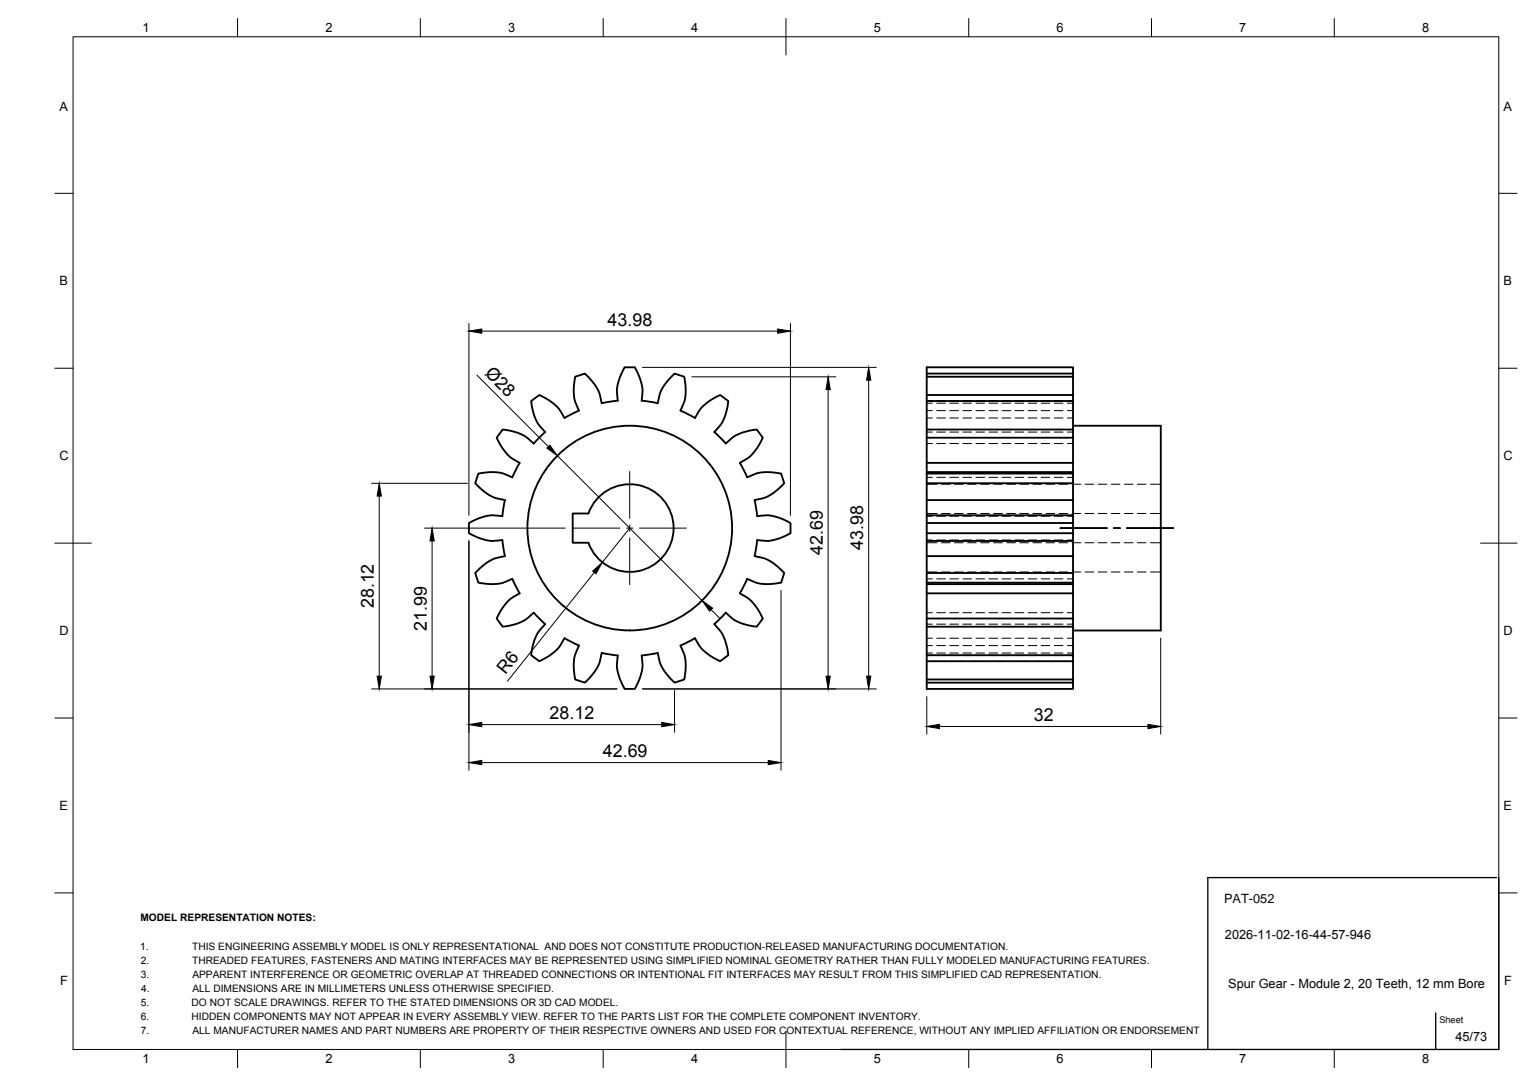
ISO-10303-21;
HEADER;
/* Generated by software containing ST-Developer
 * from STEP Tools, Inc. (www.steptools.com) 
 */

FILE_DESCRIPTION(
/* description */ ('Hand-crank gear train demonstrator'),
/* implementation_level */ '2;1');

FILE_NAME(
/* name */ 'Spur Gear - Module 2, 20 Teeth, 12 mm Bore.step',
/* time_stamp */ '2026-10-28T03:22:13-07:00',
/* author */ (''),
/* organization */ (''),
/* preprocessor_version */ 'ST-DEVELOPER v20.2',
/* originating_system */ 'Autodesk Translation Framework v15.17.0.0',
/* authorisation */ '');

FILE_SCHEMA (('AUTOMOTIVE_DESIGN { 1 0 10303 214 3 1 1 }'));
ENDSEC;

DATA;
#10=MECHANICAL_DESIGN_GEOMETRIC_PRESENTATION_REPRESENTATION('',(#1253),#62758);
#11=(
BOUNDED_SURFACE()
B_SPLINE_SURFACE(5,1,((#29730,#29731),(#29732,#29733),(#29734,#29735),(#29736,
#29737),(#29738,#29739),(#29740,#29741),(#29742,#29743),(#29744,#29745),
(#29746,#29747),(#29748,#29749),(#29750,#29751),(#29752,#29753),(#29754,
#29755),(#29756,#29757),(#29758,#29759),(#29760,#29761),(#29762,#29763),
(#29764,#29765),(#29766,#29767),(#29768,#29769),(#29770,#29771),(#29772,
#29773),(#29774,#29775),(#29776,#29777),(#29778,#29779),(#29780,#29781),
(#29782,#29783),(#29784,#29785),(#29786,#29787),(#29788,#29789),(#29790,
#29791),(#29792,#29793),(#29794,#29795),(#29796,#29797),(#29798,#29799),
(#29800,#29801),(#29802,#29803),(#29804,#29805),(#29806,#29807),(#29808,
#29809),(#29810,#29811),(#29812,#29813),(#29814,#29815),(#29816,#29817),
(#29818,#29819),(#29820,#29821),(#29822,#29823),(#29824,#29825),(#29826,
#29827),(#29828,#29829),(#29830,#29831),(#29832,#29833),(#29834,#29835),
(#29836,#29837),(#29838,#29839),(#29840,#29841),(#29842,#29843),(#29844,
#29845),(#29846,#29847),(#29848,#29849),(#29850,#29851),(#29852,#29853),
(#29854,#29855),(#29856,#29857),(#29858,#29859),(#29860,#29861),(#29862,
#29863),(#29864,#29865),(#29866,#29867),(#29868,#29869)),.UNSPECIFIED.,
 .F.,.F.,.F.)
B_SPLINE_SURFACE_WITH_KNOTS((6,1,1,1,1,1,1,1,1,1,1,1,1,1,1,1,1,1,1,1,1,
1,1,1,1,1,1,1,1,1,1,1,1,1,1,1,1,1,1,1,1,1,1,1,1,1,1,1,1,1,1,1,1,1,1,1,1,
1,1,1,1,1,1,1,1,6),(2,2),(-1.,-0.984615384615383,-0.969230769230768,-0.953846153846152,
-0.938461538461537,-0.923076923076922,-0.907692307692306,-0.892307692307691,
-0.876923076923076,-0.86153846153846,-0.846153846153845,-0.83076923076923,
-0.815384615384614,-0.799999999999999,-0.784615384615384,-0.769230769230768,
-0.753846153846153,-0.738461538461538,-0.723076923076922,-0.707692307692307,
-0.692307692307692,-0.676923076923076,-0.661538461538461,-0.646153846153846,
-0.63076923076923,-0.615384615384615,-0.6,-0.584615384615384,-0.569230769230769,
-0.553846153846154,-0.538461538461538,-0.523076923076923,-0.507692307692308,
-0.492307692307692,-0.476923076923077,-0.461538461538462,-0.446153846153846,
-0.430769230769231,-0.415384615384615,-0.4,-0.384615384615385,-0.369230769230769,
-0.353846153846154,-0.338461538461538,-0.323076923076923,-0.307692307692308,
-0.292307692307692,-0.276923076923077,-0.261538461538462,-0.246153846153846,
-0.230769230769231,-0.215384615384615,-0.2,-0.184615384615385,-0.169230769230769,
-0.153846153846154,-0.138461538461538,-0.123076923076923,-0.107692307692308,
-0.0923076923076923,-0.0769230769230769,-0.0615384615384615,-0.0461538461538462,
-0.0307692307692308,-0.0153846153846154,0.),(-1.,1.),.UNSPECIFIED.)
GEOMETRIC_REPRESENTATION_ITEM()
RATIONAL_B_SPLINE_SURFACE(((1.,1.),(1.,1.),(1.,1.),(1.,1.),(1.,1.),(1.,
1.),(1.,1.),(1.,1.),(1.,1.),(1.,1.),(1.,1.),(1.,1.),(1.,1.),(1.,1.),(1.,
1.),(1.,1.),(1.,1.),(1.,1.),(1.,1.),(1.,1.),(1.,1.),(1.,1.),(1.,1.),(1.,
1.),(1.,1.),(1.,1.),(1.,1.),(1.,1.),(1.,1.),(1.,1.),(1.,1.),(1.,1.),(1.,
1.),(1.,1.),(1.,1.),(1.,1.),(1.,1.),(1.,1.),(1.,1.),(1.,1.),(1.,1.),(1.,
1.),(1.,1.),(1.,1.),(1.,1.),(1.,1.),(1.,1.),(1.,1.),(1.,1.),(1.,1.),(1.,
1.),(1.,1.),(1.,1.),(1.,1.),(1.,1.),(1.,1.),(1.,1.),(1.,1.),(1.,1.),(1.,
1.),(1.,1.),(1.,1.),(1.,1.),(1.,1.),(1.,1.),(1.,1.),(1.,1.),(1.,1.),(1.,
1.),(1.,1.)))
REPRESENTATION_ITEM('')
SURFACE()
);
#12=(
BOUNDED_SURFACE()
B_SPLINE_SURFACE(5,1,((#29948,#29949),(#29950,#29951),(#29952,#29953),(#29954,
#29955),(#29956,#29957),(#29958,#29959),(#29960,#29961),(#29962,#29963),
(#29964,#29965),(#29966,#29967),(#29968,#29969),(#29970,#29971),(#29972,
#29973),(#29974,#29975),(#29976,#29977),(#29978,#29979),(#29980,#29981),
(#29982,#29983),(#29984,#29985),(#29986,#29987),(#29988,#29989),(#29990,
#29991),(#29992,#29993),(#29994,#29995),(#29996,#29997),(#29998,#29999),
(#30000,#30001),(#30002,#30003),(#30004,#30005),(#30006,#30007),(#30008,
#30009),(#30010,#30011),(#30012,#30013),(#30014,#30015),(#30016,#30017),
(#30018,#30019),(#30020,#30021),(#30022,#30023),(#30024,#30025),(#30026,
#30027),(#30028,#30029),(#30030,#30031),(#30032,#30033),(#30034,#30035),
(#30036,#30037),(#30038,#30039),(#30040,#30041),(#30042,#30043),(#30044,
#30045),(#30046,#30047),(#30048,#30049),(#30050,#30051),(#30052,#30053),
(#30054,#30055),(#30056,#30057),(#30058,#30059),(#30060,#30061),(#30062,
#30063),(#30064,#30065),(#30066,#30067),(#30068,#30069),(#30070,#30071),
(#30072,#30073),(#30074,#30075),(#30076,#30077),(#30078,#30079),(#30080,
#30081),(#30082,#30083),(#30084,#30085),(#30086,#30087)),.UNSPECIFIED.,
 .F.,.F.,.F.)
B_SPLINE_SURFACE_WITH_KNOTS((6,1,1,1,1,1,1,1,1,1,1,1,1,1,1,1,1,1,1,1,1,
1,1,1,1,1,1,1,1,1,1,1,1,1,1,1,1,1,1,1,1,1,1,1,1,1,1,1,1,1,1,1,1,1,1,1,1,
1,1,1,1,1,1,1,1,6),(2,2),(-1.,-0.984615384615383,-0.969230769230768,-0.953846153846152,
-0.938461538461537,-0.923076923076922,-0.907692307692306,-0.892307692307691,
-0.876923076923076,-0.86153846153846,-0.846153846153845,-0.83076923076923,
-0.815384615384614,-0.799999999999999,-0.784615384615384,-0.769230769230768,
-0.753846153846153,-0.738461538461538,-0.723076923076922,-0.707692307692307,
-0.692307692307692,-0.676923076923076,-0.661538461538461,-0.646153846153846,
-0.63076923076923,-0.615384615384615,-0.6,-0.584615384615384,-0.569230769230769,
-0.553846153846154,-0.538461538461538,-0.523076923076923,-0.507692307692308,
-0.492307692307692,-0.476923076923077,-0.461538461538462,-0.446153846153846,
-0.430769230769231,-0.415384615384615,-0.4,-0.384615384615385,-0.369230769230769,
-0.353846153846154,-0.338461538461538,-0.323076923076923,-0.307692307692308,
-0.292307692307692,-0.276923076923077,-0.261538461538462,-0.246153846153846,
-0.230769230769231,-0.215384615384615,-0.2,-0.184615384615385,-0.169230769230769,
-0.153846153846154,-0.138461538461538,-0.123076923076923,-0.107692307692308,
-0.0923076923076923,-0.0769230769230769,-0.0615384615384615,-0.0461538461538462,
-0.0307692307692308,-0.0153846153846154,0.),(-1.,1.),.UNSPECIFIED.)
GEOMETRIC_REPRESENTATION_ITEM()
RATIONAL_B_SPLINE_SURFACE(((1.,1.),(1.,1.),(1.,1.),(1.,1.),(1.,1.),(1.,
1.),(1.,1.),(1.,1.),(1.,1.),(1.,1.),(1.,1.),(1.,1.),(1.,1.),(1.,1.),(1.,
1.),(1.,1.),(1.,1.),(1.,1.),(1.,1.),(1.,1.),(1.,1.),(1.,1.),(1.,1.),(1.,
1.),(1.,1.),(1.,1.),(1.,1.),(1.,1.),(1.,1.),(1.,1.),(1.,1.),(1.,1.),(1.,
1.),(1.,1.),(1.,1.),(1.,1.),(1.,1.),(1.,1.),(1.,1.),(1.,1.),(1.,1.),(1.,
1.),(1.,1.),(1.,1.),(1.,1.),(1.,1.),(1.,1.),(1.,1.),(1.,1.),(1.,1.),(1.,
1.),(1.,1.),(1.,1.),(1.,1.),(1.,1.),(1.,1.),(1.,1.),(1.,1.),(1.,1.),(1.,
1.),(1.,1.),(1.,1.),(1.,1.),(1.,1.),(1.,1.),(1.,1.),(1.,1.),(1.,1.),(1.,
1.),(1.,1.)))
REPRESENTATION_ITEM('')
SURFACE()
);
#13=(
BOUNDED_SURFACE()
B_SPLINE_SURFACE(5,1,((#30164,#30165),(#30166,#30167),(#30168,#30169),(#30170,
#30171),(#30172,#30173),(#30174,#30175),(#30176,#30177),(#30178,#30179),
(#30180,#30181),(#30182,#30183),(#30184,#30185),(#30186,#30187),(#30188,
#30189),(#30190,#30191),(#30192,#30193),(#30194,#30195),(#30196,#30197),
(#30198,#30199),(#30200,#30201),(#30202,#30203),(#30204,#30205),(#30206,
#30207),(#30208,#30209),(#30210,#30211),(#30212,#30213),(#30214,#30215),
(#30216,#30217),(#30218,#30219),(#30220,#30221),(#30222,#30223),(#30224,
#30225),(#30226,#30227),(#30228,#30229),(#30230,#30231),(#30232,#30233),
(#30234,#30235),(#30236,#30237),(#30238,#30239),(#30240,#30241),(#30242,
#30243),(#30244,#30245),(#30246,#30247),(#30248,#30249),(#30250,#30251),
(#30252,#30253),(#30254,#30255),(#30256,#30257),(#30258,#30259),(#30260,
#30261),(#30262,#30263),(#30264,#30265),(#30266,#30267),(#30268,#30269),
(#30270,#30271),(#30272,#30273),(#30274,#30275),(#30276,#30277),(#30278,
#30279),(#30280,#30281),(#30282,#30283),(#30284,#30285),(#30286,#30287),
(#30288,#30289),(#30290,#30291),(#30292,#30293),(#30294,#30295),(#30296,
#30297),(#30298,#30299),(#30300,#30301),(#30302,#30303)),.UNSPECIFIED.,
 .F.,.F.,.F.)
B_SPLINE_SURFACE_WITH_KNOTS((6,1,1,1,1,1,1,1,1,1,1,1,1,1,1,1,1,1,1,1,1,
1,1,1,1,1,1,1,1,1,1,1,1,1,1,1,1,1,1,1,1,1,1,1,1,1,1,1,1,1,1,1,1,1,1,1,1,
1,1,1,1,1,1,1,1,6),(2,2),(-1.,-0.984615384615383,-0.969230769230768,-0.953846153846152,
-0.938461538461537,-0.923076923076922,-0.907692307692306,-0.892307692307691,
-0.876923076923076,-0.86153846153846,-0.846153846153845,-0.83076923076923,
-0.815384615384614,-0.799999999999999,-0.784615384615384,-0.769230769230768,
-0.753846153846153,-0.738461538461538,-0.723076923076922,-0.707692307692307,
-0.692307692307692,-0.676923076923076,-0.661538461538461,-0.646153846153846,
-0.63076923076923,-0.615384615384615,-0.6,-0.584615384615384,-0.569230769230769,
-0.553846153846154,-0.538461538461538,-0.523076923076923,-0.507692307692308,
-0.492307692307692,-0.476923076923077,-0.461538461538462,-0.446153846153846,
-0.430769230769231,-0.415384615384615,-0.4,-0.384615384615385,-0.369230769230769,
-0.353846153846154,-0.338461538461538,-0.323076923076923,-0.307692307692308,
-0.292307692307692,-0.276923076923077,-0.261538461538462,-0.246153846153846,
-0.230769230769231,-0.215384615384615,-0.2,-0.184615384615385,-0.169230769230769,
-0.153846153846154,-0.138461538461538,-0.123076923076923,-0.107692307692308,
-0.0923076923076923,-0.0769230769230769,-0.0615384615384615,-0.0461538461538462,
-0.0307692307692308,-0.0153846153846154,0.),(-1.,1.),.UNSPECIFIED.)
GEOMETRIC_REPRESENTATION_ITEM()
RATIONAL_B_SPLINE_SURFACE(((1.,1.),(1.,1.),(1.,1.),(1.,1.),(1.,1.),(1.,
1.),(1.,1.),(1.,1.),(1.,1.),(1.,1.),(1.,1.),(1.,1.),(1.,1.),(1.,1.),(1.,
1.),(1.,1.),(1.,1.),(1.,1.),(1.,1.),(1.,1.),(1.,1.),(1.,1.),(1.,1.),(1.,
1.),(1.,1.),(1.,1.),(1.,1.),(1.,1.),(1.,1.),(1.,1.),(1.,1.),(1.,1.),(1.,
1.),(1.,1.),(1.,1.),(1.,1.),(1.,1.),(1.,1.),(1.,1.),(1.,1.),(1.,1.),(1.,
1.),(1.,1.),(1.,1.),(1.,1.),(1.,1.),(1.,1.),(1.,1.),(1.,1.),(1.,1.),(1.,
1.),(1.,1.),(1.,1.),(1.,1.),(1.,1.),(1.,1.),(1.,1.),(1.,1.),(1.,1.),(1.,
1.),(1.,1.),(1.,1.),(1.,1.),(1.,1.),(1.,1.),(1.,1.),(1.,1.),(1.,1.),(1.,
1.),(1.,1.)))
REPRESENTATION_ITEM('')
SURFACE()
);
#14=(
BOUNDED_SURFACE()
B_SPLINE_SURFACE(5,1,((#30380,#30381),(#30382,#30383),(#30384,#30385),(#30386,
#30387),(#30388,#30389),(#30390,#30391),(#30392,#30393),(#30394,#30395),
(#30396,#30397),(#30398,#30399),(#30400,#30401),(#30402,#30403),(#30404,
#30405),(#30406,#30407),(#30408,#30409),(#30410,#30411),(#30412,#30413),
(#30414,#30415),(#30416,#30417),(#30418,#30419),(#30420,#30421),(#30422,
#30423),(#30424,#30425),(#30426,#30427),(#30428,#30429),(#30430,#30431),
(#30432,#30433),(#30434,#30435),(#30436,#30437),(#30438,#30439),(#30440,
#30441),(#30442,#30443),(#30444,#30445),(#30446,#30447),(#30448,#30449),
(#30450,#30451),(#30452,#30453),(#30454,#30455),(#30456,#30457),(#30458,
#30459),(#30460,#30461),(#30462,#30463),(#30464,#30465),(#30466,#30467),
(#30468,#30469),(#30470,#30471),(#30472,#30473),(#30474,#30475),(#30476,
#30477),(#30478,#30479),(#30480,#30481),(#30482,#30483),(#30484,#30485),
(#30486,#30487),(#30488,#30489),(#30490,#30491),(#30492,#30493),(#30494,
#30495),(#30496,#30497),(#30498,#30499),(#30500,#30501),(#30502,#30503),
(#30504,#30505),(#30506,#30507),(#30508,#30509),(#30510,#30511),(#30512,
#30513),(#30514,#30515),(#30516,#30517),(#30518,#30519)),.UNSPECIFIED.,
 .F.,.F.,.F.)
B_SPLINE_SURFACE_WITH_KNOTS((6,1,1,1,1,1,1,1,1,1,1,1,1,1,1,1,1,1,1,1,1,
1,1,1,1,1,1,1,1,1,1,1,1,1,1,1,1,1,1,1,1,1,1,1,1,1,1,1,1,1,1,1,1,1,1,1,1,
1,1,1,1,1,1,1,1,6),(2,2),(-1.,-0.984615384615383,-0.969230769230768,-0.953846153846152,
-0.938461538461537,-0.923076923076922,-0.907692307692306,-0.892307692307691,
-0.876923076923076,-0.86153846153846,-0.846153846153845,-0.83076923076923,
-0.815384615384614,-0.799999999999999,-0.784615384615384,-0.769230769230768,
-0.753846153846153,-0.738461538461538,-0.723076923076922,-0.707692307692307,
-0.692307692307692,-0.676923076923076,-0.661538461538461,-0.646153846153846,
-0.63076923076923,-0.615384615384615,-0.6,-0.584615384615384,-0.569230769230769,
-0.553846153846154,-0.538461538461538,-0.523076923076923,-0.507692307692308,
-0.492307692307692,-0.476923076923077,-0.461538461538462,-0.446153846153846,
-0.430769230769231,-0.415384615384615,-0.4,-0.384615384615385,-0.369230769230769,
-0.353846153846154,-0.338461538461538,-0.323076923076923,-0.307692307692308,
-0.292307692307692,-0.276923076923077,-0.261538461538462,-0.246153846153846,
-0.230769230769231,-0.215384615384615,-0.2,-0.184615384615385,-0.169230769230769,
-0.153846153846154,-0.138461538461538,-0.123076923076923,-0.107692307692308,
-0.0923076923076923,-0.0769230769230769,-0.0615384615384615,-0.0461538461538462,
-0.0307692307692308,-0.0153846153846154,0.),(-1.,1.),.UNSPECIFIED.)
GEOMETRIC_REPRESENTATION_ITEM()
RATIONAL_B_SPLINE_SURFACE(((1.,1.),(1.,1.),(1.,1.),(1.,1.),(1.,1.),(1.,
1.),(1.,1.),(1.,1.),(1.,1.),(1.,1.),(1.,1.),(1.,1.),(1.,1.),(1.,1.),(1.,
1.),(1.,1.),(1.,1.),(1.,1.),(1.,1.),(1.,1.),(1.,1.),(1.,1.),(1.,1.),(1.,
1.),(1.,1.),(1.,1.),(1.,1.),(1.,1.),(1.,1.),(1.,1.),(1.,1.),(1.,1.),(1.,
1.),(1.,1.),(1.,1.),(1.,1.),(1.,1.),(1.,1.),(1.,1.),(1.,1.),(1.,1.),(1.,
1.),(1.,1.),(1.,1.),(1.,1.),(1.,1.),(1.,1.),(1.,1.),(1.,1.),(1.,1.),(1.,
1.),(1.,1.),(1.,1.),(1.,1.),(1.,1.),(1.,1.),(1.,1.),(1.,1.),(1.,1.),(1.,
1.),(1.,1.),(1.,1.),(1.,1.),(1.,1.),(1.,1.),(1.,1.),(1.,1.),(1.,1.),(1.,
1.),(1.,1.)))
REPRESENTATION_ITEM('')
SURFACE()
);
#15=(
BOUNDED_SURFACE()
B_SPLINE_SURFACE(5,1,((#30596,#30597),(#30598,#30599),(#30600,#30601),(#30602,
#30603),(#30604,#30605),(#30606,#30607),(#30608,#30609),(#30610,#30611),
(#30612,#30613),(#30614,#30615),(#30616,#30617),(#30618,#30619),(#30620,
#30621),(#30622,#30623),(#30624,#30625),(#30626,#30627),(#30628,#30629),
(#30630,#30631),(#30632,#30633),(#30634,#30635),(#30636,#30637),(#30638,
#30639),(#30640,#30641),(#30642,#30643),(#30644,#30645),(#30646,#30647),
(#30648,#30649),(#30650,#30651),(#30652,#30653),(#30654,#30655),(#30656,
#30657),(#30658,#30659),(#30660,#30661),(#30662,#30663),(#30664,#30665),
(#30666,#30667),(#30668,#30669),(#30670,#30671),(#30672,#30673),(#30674,
#30675),(#30676,#30677),(#30678,#30679),(#30680,#30681),(#30682,#30683),
(#30684,#30685),(#30686,#30687),(#30688,#30689),(#30690,#30691),(#30692,
#30693),(#30694,#30695),(#30696,#30697),(#30698,#30699),(#30700,#30701),
(#30702,#30703),(#30704,#30705),(#30706,#30707),(#30708,#30709),(#30710,
#30711),(#30712,#30713),(#30714,#30715),(#30716,#30717),(#30718,#30719),
(#30720,#30721),(#30722,#30723),(#30724,#30725),(#30726,#30727),(#30728,
#30729),(#30730,#30731),(#30732,#30733),(#30734,#30735)),.UNSPECIFIED.,
 .F.,.F.,.F.)
B_SPLINE_SURFACE_WITH_KNOTS((6,1,1,1,1,1,1,1,1,1,1,1,1,1,1,1,1,1,1,1,1,
1,1,1,1,1,1,1,1,1,1,1,1,1,1,1,1,1,1,1,1,1,1,1,1,1,1,1,1,1,1,1,1,1,1,1,1,
1,1,1,1,1,1,1,1,6),(2,2),(-1.,-0.984615384615383,-0.969230769230768,-0.953846153846152,
-0.938461538461537,-0.923076923076922,-0.907692307692306,-0.892307692307691,
-0.876923076923076,-0.86153846153846,-0.846153846153845,-0.83076923076923,
-0.815384615384614,-0.799999999999999,-0.784615384615384,-0.769230769230768,
-0.753846153846153,-0.738461538461538,-0.723076923076922,-0.707692307692307,
-0.692307692307692,-0.676923076923076,-0.661538461538461,-0.646153846153846,
-0.63076923076923,-0.615384615384615,-0.6,-0.584615384615384,-0.569230769230769,
-0.553846153846154,-0.538461538461538,-0.523076923076923,-0.507692307692308,
-0.492307692307692,-0.476923076923077,-0.461538461538462,-0.446153846153846,
-0.430769230769231,-0.415384615384615,-0.4,-0.384615384615385,-0.369230769230769,
-0.353846153846154,-0.338461538461538,-0.323076923076923,-0.307692307692308,
-0.292307692307692,-0.276923076923077,-0.261538461538462,-0.246153846153846,
-0.230769230769231,-0.215384615384615,-0.2,-0.184615384615385,-0.169230769230769,
-0.153846153846154,-0.138461538461538,-0.123076923076923,-0.107692307692308,
-0.0923076923076923,-0.0769230769230769,-0.0615384615384615,-0.0461538461538462,
-0.0307692307692308,-0.0153846153846154,0.),(-1.,1.),.UNSPECIFIED.)
GEOMETRIC_REPRESENTATION_ITEM()
RATIONAL_B_SPLINE_SURFACE(((1.,1.),(1.,1.),(1.,1.),(1.,1.),(1.,1.),(1.,
1.),(1.,1.),(1.,1.),(1.,1.),(1.,1.),(1.,1.),(1.,1.),(1.,1.),(1.,1.),(1.,
1.),(1.,1.),(1.,1.),(1.,1.),(1.,1.),(1.,1.),(1.,1.),(1.,1.),(1.,1.),(1.,
1.),(1.,1.),(1.,1.),(1.,1.),(1.,1.),(1.,1.),(1.,1.),(1.,1.),(1.,1.),(1.,
1.),(1.,1.),(1.,1.),(1.,1.),(1.,1.),(1.,1.),(1.,1.),(1.,1.),(1.,1.),(1.,
1.),(1.,1.),(1.,1.),(1.,1.),(1.,1.),(1.,1.),(1.,1.),(1.,1.),(1.,1.),(1.,
1.),(1.,1.),(1.,1.),(1.,1.),(1.,1.),(1.,1.),(1.,1.),(1.,1.),(1.,1.),(1.,
1.),(1.,1.),(1.,1.),(1.,1.),(1.,1.),(1.,1.),(1.,1.),(1.,1.),(1.,1.),(1.,
1.),(1.,1.)))
REPRESENTATION_ITEM('')
SURFACE()
);
#16=(
BOUNDED_SURFACE()
B_SPLINE_SURFACE(5,1,((#30812,#30813),(#30814,#30815),(#30816,#30817),(#30818,
#30819),(#30820,#30821),(#30822,#30823),(#30824,#30825),(#30826,#30827),
(#30828,#30829),(#30830,#30831),(#30832,#30833),(#30834,#30835),(#30836,
#30837),(#30838,#30839),(#30840,#30841),(#30842,#30843),(#30844,#30845),
(#30846,#30847),(#30848,#30849),(#30850,#30851),(#30852,#30853),(#30854,
#30855),(#30856,#30857),(#30858,#30859),(#30860,#30861),(#30862,#30863),
(#30864,#30865),(#30866,#30867),(#30868,#30869),(#30870,#30871),(#30872,
#30873),(#30874,#30875),(#30876,#30877),(#30878,#30879),(#30880,#30881),
(#30882,#30883),(#30884,#30885),(#30886,#30887),(#30888,#30889),(#30890,
#30891),(#30892,#30893),(#30894,#30895),(#30896,#30897),(#30898,#30899),
(#30900,#30901),(#30902,#30903),(#30904,#30905),(#30906,#30907),(#30908,
#30909),(#30910,#30911),(#30912,#30913),(#30914,#30915),(#30916,#30917),
(#30918,#30919),(#30920,#30921),(#30922,#30923),(#30924,#30925),(#30926,
#30927),(#30928,#30929),(#30930,#30931),(#30932,#30933),(#30934,#30935),
(#30936,#30937),(#30938,#30939),(#30940,#30941),(#30942,#30943),(#30944,
#30945),(#30946,#30947),(#30948,#30949),(#30950,#30951)),.UNSPECIFIED.,
 .F.,.F.,.F.)
B_SPLINE_SURFACE_WITH_KNOTS((6,1,1,1,1,1,1,1,1,1,1,1,1,1,1,1,1,1,1,1,1,
1,1,1,1,1,1,1,1,1,1,1,1,1,1,1,1,1,1,1,1,1,1,1,1,1,1,1,1,1,1,1,1,1,1,1,1,
1,1,1,1,1,1,1,1,6),(2,2),(-1.,-0.984615384615383,-0.969230769230768,-0.953846153846152,
-0.938461538461537,-0.923076923076922,-0.907692307692306,-0.892307692307691,
-0.876923076923076,-0.86153846153846,-0.846153846153845,-0.83076923076923,
-0.815384615384614,-0.799999999999999,-0.784615384615384,-0.769230769230768,
-0.753846153846153,-0.738461538461538,-0.723076923076922,-0.707692307692307,
-0.692307692307692,-0.676923076923076,-0.661538461538461,-0.646153846153846,
-0.63076923076923,-0.615384615384615,-0.6,-0.584615384615384,-0.569230769230769,
-0.553846153846154,-0.538461538461538,-0.523076923076923,-0.507692307692308,
-0.492307692307692,-0.476923076923077,-0.461538461538462,-0.446153846153846,
-0.430769230769231,-0.415384615384615,-0.4,-0.384615384615385,-0.369230769230769,
-0.353846153846154,-0.338461538461538,-0.323076923076923,-0.307692307692308,
-0.292307692307692,-0.276923076923077,-0.261538461538462,-0.246153846153846,
-0.230769230769231,-0.215384615384615,-0.2,-0.184615384615385,-0.169230769230769,
-0.153846153846154,-0.138461538461538,-0.123076923076923,-0.107692307692308,
-0.0923076923076923,-0.0769230769230769,-0.0615384615384615,-0.0461538461538462,
-0.0307692307692308,-0.0153846153846154,0.),(-1.,1.),.UNSPECIFIED.)
GEOMETRIC_REPRESENTATION_ITEM()
RATIONAL_B_SPLINE_SURFACE(((1.,1.),(1.,1.),(1.,1.),(1.,1.),(1.,1.),(1.,
1.),(1.,1.),(1.,1.),(1.,1.),(1.,1.),(1.,1.),(1.,1.),(1.,1.),(1.,1.),(1.,
1.),(1.,1.),(1.,1.),(1.,1.),(1.,1.),(1.,1.),(1.,1.),(1.,1.),(1.,1.),(1.,
1.),(1.,1.),(1.,1.),(1.,1.),(1.,1.),(1.,1.),(1.,1.),(1.,1.),(1.,1.),(1.,
1.),(1.,1.),(1.,1.),(1.,1.),(1.,1.),(1.,1.),(1.,1.),(1.,1.),(1.,1.),(1.,
1.),(1.,1.),(1.,1.),(1.,1.),(1.,1.),(1.,1.),(1.,1.),(1.,1.),(1.,1.),(1.,
1.),(1.,1.),(1.,1.),(1.,1.),(1.,1.),(1.,1.),(1.,1.),(1.,1.),(1.,1.),(1.,
1.),(1.,1.),(1.,1.),(1.,1.),(1.,1.),(1.,1.),(1.,1.),(1.,1.),(1.,1.),(1.,
1.),(1.,1.)))
REPRESENTATION_ITEM('')
SURFACE()
);
#17=(
BOUNDED_SURFACE()
B_SPLINE_SURFACE(5,1,((#31028,#31029),(#31030,#31031),(#31032,#31033),(#31034,
#31035),(#31036,#31037),(#31038,#31039),(#31040,#31041),(#31042,#31043),
(#31044,#31045),(#31046,#31047),(#31048,#31049),(#31050,#31051),(#31052,
#31053),(#31054,#31055),(#31056,#31057),(#31058,#31059),(#31060,#31061),
(#31062,#31063),(#31064,#31065),(#31066,#31067),(#31068,#31069),(#31070,
#31071),(#31072,#31073),(#31074,#31075),(#31076,#31077),(#31078,#31079),
(#31080,#31081),(#31082,#31083),(#31084,#31085),(#31086,#31087),(#31088,
#31089),(#31090,#31091),(#31092,#31093),(#31094,#31095),(#31096,#31097),
(#31098,#31099),(#31100,#31101),(#31102,#31103),(#31104,#31105),(#31106,
#31107),(#31108,#31109),(#31110,#31111),(#31112,#31113),(#31114,#31115),
(#31116,#31117),(#31118,#31119),(#31120,#31121),(#31122,#31123),(#31124,
#31125),(#31126,#31127),(#31128,#31129),(#31130,#31131),(#31132,#31133),
(#31134,#31135),(#31136,#31137),(#31138,#31139),(#31140,#31141),(#31142,
#31143),(#31144,#31145),(#31146,#31147),(#31148,#31149),(#31150,#31151),
(#31152,#31153),(#31154,#31155),(#31156,#31157),(#31158,#31159),(#31160,
#31161),(#31162,#31163),(#31164,#31165),(#31166,#31167)),.UNSPECIFIED.,
 .F.,.F.,.F.)
B_SPLINE_SURFACE_WITH_KNOTS((6,1,1,1,1,1,1,1,1,1,1,1,1,1,1,1,1,1,1,1,1,
1,1,1,1,1,1,1,1,1,1,1,1,1,1,1,1,1,1,1,1,1,1,1,1,1,1,1,1,1,1,1,1,1,1,1,1,
1,1,1,1,1,1,1,1,6),(2,2),(-1.,-0.984615384615383,-0.969230769230768,-0.953846153846152,
-0.938461538461537,-0.923076923076922,-0.907692307692306,-0.892307692307691,
-0.876923076923076,-0.86153846153846,-0.846153846153845,-0.83076923076923,
-0.815384615384614,-0.799999999999999,-0.784615384615384,-0.769230769230768,
-0.753846153846153,-0.738461538461538,-0.723076923076922,-0.707692307692307,
-0.692307692307692,-0.676923076923076,-0.661538461538461,-0.646153846153846,
-0.63076923076923,-0.615384615384615,-0.6,-0.584615384615384,-0.569230769230769,
-0.553846153846154,-0.538461538461538,-0.523076923076923,-0.507692307692308,
-0.492307692307692,-0.476923076923077,-0.461538461538462,-0.446153846153846,
-0.430769230769231,-0.415384615384615,-0.4,-0.384615384615385,-0.369230769230769,
-0.353846153846154,-0.338461538461538,-0.323076923076923,-0.307692307692308,
-0.292307692307692,-0.276923076923077,-0.261538461538462,-0.246153846153846,
-0.230769230769231,-0.215384615384615,-0.2,-0.184615384615385,-0.169230769230769,
-0.153846153846154,-0.138461538461538,-0.123076923076923,-0.107692307692308,
-0.0923076923076923,-0.0769230769230769,-0.0615384615384615,-0.0461538461538462,
-0.0307692307692308,-0.0153846153846154,0.),(-1.,1.),.UNSPECIFIED.)
GEOMETRIC_REPRESENTATION_ITEM()
RATIONAL_B_SPLINE_SURFACE(((1.,1.),(1.,1.),(1.,1.),(1.,1.),(1.,1.),(1.,
1.),(1.,1.),(1.,1.),(1.,1.),(1.,1.),(1.,1.),(1.,1.),(1.,1.),(1.,1.),(1.,
1.),(1.,1.),(1.,1.),(1.,1.),(1.,1.),(1.,1.),(1.,1.),(1.,1.),(1.,1.),(1.,
1.),(1.,1.),(1.,1.),(1.,1.),(1.,1.),(1.,1.),(1.,1.),(1.,1.),(1.,1.),(1.,
1.),(1.,1.),(1.,1.),(1.,1.),(1.,1.),(1.,1.),(1.,1.),(1.,1.),(1.,1.),(1.,
1.),(1.,1.),(1.,1.),(1.,1.),(1.,1.),(1.,1.),(1.,1.),(1.,1.),(1.,1.),(1.,
1.),(1.,1.),(1.,1.),(1.,1.),(1.,1.),(1.,1.),(1.,1.),(1.,1.),(1.,1.),(1.,
1.),(1.,1.),(1.,1.),(1.,1.),(1.,1.),(1.,1.),(1.,1.),(1.,1.),(1.,1.),(1.,
1.),(1.,1.)))
REPRESENTATION_ITEM('')
SURFACE()
);
#18=(
BOUNDED_SURFACE()
B_SPLINE_SURFACE(5,1,((#31244,#31245),(#31246,#31247),(#31248,#31249),(#31250,
#31251),(#31252,#31253),(#31254,#31255),(#31256,#31257),(#31258,#31259),
(#31260,#31261),(#31262,#31263),(#31264,#31265),(#31266,#31267),(#31268,
#31269),(#31270,#31271),(#31272,#31273),(#31274,#31275),(#31276,#31277),
(#31278,#31279),(#31280,#31281),(#31282,#31283),(#31284,#31285),(#31286,
#31287),(#31288,#31289),(#31290,#31291),(#31292,#31293),(#31294,#31295),
(#31296,#31297),(#31298,#31299),(#31300,#31301),(#31302,#31303),(#31304,
#31305),(#31306,#31307),(#31308,#31309),(#31310,#31311),(#31312,#31313),
(#31314,#31315),(#31316,#31317),(#31318,#31319),(#31320,#31321),(#31322,
#31323),(#31324,#31325),(#31326,#31327),(#31328,#31329),(#31330,#31331),
(#31332,#31333),(#31334,#31335),(#31336,#31337),(#31338,#31339),(#31340,
#31341),(#31342,#31343),(#31344,#31345),(#31346,#31347),(#31348,#31349),
(#31350,#31351),(#31352,#31353),(#31354,#31355),(#31356,#31357),(#31358,
#31359),(#31360,#31361),(#31362,#31363),(#31364,#31365),(#31366,#31367),
(#31368,#31369),(#31370,#31371),(#31372,#31373),(#31374,#31375),(#31376,
#31377),(#31378,#31379),(#31380,#31381),(#31382,#31383)),.UNSPECIFIED.,
 .F.,.F.,.F.)
B_SPLINE_SURFACE_WITH_KNOTS((6,1,1,1,1,1,1,1,1,1,1,1,1,1,1,1,1,1,1,1,1,
1,1,1,1,1,1,1,1,1,1,1,1,1,1,1,1,1,1,1,1,1,1,1,1,1,1,1,1,1,1,1,1,1,1,1,1,
1,1,1,1,1,1,1,1,6),(2,2),(-1.,-0.984615384615383,-0.969230769230768,-0.953846153846152,
-0.938461538461537,-0.923076923076922,-0.907692307692306,-0.892307692307691,
-0.876923076923076,-0.86153846153846,-0.846153846153845,-0.83076923076923,
-0.815384615384614,-0.799999999999999,-0.784615384615384,-0.769230769230768,
-0.753846153846153,-0.738461538461538,-0.723076923076922,-0.707692307692307,
-0.692307692307692,-0.676923076923076,-0.661538461538461,-0.646153846153846,
-0.63076923076923,-0.615384615384615,-0.6,-0.584615384615384,-0.569230769230769,
-0.553846153846154,-0.538461538461538,-0.523076923076923,-0.507692307692308,
-0.492307692307692,-0.476923076923077,-0.461538461538462,-0.446153846153846,
-0.430769230769231,-0.415384615384615,-0.4,-0.384615384615385,-0.369230769230769,
-0.353846153846154,-0.338461538461538,-0.323076923076923,-0.307692307692308,
-0.292307692307692,-0.276923076923077,-0.261538461538462,-0.246153846153846,
-0.230769230769231,-0.215384615384615,-0.2,-0.184615384615385,-0.169230769230769,
-0.153846153846154,-0.138461538461538,-0.123076923076923,-0.107692307692308,
-0.0923076923076923,-0.0769230769230769,-0.0615384615384615,-0.0461538461538462,
-0.0307692307692308,-0.0153846153846154,0.),(-1.,1.),.UNSPECIFIED.)
GEOMETRIC_REPRESENTATION_ITEM()
RATIONAL_B_SPLINE_SURFACE(((1.,1.),(1.,1.),(1.,1.),(1.,1.),(1.,1.),(1.,
1.),(1.,1.),(1.,1.),(1.,1.),(1.,1.),(1.,1.),(1.,1.),(1.,1.),(1.,1.),(1.,
1.),(1.,1.),(1.,1.),(1.,1.),(1.,1.),(1.,1.),(1.,1.),(1.,1.),(1.,1.),(1.,
1.),(1.,1.),(1.,1.),(1.,1.),(1.,1.),(1.,1.),(1.,1.),(1.,1.),(1.,1.),(1.,
1.),(1.,1.),(1.,1.),(1.,1.),(1.,1.),(1.,1.),(1.,1.),(1.,1.),(1.,1.),(1.,
1.),(1.,1.),(1.,1.),(1.,1.),(1.,1.),(1.,1.),(1.,1.),(1.,1.),(1.,1.),(1.,
1.),(1.,1.),(1.,1.),(1.,1.),(1.,1.),(1.,1.),(1.,1.),(1.,1.),(1.,1.),(1.,
1.),(1.,1.),(1.,1.),(1.,1.),(1.,1.),(1.,1.),(1.,1.),(1.,1.),(1.,1.),(1.,
1.),(1.,1.)))
REPRESENTATION_ITEM('')
SURFACE()
);
#19=(
BOUNDED_SURFACE()
B_SPLINE_SURFACE(5,1,((#31460,#31461),(#31462,#31463),(#31464,#31465),(#31466,
#31467),(#31468,#31469),(#31470,#31471),(#31472,#31473),(#31474,#31475),
(#31476,#31477),(#31478,#31479),(#31480,#31481),(#31482,#31483),(#31484,
#31485),(#31486,#31487),(#31488,#31489),(#31490,#31491),(#31492,#31493),
(#31494,#31495),(#31496,#31497),(#31498,#31499),(#31500,#31501),(#31502,
#31503),(#31504,#31505),(#31506,#31507),(#31508,#31509),(#31510,#31511),
(#31512,#31513),(#31514,#31515),(#31516,#31517),(#31518,#31519),(#31520,
#31521),(#31522,#31523),(#31524,#31525),(#31526,#31527),(#31528,#31529),
(#31530,#31531),(#31532,#31533),(#31534,#31535),(#31536,#31537),(#31538,
#31539),(#31540,#31541),(#31542,#31543),(#31544,#31545),(#31546,#31547),
(#31548,#31549),(#31550,#31551),(#31552,#31553),(#31554,#31555),(#31556,
#31557),(#31558,#31559),(#31560,#31561),(#31562,#31563),(#31564,#31565),
(#31566,#31567),(#31568,#31569),(#31570,#31571),(#31572,#31573),(#31574,
#31575),(#31576,#31577),(#31578,#31579),(#31580,#31581),(#31582,#31583),
(#31584,#31585),(#31586,#31587),(#31588,#31589),(#31590,#31591),(#31592,
#31593),(#31594,#31595),(#31596,#31597),(#31598,#31599)),.UNSPECIFIED.,
 .F.,.F.,.F.)
B_SPLINE_SURFACE_WITH_KNOTS((6,1,1,1,1,1,1,1,1,1,1,1,1,1,1,1,1,1,1,1,1,
1,1,1,1,1,1,1,1,1,1,1,1,1,1,1,1,1,1,1,1,1,1,1,1,1,1,1,1,1,1,1,1,1,1,1,1,
1,1,1,1,1,1,1,1,6),(2,2),(-1.,-0.984615384615383,-0.969230769230768,-0.953846153846152,
-0.938461538461537,-0.923076923076922,-0.907692307692306,-0.892307692307691,
-0.876923076923076,-0.86153846153846,-0.846153846153845,-0.83076923076923,
-0.815384615384614,-0.799999999999999,-0.784615384615384,-0.769230769230768,
-0.753846153846153,-0.738461538461538,-0.723076923076922,-0.707692307692307,
-0.692307692307692,-0.676923076923076,-0.661538461538461,-0.646153846153846,
-0.63076923076923,-0.615384615384615,-0.6,-0.584615384615384,-0.569230769230769,
-0.553846153846154,-0.538461538461538,-0.523076923076923,-0.507692307692308,
-0.492307692307692,-0.476923076923077,-0.461538461538462,-0.446153846153846,
-0.430769230769231,-0.415384615384615,-0.4,-0.384615384615385,-0.369230769230769,
-0.353846153846154,-0.338461538461538,-0.323076923076923,-0.307692307692308,
-0.292307692307692,-0.276923076923077,-0.261538461538462,-0.246153846153846,
-0.230769230769231,-0.215384615384615,-0.2,-0.184615384615385,-0.169230769230769,
-0.153846153846154,-0.138461538461538,-0.123076923076923,-0.107692307692308,
-0.0923076923076923,-0.0769230769230769,-0.0615384615384615,-0.0461538461538462,
-0.0307692307692308,-0.0153846153846154,0.),(-1.,1.),.UNSPECIFIED.)
GEOMETRIC_REPRESENTATION_ITEM()
RATIONAL_B_SPLINE_SURFACE(((1.,1.),(1.,1.),(1.,1.),(1.,1.),(1.,1.),(1.,
1.),(1.,1.),(1.,1.),(1.,1.),(1.,1.),(1.,1.),(1.,1.),(1.,1.),(1.,1.),(1.,
1.),(1.,1.),(1.,1.),(1.,1.),(1.,1.),(1.,1.),(1.,1.),(1.,1.),(1.,1.),(1.,
1.),(1.,1.),(1.,1.),(1.,1.),(1.,1.),(1.,1.),(1.,1.),(1.,1.),(1.,1.),(1.,
1.),(1.,1.),(1.,1.),(1.,1.),(1.,1.),(1.,1.),(1.,1.),(1.,1.),(1.,1.),(1.,
1.),(1.,1.),(1.,1.),(1.,1.),(1.,1.),(1.,1.),(1.,1.),(1.,1.),(1.,1.),(1.,
1.),(1.,1.),(1.,1.),(1.,1.),(1.,1.),(1.,1.),(1.,1.),(1.,1.),(1.,1.),(1.,
1.),(1.,1.),(1.,1.),(1.,1.),(1.,1.),(1.,1.),(1.,1.),(1.,1.),(1.,1.),(1.,
1.),(1.,1.)))
REPRESENTATION_ITEM('')
SURFACE()
);
#20=(
BOUNDED_SURFACE()
B_SPLINE_SURFACE(5,1,((#31676,#31677),(#31678,#31679),(#31680,#31681),(#31682,
#31683),(#31684,#31685),(#31686,#31687),(#31688,#31689),(#31690,#31691),
(#31692,#31693),(#31694,#31695),(#31696,#31697),(#31698,#31699),(#31700,
#31701),(#31702,#31703),(#31704,#31705),(#31706,#31707),(#31708,#31709),
(#31710,#31711),(#31712,#31713),(#31714,#31715),(#31716,#31717),(#31718,
#31719),(#31720,#31721),(#31722,#31723),(#31724,#31725),(#31726,#31727),
(#31728,#31729),(#31730,#31731),(#31732,#31733),(#31734,#31735),(#31736,
#31737),(#31738,#31739),(#31740,#31741),(#31742,#31743),(#31744,#31745),
(#31746,#31747),(#31748,#31749),(#31750,#31751),(#31752,#31753),(#31754,
#31755),(#31756,#31757),(#31758,#31759),(#31760,#31761),(#31762,#31763),
(#31764,#31765),(#31766,#31767),(#31768,#31769),(#31770,#31771),(#31772,
#31773),(#31774,#31775),(#31776,#31777),(#31778,#31779),(#31780,#31781),
(#31782,#31783),(#31784,#31785),(#31786,#31787),(#31788,#31789),(#31790,
#31791),(#31792,#31793),(#31794,#31795),(#31796,#31797),(#31798,#31799),
(#31800,#31801),(#31802,#31803),(#31804,#31805),(#31806,#31807),(#31808,
#31809),(#31810,#31811),(#31812,#31813),(#31814,#31815)),.UNSPECIFIED.,
 .F.,.F.,.F.)
B_SPLINE_SURFACE_WITH_KNOTS((6,1,1,1,1,1,1,1,1,1,1,1,1,1,1,1,1,1,1,1,1,
1,1,1,1,1,1,1,1,1,1,1,1,1,1,1,1,1,1,1,1,1,1,1,1,1,1,1,1,1,1,1,1,1,1,1,1,
1,1,1,1,1,1,1,1,6),(2,2),(-1.,-0.984615384615383,-0.969230769230768,-0.953846153846152,
-0.938461538461537,-0.923076923076922,-0.907692307692306,-0.892307692307691,
-0.876923076923076,-0.86153846153846,-0.846153846153845,-0.83076923076923,
-0.815384615384614,-0.799999999999999,-0.784615384615384,-0.769230769230768,
-0.753846153846153,-0.738461538461538,-0.723076923076922,-0.707692307692307,
-0.692307692307692,-0.676923076923076,-0.661538461538461,-0.646153846153846,
-0.63076923076923,-0.615384615384615,-0.6,-0.584615384615384,-0.569230769230769,
-0.553846153846154,-0.538461538461538,-0.523076923076923,-0.507692307692308,
-0.492307692307692,-0.476923076923077,-0.461538461538462,-0.446153846153846,
-0.430769230769231,-0.415384615384615,-0.4,-0.384615384615385,-0.369230769230769,
-0.353846153846154,-0.338461538461538,-0.323076923076923,-0.307692307692308,
-0.292307692307692,-0.276923076923077,-0.261538461538462,-0.246153846153846,
-0.230769230769231,-0.215384615384615,-0.2,-0.184615384615385,-0.169230769230769,
-0.153846153846154,-0.138461538461538,-0.123076923076923,-0.107692307692308,
-0.0923076923076923,-0.0769230769230769,-0.0615384615384615,-0.0461538461538462,
-0.0307692307692308,-0.0153846153846154,0.),(-1.,1.),.UNSPECIFIED.)
GEOMETRIC_REPRESENTATION_ITEM()
RATIONAL_B_SPLINE_SURFACE(((1.,1.),(1.,1.),(1.,1.),(1.,1.),(1.,1.),(1.,
1.),(1.,1.),(1.,1.),(1.,1.),(1.,1.),(1.,1.),(1.,1.),(1.,1.),(1.,1.),(1.,
1.),(1.,1.),(1.,1.),(1.,1.),(1.,1.),(1.,1.),(1.,1.),(1.,1.),(1.,1.),(1.,
1.),(1.,1.),(1.,1.),(1.,1.),(1.,1.),(1.,1.),(1.,1.),(1.,1.),(1.,1.),(1.,
1.),(1.,1.),(1.,1.),(1.,1.),(1.,1.),(1.,1.),(1.,1.),(1.,1.),(1.,1.),(1.,
1.),(1.,1.),(1.,1.),(1.,1.),(1.,1.),(1.,1.),(1.,1.),(1.,1.),(1.,1.),(1.,
1.),(1.,1.),(1.,1.),(1.,1.),(1.,1.),(1.,1.),(1.,1.),(1.,1.),(1.,1.),(1.,
1.),(1.,1.),(1.,1.),(1.,1.),(1.,1.),(1.,1.),(1.,1.),(1.,1.),(1.,1.),(1.,
1.),(1.,1.)))
REPRESENTATION_ITEM('')
SURFACE()
);
#21=(
BOUNDED_SURFACE()
B_SPLINE_SURFACE(5,1,((#31892,#31893),(#31894,#31895),(#31896,#31897),(#31898,
#31899),(#31900,#31901),(#31902,#31903),(#31904,#31905),(#31906,#31907),
(#31908,#31909),(#31910,#31911),(#31912,#31913),(#31914,#31915),(#31916,
#31917),(#31918,#31919),(#31920,#31921),(#31922,#31923),(#31924,#31925),
(#31926,#31927),(#31928,#31929),(#31930,#31931),(#31932,#31933),(#31934,
#31935),(#31936,#31937),(#31938,#31939),(#31940,#31941),(#31942,#31943),
(#31944,#31945),(#31946,#31947),(#31948,#31949),(#31950,#31951),(#31952,
#31953),(#31954,#31955),(#31956,#31957),(#31958,#31959),(#31960,#31961),
(#31962,#31963),(#31964,#31965),(#31966,#31967),(#31968,#31969),(#31970,
#31971),(#31972,#31973),(#31974,#31975),(#31976,#31977),(#31978,#31979),
(#31980,#31981),(#31982,#31983),(#31984,#31985),(#31986,#31987),(#31988,
#31989),(#31990,#31991),(#31992,#31993),(#31994,#31995),(#31996,#31997),
(#31998,#31999),(#32000,#32001),(#32002,#32003),(#32004,#32005),(#32006,
#32007),(#32008,#32009),(#32010,#32011),(#32012,#32013),(#32014,#32015),
(#32016,#32017),(#32018,#32019),(#32020,#32021),(#32022,#32023),(#32024,
#32025),(#32026,#32027),(#32028,#32029),(#32030,#32031)),.UNSPECIFIED.,
 .F.,.F.,.F.)
B_SPLINE_SURFACE_WITH_KNOTS((6,1,1,1,1,1,1,1,1,1,1,1,1,1,1,1,1,1,1,1,1,
1,1,1,1,1,1,1,1,1,1,1,1,1,1,1,1,1,1,1,1,1,1,1,1,1,1,1,1,1,1,1,1,1,1,1,1,
1,1,1,1,1,1,1,1,6),(2,2),(-1.,-0.984615384615383,-0.969230769230768,-0.953846153846152,
-0.938461538461537,-0.923076923076922,-0.907692307692306,-0.892307692307691,
-0.876923076923076,-0.86153846153846,-0.846153846153845,-0.83076923076923,
-0.815384615384614,-0.799999999999999,-0.784615384615384,-0.769230769230768,
-0.753846153846153,-0.738461538461538,-0.723076923076922,-0.707692307692307,
-0.692307692307692,-0.676923076923076,-0.661538461538461,-0.646153846153846,
-0.63076923076923,-0.615384615384615,-0.6,-0.584615384615384,-0.569230769230769,
-0.553846153846154,-0.538461538461538,-0.523076923076923,-0.507692307692308,
-0.492307692307692,-0.476923076923077,-0.461538461538462,-0.446153846153846,
-0.430769230769231,-0.415384615384615,-0.4,-0.384615384615385,-0.369230769230769,
-0.353846153846154,-0.338461538461538,-0.323076923076923,-0.307692307692308,
-0.292307692307692,-0.276923076923077,-0.261538461538462,-0.246153846153846,
-0.230769230769231,-0.215384615384615,-0.2,-0.184615384615385,-0.169230769230769,
-0.153846153846154,-0.138461538461538,-0.123076923076923,-0.107692307692308,
-0.0923076923076923,-0.0769230769230769,-0.0615384615384615,-0.0461538461538462,
-0.0307692307692308,-0.0153846153846154,0.),(-1.,1.),.UNSPECIFIED.)
GEOMETRIC_REPRESENTATION_ITEM()
RATIONAL_B_SPLINE_SURFACE(((1.,1.),(1.,1.),(1.,1.),(1.,1.),(1.,1.),(1.,
1.),(1.,1.),(1.,1.),(1.,1.),(1.,1.),(1.,1.),(1.,1.),(1.,1.),(1.,1.),(1.,
1.),(1.,1.),(1.,1.),(1.,1.),(1.,1.),(1.,1.),(1.,1.),(1.,1.),(1.,1.),(1.,
1.),(1.,1.),(1.,1.),(1.,1.),(1.,1.),(1.,1.),(1.,1.),(1.,1.),(1.,1.),(1.,
1.),(1.,1.),(1.,1.),(1.,1.),(1.,1.),(1.,1.),(1.,1.),(1.,1.),(1.,1.),(1.,
1.),(1.,1.),(1.,1.),(1.,1.),(1.,1.),(1.,1.),(1.,1.),(1.,1.),(1.,1.),(1.,
1.),(1.,1.),(1.,1.),(1.,1.),(1.,1.),(1.,1.),(1.,1.),(1.,1.),(1.,1.),(1.,
1.),(1.,1.),(1.,1.),(1.,1.),(1.,1.),(1.,1.),(1.,1.),(1.,1.),(1.,1.),(1.,
1.),(1.,1.)))
REPRESENTATION_ITEM('')
SURFACE()
);
#22=(
BOUNDED_SURFACE()
B_SPLINE_SURFACE(5,1,((#32108,#32109),(#32110,#32111),(#32112,#32113),(#32114,
#32115),(#32116,#32117),(#32118,#32119),(#32120,#32121),(#32122,#32123),
(#32124,#32125),(#32126,#32127),(#32128,#32129),(#32130,#32131),(#32132,
#32133),(#32134,#32135),(#32136,#32137),(#32138,#32139),(#32140,#32141),
(#32142,#32143),(#32144,#32145),(#32146,#32147),(#32148,#32149),(#32150,
#32151),(#32152,#32153),(#32154,#32155),(#32156,#32157),(#32158,#32159),
(#32160,#32161),(#32162,#32163),(#32164,#32165),(#32166,#32167),(#32168,
#32169),(#32170,#32171),(#32172,#32173),(#32174,#32175),(#32176,#32177),
(#32178,#32179),(#32180,#32181),(#32182,#32183),(#32184,#32185),(#32186,
#32187),(#32188,#32189),(#32190,#32191),(#32192,#32193),(#32194,#32195),
(#32196,#32197),(#32198,#32199),(#32200,#32201),(#32202,#32203),(#32204,
#32205),(#32206,#32207),(#32208,#32209),(#32210,#32211),(#32212,#32213),
(#32214,#32215),(#32216,#32217),(#32218,#32219),(#32220,#32221),(#32222,
#32223),(#32224,#32225),(#32226,#32227),(#32228,#32229),(#32230,#32231),
(#32232,#32233),(#32234,#32235),(#32236,#32237),(#32238,#32239),(#32240,
#32241),(#32242,#32243),(#32244,#32245),(#32246,#32247)),.UNSPECIFIED.,
 .F.,.F.,.F.)
B_SPLINE_SURFACE_WITH_KNOTS((6,1,1,1,1,1,1,1,1,1,1,1,1,1,1,1,1,1,1,1,1,
1,1,1,1,1,1,1,1,1,1,1,1,1,1,1,1,1,1,1,1,1,1,1,1,1,1,1,1,1,1,1,1,1,1,1,1,
1,1,1,1,1,1,1,1,6),(2,2),(-1.,-0.984615384615383,-0.969230769230768,-0.953846153846152,
-0.938461538461537,-0.923076923076922,-0.907692307692306,-0.892307692307691,
-0.876923076923076,-0.86153846153846,-0.846153846153845,-0.83076923076923,
-0.815384615384614,-0.799999999999999,-0.784615384615384,-0.769230769230768,
-0.753846153846153,-0.738461538461538,-0.723076923076922,-0.707692307692307,
-0.692307692307692,-0.676923076923076,-0.661538461538461,-0.646153846153846,
-0.63076923076923,-0.615384615384615,-0.6,-0.584615384615384,-0.569230769230769,
-0.553846153846154,-0.538461538461538,-0.523076923076923,-0.507692307692308,
-0.492307692307692,-0.476923076923077,-0.461538461538462,-0.446153846153846,
-0.430769230769231,-0.415384615384615,-0.4,-0.384615384615385,-0.369230769230769,
-0.353846153846154,-0.338461538461538,-0.323076923076923,-0.307692307692308,
-0.292307692307692,-0.276923076923077,-0.261538461538462,-0.246153846153846,
-0.230769230769231,-0.215384615384615,-0.2,-0.184615384615385,-0.169230769230769,
-0.153846153846154,-0.138461538461538,-0.123076923076923,-0.107692307692308,
-0.0923076923076923,-0.0769230769230769,-0.0615384615384615,-0.0461538461538462,
-0.0307692307692308,-0.0153846153846154,0.),(-1.,1.),.UNSPECIFIED.)
GEOMETRIC_REPRESENTATION_ITEM()
RATIONAL_B_SPLINE_SURFACE(((1.,1.),(1.,1.),(1.,1.),(1.,1.),(1.,1.),(1.,
1.),(1.,1.),(1.,1.),(1.,1.),(1.,1.),(1.,1.),(1.,1.),(1.,1.),(1.,1.),(1.,
1.),(1.,1.),(1.,1.),(1.,1.),(1.,1.),(1.,1.),(1.,1.),(1.,1.),(1.,1.),(1.,
1.),(1.,1.),(1.,1.),(1.,1.),(1.,1.),(1.,1.),(1.,1.),(1.,1.),(1.,1.),(1.,
1.),(1.,1.),(1.,1.),(1.,1.),(1.,1.),(1.,1.),(1.,1.),(1.,1.),(1.,1.),(1.,
1.),(1.,1.),(1.,1.),(1.,1.),(1.,1.),(1.,1.),(1.,1.),(1.,1.),(1.,1.),(1.,
1.),(1.,1.),(1.,1.),(1.,1.),(1.,1.),(1.,1.),(1.,1.),(1.,1.),(1.,1.),(1.,
1.),(1.,1.),(1.,1.),(1.,1.),(1.,1.),(1.,1.),(1.,1.),(1.,1.),(1.,1.),(1.,
1.),(1.,1.)))
REPRESENTATION_ITEM('')
SURFACE()
);
#23=(
BOUNDED_SURFACE()
B_SPLINE_SURFACE(5,1,((#32324,#32325),(#32326,#32327),(#32328,#32329),(#32330,
#32331),(#32332,#32333),(#32334,#32335),(#32336,#32337),(#32338,#32339),
(#32340,#32341),(#32342,#32343),(#32344,#32345),(#32346,#32347),(#32348,
#32349),(#32350,#32351),(#32352,#32353),(#32354,#32355),(#32356,#32357),
(#32358,#32359),(#32360,#32361),(#32362,#32363),(#32364,#32365),(#32366,
#32367),(#32368,#32369),(#32370,#32371),(#32372,#32373),(#32374,#32375),
(#32376,#32377),(#32378,#32379),(#32380,#32381),(#32382,#32383),(#32384,
#32385),(#32386,#32387),(#32388,#32389),(#32390,#32391),(#32392,#32393),
(#32394,#32395),(#32396,#32397),(#32398,#32399),(#32400,#32401),(#32402,
#32403),(#32404,#32405),(#32406,#32407),(#32408,#32409),(#32410,#32411),
(#32412,#32413),(#32414,#32415),(#32416,#32417),(#32418,#32419),(#32420,
#32421),(#32422,#32423),(#32424,#32425),(#32426,#32427),(#32428,#32429),
(#32430,#32431),(#32432,#32433),(#32434,#32435),(#32436,#32437),(#32438,
#32439),(#32440,#32441),(#32442,#32443),(#32444,#32445),(#32446,#32447),
(#32448,#32449),(#32450,#32451),(#32452,#32453),(#32454,#32455),(#32456,
#32457),(#32458,#32459),(#32460,#32461),(#32462,#32463)),.UNSPECIFIED.,
 .F.,.F.,.F.)
B_SPLINE_SURFACE_WITH_KNOTS((6,1,1,1,1,1,1,1,1,1,1,1,1,1,1,1,1,1,1,1,1,
1,1,1,1,1,1,1,1,1,1,1,1,1,1,1,1,1,1,1,1,1,1,1,1,1,1,1,1,1,1,1,1,1,1,1,1,
1,1,1,1,1,1,1,1,6),(2,2),(-1.,-0.984615384615383,-0.969230769230768,-0.953846153846152,
-0.938461538461537,-0.923076923076922,-0.907692307692306,-0.892307692307691,
-0.876923076923076,-0.86153846153846,-0.846153846153845,-0.83076923076923,
-0.815384615384614,-0.799999999999999,-0.784615384615384,-0.769230769230768,
-0.753846153846153,-0.738461538461538,-0.723076923076922,-0.707692307692307,
-0.692307692307692,-0.676923076923076,-0.661538461538461,-0.646153846153846,
-0.63076923076923,-0.615384615384615,-0.6,-0.584615384615384,-0.569230769230769,
-0.553846153846154,-0.538461538461538,-0.523076923076923,-0.507692307692308,
-0.492307692307692,-0.476923076923077,-0.461538461538462,-0.446153846153846,
-0.430769230769231,-0.415384615384615,-0.4,-0.384615384615385,-0.369230769230769,
-0.353846153846154,-0.338461538461538,-0.323076923076923,-0.307692307692308,
-0.292307692307692,-0.276923076923077,-0.261538461538462,-0.246153846153846,
-0.230769230769231,-0.215384615384615,-0.2,-0.184615384615385,-0.169230769230769,
-0.153846153846154,-0.138461538461538,-0.123076923076923,-0.107692307692308,
-0.0923076923076923,-0.0769230769230769,-0.0615384615384615,-0.0461538461538462,
-0.0307692307692308,-0.0153846153846154,0.),(-1.,1.),.UNSPECIFIED.)
GEOMETRIC_REPRESENTATION_ITEM()
RATIONAL_B_SPLINE_SURFACE(((1.,1.),(1.,1.),(1.,1.),(1.,1.),(1.,1.),(1.,
1.),(1.,1.),(1.,1.),(1.,1.),(1.,1.),(1.,1.),(1.,1.),(1.,1.),(1.,1.),(1.,
1.),(1.,1.),(1.,1.),(1.,1.),(1.,1.),(1.,1.),(1.,1.),(1.,1.),(1.,1.),(1.,
1.),(1.,1.),(1.,1.),(1.,1.),(1.,1.),(1.,1.),(1.,1.),(1.,1.),(1.,1.),(1.,
1.),(1.,1.),(1.,1.),(1.,1.),(1.,1.),(1.,1.),(1.,1.),(1.,1.),(1.,1.),(1.,
1.),(1.,1.),(1.,1.),(1.,1.),(1.,1.),(1.,1.),(1.,1.),(1.,1.),(1.,1.),(1.,
1.),(1.,1.),(1.,1.),(1.,1.),(1.,1.),(1.,1.),(1.,1.),(1.,1.),(1.,1.),(1.,
1.),(1.,1.),(1.,1.),(1.,1.),(1.,1.),(1.,1.),(1.,1.),(1.,1.),(1.,1.),(1.,
1.),(1.,1.)))
REPRESENTATION_ITEM('')
SURFACE()
);
#24=(
BOUNDED_SURFACE()
B_SPLINE_SURFACE(5,1,((#32540,#32541),(#32542,#32543),(#32544,#32545),(#32546,
#32547),(#32548,#32549),(#32550,#32551),(#32552,#32553),(#32554,#32555),
(#32556,#32557),(#32558,#32559),(#32560,#32561),(#32562,#32563),(#32564,
#32565),(#32566,#32567),(#32568,#32569),(#32570,#32571),(#32572,#32573),
(#32574,#32575),(#32576,#32577),(#32578,#32579),(#32580,#32581),(#32582,
#32583),(#32584,#32585),(#32586,#32587),(#32588,#32589),(#32590,#32591),
(#32592,#32593),(#32594,#32595),(#32596,#32597),(#32598,#32599),(#32600,
#32601),(#32602,#32603),(#32604,#32605),(#32606,#32607),(#32608,#32609),
(#32610,#32611),(#32612,#32613),(#32614,#32615),(#32616,#32617),(#32618,
#32619),(#32620,#32621),(#32622,#32623),(#32624,#32625),(#32626,#32627),
(#32628,#32629),(#32630,#32631),(#32632,#32633),(#32634,#32635),(#32636,
#32637),(#32638,#32639),(#32640,#32641),(#32642,#32643),(#32644,#32645),
(#32646,#32647),(#32648,#32649),(#32650,#32651),(#32652,#32653),(#32654,
#32655),(#32656,#32657),(#32658,#32659),(#32660,#32661),(#32662,#32663),
(#32664,#32665),(#32666,#32667),(#32668,#32669),(#32670,#32671),(#32672,
#32673),(#32674,#32675),(#32676,#32677),(#32678,#32679)),.UNSPECIFIED.,
 .F.,.F.,.F.)
B_SPLINE_SURFACE_WITH_KNOTS((6,1,1,1,1,1,1,1,1,1,1,1,1,1,1,1,1,1,1,1,1,
1,1,1,1,1,1,1,1,1,1,1,1,1,1,1,1,1,1,1,1,1,1,1,1,1,1,1,1,1,1,1,1,1,1,1,1,
1,1,1,1,1,1,1,1,6),(2,2),(-1.,-0.984615384615383,-0.969230769230768,-0.953846153846152,
-0.938461538461537,-0.923076923076922,-0.907692307692306,-0.892307692307691,
-0.876923076923076,-0.86153846153846,-0.846153846153845,-0.83076923076923,
-0.815384615384614,-0.799999999999999,-0.784615384615384,-0.769230769230768,
-0.753846153846153,-0.738461538461538,-0.723076923076922,-0.707692307692307,
-0.692307692307692,-0.676923076923076,-0.661538461538461,-0.646153846153846,
-0.63076923076923,-0.615384615384615,-0.6,-0.584615384615384,-0.569230769230769,
-0.553846153846154,-0.538461538461538,-0.523076923076923,-0.507692307692308,
-0.492307692307692,-0.476923076923077,-0.461538461538462,-0.446153846153846,
-0.430769230769231,-0.415384615384615,-0.4,-0.384615384615385,-0.369230769230769,
-0.353846153846154,-0.338461538461538,-0.323076923076923,-0.307692307692308,
-0.292307692307692,-0.276923076923077,-0.261538461538462,-0.246153846153846,
-0.230769230769231,-0.215384615384615,-0.2,-0.184615384615385,-0.169230769230769,
-0.153846153846154,-0.138461538461538,-0.123076923076923,-0.107692307692308,
-0.0923076923076923,-0.0769230769230769,-0.0615384615384615,-0.0461538461538462,
-0.0307692307692308,-0.0153846153846154,0.),(-1.,1.),.UNSPECIFIED.)
GEOMETRIC_REPRESENTATION_ITEM()
RATIONAL_B_SPLINE_SURFACE(((1.,1.),(1.,1.),(1.,1.),(1.,1.),(1.,1.),(1.,
1.),(1.,1.),(1.,1.),(1.,1.),(1.,1.),(1.,1.),(1.,1.),(1.,1.),(1.,1.),(1.,
1.),(1.,1.),(1.,1.),(1.,1.),(1.,1.),(1.,1.),(1.,1.),(1.,1.),(1.,1.),(1.,
1.),(1.,1.),(1.,1.),(1.,1.),(1.,1.),(1.,1.),(1.,1.),(1.,1.),(1.,1.),(1.,
1.),(1.,1.),(1.,1.),(1.,1.),(1.,1.),(1.,1.),(1.,1.),(1.,1.),(1.,1.),(1.,
1.),(1.,1.),(1.,1.),(1.,1.),(1.,1.),(1.,1.),(1.,1.),(1.,1.),(1.,1.),(1.,
1.),(1.,1.),(1.,1.),(1.,1.),(1.,1.),(1.,1.),(1.,1.),(1.,1.),(1.,1.),(1.,
1.),(1.,1.),(1.,1.),(1.,1.),(1.,1.),(1.,1.),(1.,1.),(1.,1.),(1.,1.),(1.,
1.),(1.,1.)))
REPRESENTATION_ITEM('')
SURFACE()
);
#25=(
BOUNDED_SURFACE()
B_SPLINE_SURFACE(5,1,((#32756,#32757),(#32758,#32759),(#32760,#32761),(#32762,
#32763),(#32764,#32765),(#32766,#32767),(#32768,#32769),(#32770,#32771),
(#32772,#32773),(#32774,#32775),(#32776,#32777),(#32778,#32779),(#32780,
#32781),(#32782,#32783),(#32784,#32785),(#32786,#32787),(#32788,#32789),
(#32790,#32791),(#32792,#32793),(#32794,#32795),(#32796,#32797),(#32798,
#32799),(#32800,#32801),(#32802,#32803),(#32804,#32805),(#32806,#32807),
(#32808,#32809),(#32810,#32811),(#32812,#32813),(#32814,#32815),(#32816,
#32817),(#32818,#32819),(#32820,#32821),(#32822,#32823),(#32824,#32825),
(#32826,#32827),(#32828,#32829),(#32830,#32831),(#32832,#32833),(#32834,
#32835),(#32836,#32837),(#32838,#32839),(#32840,#32841),(#32842,#32843),
(#32844,#32845),(#32846,#32847),(#32848,#32849),(#32850,#32851),(#32852,
#32853),(#32854,#32855),(#32856,#32857),(#32858,#32859),(#32860,#32861),
(#32862,#32863),(#32864,#32865),(#32866,#32867),(#32868,#32869),(#32870,
#32871),(#32872,#32873),(#32874,#32875),(#32876,#32877),(#32878,#32879),
(#32880,#32881),(#32882,#32883),(#32884,#32885),(#32886,#32887),(#32888,
#32889),(#32890,#32891),(#32892,#32893),(#32894,#32895)),.UNSPECIFIED.,
 .F.,.F.,.F.)
B_SPLINE_SURFACE_WITH_KNOTS((6,1,1,1,1,1,1,1,1,1,1,1,1,1,1,1,1,1,1,1,1,
1,1,1,1,1,1,1,1,1,1,1,1,1,1,1,1,1,1,1,1,1,1,1,1,1,1,1,1,1,1,1,1,1,1,1,1,
1,1,1,1,1,1,1,1,6),(2,2),(-1.,-0.984615384615383,-0.969230769230768,-0.953846153846152,
-0.938461538461537,-0.923076923076922,-0.907692307692306,-0.892307692307691,
-0.876923076923076,-0.86153846153846,-0.846153846153845,-0.83076923076923,
-0.815384615384614,-0.799999999999999,-0.784615384615384,-0.769230769230768,
-0.753846153846153,-0.738461538461538,-0.723076923076922,-0.707692307692307,
-0.692307692307692,-0.676923076923076,-0.661538461538461,-0.646153846153846,
-0.63076923076923,-0.615384615384615,-0.6,-0.584615384615384,-0.569230769230769,
-0.553846153846154,-0.538461538461538,-0.523076923076923,-0.507692307692308,
-0.492307692307692,-0.476923076923077,-0.461538461538462,-0.446153846153846,
-0.430769230769231,-0.415384615384615,-0.4,-0.384615384615385,-0.369230769230769,
-0.353846153846154,-0.338461538461538,-0.323076923076923,-0.307692307692308,
-0.292307692307692,-0.276923076923077,-0.261538461538462,-0.246153846153846,
-0.230769230769231,-0.215384615384615,-0.2,-0.184615384615385,-0.169230769230769,
-0.153846153846154,-0.138461538461538,-0.123076923076923,-0.107692307692308,
-0.0923076923076923,-0.0769230769230769,-0.0615384615384615,-0.0461538461538462,
-0.0307692307692308,-0.0153846153846154,0.),(-1.,1.),.UNSPECIFIED.)
GEOMETRIC_REPRESENTATION_ITEM()
RATIONAL_B_SPLINE_SURFACE(((1.,1.),(1.,1.),(1.,1.),(1.,1.),(1.,1.),(1.,
1.),(1.,1.),(1.,1.),(1.,1.),(1.,1.),(1.,1.),(1.,1.),(1.,1.),(1.,1.),(1.,
1.),(1.,1.),(1.,1.),(1.,1.),(1.,1.),(1.,1.),(1.,1.),(1.,1.),(1.,1.),(1.,
1.),(1.,1.),(1.,1.),(1.,1.),(1.,1.),(1.,1.),(1.,1.),(1.,1.),(1.,1.),(1.,
1.),(1.,1.),(1.,1.),(1.,1.),(1.,1.),(1.,1.),(1.,1.),(1.,1.),(1.,1.),(1.,
1.),(1.,1.),(1.,1.),(1.,1.),(1.,1.),(1.,1.),(1.,1.),(1.,1.),(1.,1.),(1.,
1.),(1.,1.),(1.,1.),(1.,1.),(1.,1.),(1.,1.),(1.,1.),(1.,1.),(1.,1.),(1.,
1.),(1.,1.),(1.,1.),(1.,1.),(1.,1.),(1.,1.),(1.,1.),(1.,1.),(1.,1.),(1.,
1.),(1.,1.)))
REPRESENTATION_ITEM('')
SURFACE()
);
#26=(
BOUNDED_SURFACE()
B_SPLINE_SURFACE(5,1,((#32972,#32973),(#32974,#32975),(#32976,#32977),(#32978,
#32979),(#32980,#32981),(#32982,#32983),(#32984,#32985),(#32986,#32987),
(#32988,#32989),(#32990,#32991),(#32992,#32993),(#32994,#32995),(#32996,
#32997),(#32998,#32999),(#33000,#33001),(#33002,#33003),(#33004,#33005),
(#33006,#33007),(#33008,#33009),(#33010,#33011),(#33012,#33013),(#33014,
#33015),(#33016,#33017),(#33018,#33019),(#33020,#33021),(#33022,#33023),
(#33024,#33025),(#33026,#33027),(#33028,#33029),(#33030,#33031),(#33032,
#33033),(#33034,#33035),(#33036,#33037),(#33038,#33039),(#33040,#33041),
(#33042,#33043),(#33044,#33045),(#33046,#33047),(#33048,#33049),(#33050,
#33051),(#33052,#33053),(#33054,#33055),(#33056,#33057),(#33058,#33059),
(#33060,#33061),(#33062,#33063),(#33064,#33065),(#33066,#33067),(#33068,
#33069),(#33070,#33071),(#33072,#33073),(#33074,#33075),(#33076,#33077),
(#33078,#33079),(#33080,#33081),(#33082,#33083),(#33084,#33085),(#33086,
#33087),(#33088,#33089),(#33090,#33091),(#33092,#33093),(#33094,#33095),
(#33096,#33097),(#33098,#33099),(#33100,#33101),(#33102,#33103),(#33104,
#33105),(#33106,#33107),(#33108,#33109),(#33110,#33111)),.UNSPECIFIED.,
 .F.,.F.,.F.)
B_SPLINE_SURFACE_WITH_KNOTS((6,1,1,1,1,1,1,1,1,1,1,1,1,1,1,1,1,1,1,1,1,
1,1,1,1,1,1,1,1,1,1,1,1,1,1,1,1,1,1,1,1,1,1,1,1,1,1,1,1,1,1,1,1,1,1,1,1,
1,1,1,1,1,1,1,1,6),(2,2),(-1.,-0.984615384615383,-0.969230769230768,-0.953846153846152,
-0.938461538461537,-0.923076923076922,-0.907692307692306,-0.892307692307691,
-0.876923076923076,-0.86153846153846,-0.846153846153845,-0.83076923076923,
-0.815384615384614,-0.799999999999999,-0.784615384615384,-0.769230769230768,
-0.753846153846153,-0.738461538461538,-0.723076923076922,-0.707692307692307,
-0.692307692307692,-0.676923076923076,-0.661538461538461,-0.646153846153846,
-0.63076923076923,-0.615384615384615,-0.6,-0.584615384615384,-0.569230769230769,
-0.553846153846154,-0.538461538461538,-0.523076923076923,-0.507692307692308,
-0.492307692307692,-0.476923076923077,-0.461538461538462,-0.446153846153846,
-0.430769230769231,-0.415384615384615,-0.4,-0.384615384615385,-0.369230769230769,
-0.353846153846154,-0.338461538461538,-0.323076923076923,-0.307692307692308,
-0.292307692307692,-0.276923076923077,-0.261538461538462,-0.246153846153846,
-0.230769230769231,-0.215384615384615,-0.2,-0.184615384615385,-0.169230769230769,
-0.153846153846154,-0.138461538461538,-0.123076923076923,-0.107692307692308,
-0.0923076923076923,-0.0769230769230769,-0.0615384615384615,-0.0461538461538462,
-0.0307692307692308,-0.0153846153846154,0.),(-1.,1.),.UNSPECIFIED.)
GEOMETRIC_REPRESENTATION_ITEM()
RATIONAL_B_SPLINE_SURFACE(((1.,1.),(1.,1.),(1.,1.),(1.,1.),(1.,1.),(1.,
1.),(1.,1.),(1.,1.),(1.,1.),(1.,1.),(1.,1.),(1.,1.),(1.,1.),(1.,1.),(1.,
1.),(1.,1.),(1.,1.),(1.,1.),(1.,1.),(1.,1.),(1.,1.),(1.,1.),(1.,1.),(1.,
1.),(1.,1.),(1.,1.),(1.,1.),(1.,1.),(1.,1.),(1.,1.),(1.,1.),(1.,1.),(1.,
1.),(1.,1.),(1.,1.),(1.,1.),(1.,1.),(1.,1.),(1.,1.),(1.,1.),(1.,1.),(1.,
1.),(1.,1.),(1.,1.),(1.,1.),(1.,1.),(1.,1.),(1.,1.),(1.,1.),(1.,1.),(1.,
1.),(1.,1.),(1.,1.),(1.,1.),(1.,1.),(1.,1.),(1.,1.),(1.,1.),(1.,1.),(1.,
1.),(1.,1.),(1.,1.),(1.,1.),(1.,1.),(1.,1.),(1.,1.),(1.,1.),(1.,1.),(1.,
1.),(1.,1.)))
REPRESENTATION_ITEM('')
SURFACE()
);
#27=(
BOUNDED_SURFACE()
B_SPLINE_SURFACE(5,1,((#33188,#33189),(#33190,#33191),(#33192,#33193),(#33194,
#33195),(#33196,#33197),(#33198,#33199),(#33200,#33201),(#33202,#33203),
(#33204,#33205),(#33206,#33207),(#33208,#33209),(#33210,#33211),(#33212,
#33213),(#33214,#33215),(#33216,#33217),(#33218,#33219),(#33220,#33221),
(#33222,#33223),(#33224,#33225),(#33226,#33227),(#33228,#33229),(#33230,
#33231),(#33232,#33233),(#33234,#33235),(#33236,#33237),(#33238,#33239),
(#33240,#33241),(#33242,#33243),(#33244,#33245),(#33246,#33247),(#33248,
#33249),(#33250,#33251),(#33252,#33253),(#33254,#33255),(#33256,#33257),
(#33258,#33259),(#33260,#33261),(#33262,#33263),(#33264,#33265),(#33266,
#33267),(#33268,#33269),(#33270,#33271),(#33272,#33273),(#33274,#33275),
(#33276,#33277),(#33278,#33279),(#33280,#33281),(#33282,#33283),(#33284,
#33285),(#33286,#33287),(#33288,#33289),(#33290,#33291),(#33292,#33293),
(#33294,#33295),(#33296,#33297),(#33298,#33299),(#33300,#33301),(#33302,
#33303),(#33304,#33305),(#33306,#33307),(#33308,#33309),(#33310,#33311),
(#33312,#33313),(#33314,#33315),(#33316,#33317),(#33318,#33319),(#33320,
#33321),(#33322,#33323),(#33324,#33325),(#33326,#33327)),.UNSPECIFIED.,
 .F.,.F.,.F.)
B_SPLINE_SURFACE_WITH_KNOTS((6,1,1,1,1,1,1,1,1,1,1,1,1,1,1,1,1,1,1,1,1,
1,1,1,1,1,1,1,1,1,1,1,1,1,1,1,1,1,1,1,1,1,1,1,1,1,1,1,1,1,1,1,1,1,1,1,1,
1,1,1,1,1,1,1,1,6),(2,2),(-1.,-0.984615384615383,-0.969230769230768,-0.953846153846152,
-0.938461538461537,-0.923076923076922,-0.907692307692306,-0.892307692307691,
-0.876923076923076,-0.86153846153846,-0.846153846153845,-0.83076923076923,
-0.815384615384614,-0.799999999999999,-0.784615384615384,-0.769230769230768,
-0.753846153846153,-0.738461538461538,-0.723076923076922,-0.707692307692307,
-0.692307692307692,-0.676923076923076,-0.661538461538461,-0.646153846153846,
-0.63076923076923,-0.615384615384615,-0.6,-0.584615384615384,-0.569230769230769,
-0.553846153846154,-0.538461538461538,-0.523076923076923,-0.507692307692308,
-0.492307692307692,-0.476923076923077,-0.461538461538462,-0.446153846153846,
-0.430769230769231,-0.415384615384615,-0.4,-0.384615384615385,-0.369230769230769,
-0.353846153846154,-0.338461538461538,-0.323076923076923,-0.307692307692308,
-0.292307692307692,-0.276923076923077,-0.261538461538462,-0.246153846153846,
-0.230769230769231,-0.215384615384615,-0.2,-0.184615384615385,-0.169230769230769,
-0.153846153846154,-0.138461538461538,-0.123076923076923,-0.107692307692308,
-0.0923076923076923,-0.0769230769230769,-0.0615384615384615,-0.0461538461538462,
-0.0307692307692308,-0.0153846153846154,0.),(-1.,1.),.UNSPECIFIED.)
GEOMETRIC_REPRESENTATION_ITEM()
RATIONAL_B_SPLINE_SURFACE(((1.,1.),(1.,1.),(1.,1.),(1.,1.),(1.,1.),(1.,
1.),(1.,1.),(1.,1.),(1.,1.),(1.,1.),(1.,1.),(1.,1.),(1.,1.),(1.,1.),(1.,
1.),(1.,1.),(1.,1.),(1.,1.),(1.,1.),(1.,1.),(1.,1.),(1.,1.),(1.,1.),(1.,
1.),(1.,1.),(1.,1.),(1.,1.),(1.,1.),(1.,1.),(1.,1.),(1.,1.),(1.,1.),(1.,
1.),(1.,1.),(1.,1.),(1.,1.),(1.,1.),(1.,1.),(1.,1.),(1.,1.),(1.,1.),(1.,
1.),(1.,1.),(1.,1.),(1.,1.),(1.,1.),(1.,1.),(1.,1.),(1.,1.),(1.,1.),(1.,
1.),(1.,1.),(1.,1.),(1.,1.),(1.,1.),(1.,1.),(1.,1.),(1.,1.),(1.,1.),(1.,
1.),(1.,1.),(1.,1.),(1.,1.),(1.,1.),(1.,1.),(1.,1.),(1.,1.),(1.,1.),(1.,
1.),(1.,1.)))
REPRESENTATION_ITEM('')
SURFACE()
);
#28=(
BOUNDED_SURFACE()
B_SPLINE_SURFACE(5,1,((#33404,#33405),(#33406,#33407),(#33408,#33409),(#33410,
#33411),(#33412,#33413),(#33414,#33415),(#33416,#33417),(#33418,#33419),
(#33420,#33421),(#33422,#33423),(#33424,#33425),(#33426,#33427),(#33428,
#33429),(#33430,#33431),(#33432,#33433),(#33434,#33435),(#33436,#33437),
(#33438,#33439),(#33440,#33441),(#33442,#33443),(#33444,#33445),(#33446,
#33447),(#33448,#33449),(#33450,#33451),(#33452,#33453),(#33454,#33455),
(#33456,#33457),(#33458,#33459),(#33460,#33461),(#33462,#33463),(#33464,
#33465),(#33466,#33467),(#33468,#33469),(#33470,#33471),(#33472,#33473),
(#33474,#33475),(#33476,#33477),(#33478,#33479),(#33480,#33481),(#33482,
#33483),(#33484,#33485),(#33486,#33487),(#33488,#33489),(#33490,#33491),
(#33492,#33493),(#33494,#33495),(#33496,#33497),(#33498,#33499),(#33500,
#33501),(#33502,#33503),(#33504,#33505),(#33506,#33507),(#33508,#33509),
(#33510,#33511),(#33512,#33513),(#33514,#33515),(#33516,#33517),(#33518,
#33519),(#33520,#33521),(#33522,#33523),(#33524,#33525),(#33526,#33527),
(#33528,#33529),(#33530,#33531),(#33532,#33533),(#33534,#33535),(#33536,
#33537),(#33538,#33539),(#33540,#33541),(#33542,#33543)),.UNSPECIFIED.,
 .F.,.F.,.F.)
B_SPLINE_SURFACE_WITH_KNOTS((6,1,1,1,1,1,1,1,1,1,1,1,1,1,1,1,1,1,1,1,1,
1,1,1,1,1,1,1,1,1,1,1,1,1,1,1,1,1,1,1,1,1,1,1,1,1,1,1,1,1,1,1,1,1,1,1,1,
1,1,1,1,1,1,1,1,6),(2,2),(-1.,-0.984615384615383,-0.969230769230768,-0.953846153846152,
-0.938461538461537,-0.923076923076922,-0.907692307692306,-0.892307692307691,
-0.876923076923076,-0.86153846153846,-0.846153846153845,-0.83076923076923,
-0.815384615384614,-0.799999999999999,-0.784615384615384,-0.769230769230768,
-0.753846153846153,-0.738461538461538,-0.723076923076922,-0.707692307692307,
-0.692307692307692,-0.676923076923076,-0.661538461538461,-0.646153846153846,
-0.63076923076923,-0.615384615384615,-0.6,-0.584615384615384,-0.569230769230769,
-0.553846153846154,-0.538461538461538,-0.523076923076923,-0.507692307692308,
-0.492307692307692,-0.476923076923077,-0.461538461538462,-0.446153846153846,
-0.430769230769231,-0.415384615384615,-0.4,-0.384615384615385,-0.369230769230769,
-0.353846153846154,-0.338461538461538,-0.323076923076923,-0.307692307692308,
-0.292307692307692,-0.276923076923077,-0.261538461538462,-0.246153846153846,
-0.230769230769231,-0.215384615384615,-0.2,-0.184615384615385,-0.169230769230769,
-0.153846153846154,-0.138461538461538,-0.123076923076923,-0.107692307692308,
-0.0923076923076923,-0.0769230769230769,-0.0615384615384615,-0.0461538461538462,
-0.0307692307692308,-0.0153846153846154,0.),(-1.,1.),.UNSPECIFIED.)
GEOMETRIC_REPRESENTATION_ITEM()
RATIONAL_B_SPLINE_SURFACE(((1.,1.),(1.,1.),(1.,1.),(1.,1.),(1.,1.),(1.,
1.),(1.,1.),(1.,1.),(1.,1.),(1.,1.),(1.,1.),(1.,1.),(1.,1.),(1.,1.),(1.,
1.),(1.,1.),(1.,1.),(1.,1.),(1.,1.),(1.,1.),(1.,1.),(1.,1.),(1.,1.),(1.,
1.),(1.,1.),(1.,1.),(1.,1.),(1.,1.),(1.,1.),(1.,1.),(1.,1.),(1.,1.),(1.,
1.),(1.,1.),(1.,1.),(1.,1.),(1.,1.),(1.,1.),(1.,1.),(1.,1.),(1.,1.),(1.,
1.),(1.,1.),(1.,1.),(1.,1.),(1.,1.),(1.,1.),(1.,1.),(1.,1.),(1.,1.),(1.,
1.),(1.,1.),(1.,1.),(1.,1.),(1.,1.),(1.,1.),(1.,1.),(1.,1.),(1.,1.),(1.,
1.),(1.,1.),(1.,1.),(1.,1.),(1.,1.),(1.,1.),(1.,1.),(1.,1.),(1.,1.),(1.,
1.),(1.,1.)))
REPRESENTATION_ITEM('')
SURFACE()
);
#29=(
BOUNDED_SURFACE()
B_SPLINE_SURFACE(5,1,((#33620,#33621),(#33622,#33623),(#33624,#33625),(#33626,
#33627),(#33628,#33629),(#33630,#33631),(#33632,#33633),(#33634,#33635),
(#33636,#33637),(#33638,#33639),(#33640,#33641),(#33642,#33643),(#33644,
#33645),(#33646,#33647),(#33648,#33649),(#33650,#33651),(#33652,#33653),
(#33654,#33655),(#33656,#33657),(#33658,#33659),(#33660,#33661),(#33662,
#33663),(#33664,#33665),(#33666,#33667),(#33668,#33669),(#33670,#33671),
(#33672,#33673),(#33674,#33675),(#33676,#33677),(#33678,#33679),(#33680,
#33681),(#33682,#33683),(#33684,#33685),(#33686,#33687),(#33688,#33689),
(#33690,#33691),(#33692,#33693),(#33694,#33695),(#33696,#33697),(#33698,
#33699),(#33700,#33701),(#33702,#33703),(#33704,#33705),(#33706,#33707),
(#33708,#33709),(#33710,#33711),(#33712,#33713),(#33714,#33715),(#33716,
#33717),(#33718,#33719),(#33720,#33721),(#33722,#33723),(#33724,#33725),
(#33726,#33727),(#33728,#33729),(#33730,#33731),(#33732,#33733),(#33734,
#33735),(#33736,#33737),(#33738,#33739),(#33740,#33741),(#33742,#33743),
(#33744,#33745),(#33746,#33747),(#33748,#33749),(#33750,#33751),(#33752,
#33753),(#33754,#33755),(#33756,#33757),(#33758,#33759)),.UNSPECIFIED.,
 .F.,.F.,.F.)
B_SPLINE_SURFACE_WITH_KNOTS((6,1,1,1,1,1,1,1,1,1,1,1,1,1,1,1,1,1,1,1,1,
1,1,1,1,1,1,1,1,1,1,1,1,1,1,1,1,1,1,1,1,1,1,1,1,1,1,1,1,1,1,1,1,1,1,1,1,
1,1,1,1,1,1,1,1,6),(2,2),(-1.,-0.984615384615383,-0.969230769230768,-0.953846153846152,
-0.938461538461537,-0.923076923076922,-0.907692307692306,-0.892307692307691,
-0.876923076923076,-0.86153846153846,-0.846153846153845,-0.83076923076923,
-0.815384615384614,-0.799999999999999,-0.784615384615384,-0.769230769230768,
-0.753846153846153,-0.738461538461538,-0.723076923076922,-0.707692307692307,
-0.692307692307692,-0.676923076923076,-0.661538461538461,-0.646153846153846,
-0.63076923076923,-0.615384615384615,-0.6,-0.584615384615384,-0.569230769230769,
-0.553846153846154,-0.538461538461538,-0.523076923076923,-0.507692307692308,
-0.492307692307692,-0.476923076923077,-0.461538461538462,-0.446153846153846,
-0.430769230769231,-0.415384615384615,-0.4,-0.384615384615385,-0.369230769230769,
-0.353846153846154,-0.338461538461538,-0.323076923076923,-0.307692307692308,
-0.292307692307692,-0.276923076923077,-0.261538461538462,-0.246153846153846,
-0.230769230769231,-0.215384615384615,-0.2,-0.184615384615385,-0.169230769230769,
-0.153846153846154,-0.138461538461538,-0.123076923076923,-0.107692307692308,
-0.0923076923076923,-0.0769230769230769,-0.0615384615384615,-0.0461538461538462,
-0.0307692307692308,-0.0153846153846154,0.),(-1.,1.),.UNSPECIFIED.)
GEOMETRIC_REPRESENTATION_ITEM()
RATIONAL_B_SPLINE_SURFACE(((1.,1.),(1.,1.),(1.,1.),(1.,1.),(1.,1.),(1.,
1.),(1.,1.),(1.,1.),(1.,1.),(1.,1.),(1.,1.),(1.,1.),(1.,1.),(1.,1.),(1.,
1.),(1.,1.),(1.,1.),(1.,1.),(1.,1.),(1.,1.),(1.,1.),(1.,1.),(1.,1.),(1.,
1.),(1.,1.),(1.,1.),(1.,1.),(1.,1.),(1.,1.),(1.,1.),(1.,1.),(1.,1.),(1.,
1.),(1.,1.),(1.,1.),(1.,1.),(1.,1.),(1.,1.),(1.,1.),(1.,1.),(1.,1.),(1.,
1.),(1.,1.),(1.,1.),(1.,1.),(1.,1.),(1.,1.),(1.,1.),(1.,1.),(1.,1.),(1.,
1.),(1.,1.),(1.,1.),(1.,1.),(1.,1.),(1.,1.),(1.,1.),(1.,1.),(1.,1.),(1.,
1.),(1.,1.),(1.,1.),(1.,1.),(1.,1.),(1.,1.),(1.,1.),(1.,1.),(1.,1.),(1.,
1.),(1.,1.)))
REPRESENTATION_ITEM('')
SURFACE()
);
#30=(
BOUNDED_SURFACE()
B_SPLINE_SURFACE(5,1,((#33836,#33837),(#33838,#33839),(#33840,#33841),(#33842,
#33843),(#33844,#33845),(#33846,#33847),(#33848,#33849),(#33850,#33851),
(#33852,#33853),(#33854,#33855),(#33856,#33857),(#33858,#33859),(#33860,
#33861),(#33862,#33863),(#33864,#33865),(#33866,#33867),(#33868,#33869),
(#33870,#33871),(#33872,#33873),(#33874,#33875),(#33876,#33877),(#33878,
#33879),(#33880,#33881),(#33882,#33883),(#33884,#33885),(#33886,#33887),
(#33888,#33889),(#33890,#33891),(#33892,#33893),(#33894,#33895),(#33896,
#33897),(#33898,#33899),(#33900,#33901),(#33902,#33903),(#33904,#33905),
(#33906,#33907),(#33908,#33909),(#33910,#33911),(#33912,#33913),(#33914,
#33915),(#33916,#33917),(#33918,#33919),(#33920,#33921),(#33922,#33923),
(#33924,#33925),(#33926,#33927),(#33928,#33929),(#33930,#33931),(#33932,
#33933),(#33934,#33935),(#33936,#33937),(#33938,#33939),(#33940,#33941),
(#33942,#33943),(#33944,#33945),(#33946,#33947),(#33948,#33949),(#33950,
#33951),(#33952,#33953),(#33954,#33955),(#33956,#33957),(#33958,#33959),
(#33960,#33961),(#33962,#33963),(#33964,#33965),(#33966,#33967),(#33968,
#33969),(#33970,#33971),(#33972,#33973),(#33974,#33975)),.UNSPECIFIED.,
 .F.,.F.,.F.)
B_SPLINE_SURFACE_WITH_KNOTS((6,1,1,1,1,1,1,1,1,1,1,1,1,1,1,1,1,1,1,1,1,
1,1,1,1,1,1,1,1,1,1,1,1,1,1,1,1,1,1,1,1,1,1,1,1,1,1,1,1,1,1,1,1,1,1,1,1,
1,1,1,1,1,1,1,1,6),(2,2),(-1.,-0.984615384615383,-0.969230769230768,-0.953846153846152,
-0.938461538461537,-0.923076923076922,-0.907692307692306,-0.892307692307691,
-0.876923076923076,-0.86153846153846,-0.846153846153845,-0.83076923076923,
-0.815384615384614,-0.799999999999999,-0.784615384615384,-0.769230769230768,
-0.753846153846153,-0.738461538461538,-0.723076923076922,-0.707692307692307,
-0.692307692307692,-0.676923076923076,-0.661538461538461,-0.646153846153846,
-0.63076923076923,-0.615384615384615,-0.6,-0.584615384615384,-0.569230769230769,
-0.553846153846154,-0.538461538461538,-0.523076923076923,-0.507692307692308,
-0.492307692307692,-0.476923076923077,-0.461538461538462,-0.446153846153846,
-0.430769230769231,-0.415384615384615,-0.4,-0.384615384615385,-0.369230769230769,
-0.353846153846154,-0.338461538461538,-0.323076923076923,-0.307692307692308,
-0.292307692307692,-0.276923076923077,-0.261538461538462,-0.246153846153846,
-0.230769230769231,-0.215384615384615,-0.2,-0.184615384615385,-0.169230769230769,
-0.153846153846154,-0.138461538461538,-0.123076923076923,-0.107692307692308,
-0.0923076923076923,-0.0769230769230769,-0.0615384615384615,-0.0461538461538462,
-0.0307692307692308,-0.0153846153846154,0.),(-1.,1.),.UNSPECIFIED.)
GEOMETRIC_REPRESENTATION_ITEM()
RATIONAL_B_SPLINE_SURFACE(((1.,1.),(1.,1.),(1.,1.),(1.,1.),(1.,1.),(1.,
1.),(1.,1.),(1.,1.),(1.,1.),(1.,1.),(1.,1.),(1.,1.),(1.,1.),(1.,1.),(1.,
1.),(1.,1.),(1.,1.),(1.,1.),(1.,1.),(1.,1.),(1.,1.),(1.,1.),(1.,1.),(1.,
1.),(1.,1.),(1.,1.),(1.,1.),(1.,1.),(1.,1.),(1.,1.),(1.,1.),(1.,1.),(1.,
1.),(1.,1.),(1.,1.),(1.,1.),(1.,1.),(1.,1.),(1.,1.),(1.,1.),(1.,1.),(1.,
1.),(1.,1.),(1.,1.),(1.,1.),(1.,1.),(1.,1.),(1.,1.),(1.,1.),(1.,1.),(1.,
1.),(1.,1.),(1.,1.),(1.,1.),(1.,1.),(1.,1.),(1.,1.),(1.,1.),(1.,1.),(1.,
1.),(1.,1.),(1.,1.),(1.,1.),(1.,1.),(1.,1.),(1.,1.),(1.,1.),(1.,1.),(1.,
1.),(1.,1.)))
REPRESENTATION_ITEM('')
SURFACE()
);
#31=(
BOUNDED_SURFACE()
B_SPLINE_SURFACE(5,1,((#34052,#34053),(#34054,#34055),(#34056,#34057),(#34058,
#34059),(#34060,#34061),(#34062,#34063),(#34064,#34065),(#34066,#34067),
(#34068,#34069),(#34070,#34071),(#34072,#34073),(#34074,#34075),(#34076,
#34077),(#34078,#34079),(#34080,#34081),(#34082,#34083),(#34084,#34085),
(#34086,#34087),(#34088,#34089),(#34090,#34091),(#34092,#34093),(#34094,
#34095),(#34096,#34097),(#34098,#34099),(#34100,#34101),(#34102,#34103),
(#34104,#34105),(#34106,#34107),(#34108,#34109),(#34110,#34111),(#34112,
#34113),(#34114,#34115),(#34116,#34117),(#34118,#34119),(#34120,#34121),
(#34122,#34123),(#34124,#34125),(#34126,#34127),(#34128,#34129),(#34130,
#34131),(#34132,#34133),(#34134,#34135),(#34136,#34137),(#34138,#34139),
(#34140,#34141),(#34142,#34143),(#34144,#34145),(#34146,#34147),(#34148,
#34149),(#34150,#34151),(#34152,#34153),(#34154,#34155),(#34156,#34157),
(#34158,#34159),(#34160,#34161),(#34162,#34163),(#34164,#34165),(#34166,
#34167),(#34168,#34169),(#34170,#34171),(#34172,#34173),(#34174,#34175),
(#34176,#34177),(#34178,#34179),(#34180,#34181),(#34182,#34183),(#34184,
#34185),(#34186,#34187),(#34188,#34189),(#34190,#34191)),.UNSPECIFIED.,
 .F.,.F.,.F.)
B_SPLINE_SURFACE_WITH_KNOTS((6,1,1,1,1,1,1,1,1,1,1,1,1,1,1,1,1,1,1,1,1,
1,1,1,1,1,1,1,1,1,1,1,1,1,1,1,1,1,1,1,1,1,1,1,1,1,1,1,1,1,1,1,1,1,1,1,1,
1,1,1,1,1,1,1,1,6),(2,2),(-1.,-0.984615384615383,-0.969230769230768,-0.953846153846152,
-0.938461538461537,-0.923076923076922,-0.907692307692306,-0.892307692307691,
-0.876923076923076,-0.86153846153846,-0.846153846153845,-0.83076923076923,
-0.815384615384614,-0.799999999999999,-0.784615384615384,-0.769230769230768,
-0.753846153846153,-0.738461538461538,-0.723076923076922,-0.707692307692307,
-0.692307692307692,-0.676923076923076,-0.661538461538461,-0.646153846153846,
-0.63076923076923,-0.615384615384615,-0.6,-0.584615384615384,-0.569230769230769,
-0.553846153846154,-0.538461538461538,-0.523076923076923,-0.507692307692308,
-0.492307692307692,-0.476923076923077,-0.461538461538462,-0.446153846153846,
-0.430769230769231,-0.415384615384615,-0.4,-0.384615384615385,-0.369230769230769,
-0.353846153846154,-0.338461538461538,-0.323076923076923,-0.307692307692308,
-0.292307692307692,-0.276923076923077,-0.261538461538462,-0.246153846153846,
-0.230769230769231,-0.215384615384615,-0.2,-0.184615384615385,-0.169230769230769,
-0.153846153846154,-0.138461538461538,-0.123076923076923,-0.107692307692308,
-0.0923076923076923,-0.0769230769230769,-0.0615384615384615,-0.0461538461538462,
-0.0307692307692308,-0.0153846153846154,0.),(-1.,1.),.UNSPECIFIED.)
GEOMETRIC_REPRESENTATION_ITEM()
RATIONAL_B_SPLINE_SURFACE(((1.,1.),(1.,1.),(1.,1.),(1.,1.),(1.,1.),(1.,
1.),(1.,1.),(1.,1.),(1.,1.),(1.,1.),(1.,1.),(1.,1.),(1.,1.),(1.,1.),(1.,
1.),(1.,1.),(1.,1.),(1.,1.),(1.,1.),(1.,1.),(1.,1.),(1.,1.),(1.,1.),(1.,
1.),(1.,1.),(1.,1.),(1.,1.),(1.,1.),(1.,1.),(1.,1.),(1.,1.),(1.,1.),(1.,
1.),(1.,1.),(1.,1.),(1.,1.),(1.,1.),(1.,1.),(1.,1.),(1.,1.),(1.,1.),(1.,
1.),(1.,1.),(1.,1.),(1.,1.),(1.,1.),(1.,1.),(1.,1.),(1.,1.),(1.,1.),(1.,
1.),(1.,1.),(1.,1.),(1.,1.),(1.,1.),(1.,1.),(1.,1.),(1.,1.),(1.,1.),(1.,
1.),(1.,1.),(1.,1.),(1.,1.),(1.,1.),(1.,1.),(1.,1.),(1.,1.),(1.,1.),(1.,
1.),(1.,1.)))
REPRESENTATION_ITEM('')
SURFACE()
);
#32=(
BOUNDED_SURFACE()
B_SPLINE_SURFACE(5,1,((#34268,#34269),(#34270,#34271),(#34272,#34273),(#34274,
#34275),(#34276,#34277),(#34278,#34279),(#34280,#34281),(#34282,#34283),
(#34284,#34285),(#34286,#34287),(#34288,#34289),(#34290,#34291),(#34292,
#34293),(#34294,#34295),(#34296,#34297),(#34298,#34299),(#34300,#34301),
(#34302,#34303),(#34304,#34305),(#34306,#34307),(#34308,#34309),(#34310,
#34311),(#34312,#34313),(#34314,#34315),(#34316,#34317),(#34318,#34319),
(#34320,#34321),(#34322,#34323),(#34324,#34325),(#34326,#34327),(#34328,
#34329),(#34330,#34331),(#34332,#34333),(#34334,#34335),(#34336,#34337),
(#34338,#34339),(#34340,#34341),(#34342,#34343),(#34344,#34345),(#34346,
#34347),(#34348,#34349),(#34350,#34351),(#34352,#34353),(#34354,#34355),
(#34356,#34357),(#34358,#34359),(#34360,#34361),(#34362,#34363),(#34364,
#34365),(#34366,#34367),(#34368,#34369),(#34370,#34371),(#34372,#34373),
(#34374,#34375),(#34376,#34377),(#34378,#34379),(#34380,#34381),(#34382,
#34383),(#34384,#34385),(#34386,#34387),(#34388,#34389),(#34390,#34391),
(#34392,#34393),(#34394,#34395),(#34396,#34397),(#34398,#34399),(#34400,
#34401),(#34402,#34403),(#34404,#34405),(#34406,#34407)),.UNSPECIFIED.,
 .F.,.F.,.F.)
B_SPLINE_SURFACE_WITH_KNOTS((6,1,1,1,1,1,1,1,1,1,1,1,1,1,1,1,1,1,1,1,1,
1,1,1,1,1,1,1,1,1,1,1,1,1,1,1,1,1,1,1,1,1,1,1,1,1,1,1,1,1,1,1,1,1,1,1,1,
1,1,1,1,1,1,1,1,6),(2,2),(-1.,-0.984615384615383,-0.969230769230768,-0.953846153846152,
-0.938461538461537,-0.923076923076922,-0.907692307692306,-0.892307692307691,
-0.876923076923076,-0.86153846153846,-0.846153846153845,-0.83076923076923,
-0.815384615384614,-0.799999999999999,-0.784615384615384,-0.769230769230768,
-0.753846153846153,-0.738461538461538,-0.723076923076922,-0.707692307692307,
-0.692307692307692,-0.676923076923076,-0.661538461538461,-0.646153846153846,
-0.63076923076923,-0.615384615384615,-0.6,-0.584615384615384,-0.569230769230769,
-0.553846153846154,-0.538461538461538,-0.523076923076923,-0.507692307692308,
-0.492307692307692,-0.476923076923077,-0.461538461538462,-0.446153846153846,
-0.430769230769231,-0.415384615384615,-0.4,-0.384615384615385,-0.369230769230769,
-0.353846153846154,-0.338461538461538,-0.323076923076923,-0.307692307692308,
-0.292307692307692,-0.276923076923077,-0.261538461538462,-0.246153846153846,
-0.230769230769231,-0.215384615384615,-0.2,-0.184615384615385,-0.169230769230769,
-0.153846153846154,-0.138461538461538,-0.123076923076923,-0.107692307692308,
-0.0923076923076923,-0.0769230769230769,-0.0615384615384615,-0.0461538461538462,
-0.0307692307692308,-0.0153846153846154,0.),(-1.,1.),.UNSPECIFIED.)
GEOMETRIC_REPRESENTATION_ITEM()
RATIONAL_B_SPLINE_SURFACE(((1.,1.),(1.,1.),(1.,1.),(1.,1.),(1.,1.),(1.,
1.),(1.,1.),(1.,1.),(1.,1.),(1.,1.),(1.,1.),(1.,1.),(1.,1.),(1.,1.),(1.,
1.),(1.,1.),(1.,1.),(1.,1.),(1.,1.),(1.,1.),(1.,1.),(1.,1.),(1.,1.),(1.,
1.),(1.,1.),(1.,1.),(1.,1.),(1.,1.),(1.,1.),(1.,1.),(1.,1.),(1.,1.),(1.,
1.),(1.,1.),(1.,1.),(1.,1.),(1.,1.),(1.,1.),(1.,1.),(1.,1.),(1.,1.),(1.,
1.),(1.,1.),(1.,1.),(1.,1.),(1.,1.),(1.,1.),(1.,1.),(1.,1.),(1.,1.),(1.,
1.),(1.,1.),(1.,1.),(1.,1.),(1.,1.),(1.,1.),(1.,1.),(1.,1.),(1.,1.),(1.,
1.),(1.,1.),(1.,1.),(1.,1.),(1.,1.),(1.,1.),(1.,1.),(1.,1.),(1.,1.),(1.,
1.),(1.,1.)))
REPRESENTATION_ITEM('')
SURFACE()
);
#33=(
BOUNDED_SURFACE()
B_SPLINE_SURFACE(5,1,((#34484,#34485),(#34486,#34487),(#34488,#34489),(#34490,
#34491),(#34492,#34493),(#34494,#34495),(#34496,#34497),(#34498,#34499),
(#34500,#34501),(#34502,#34503),(#34504,#34505),(#34506,#34507),(#34508,
#34509),(#34510,#34511),(#34512,#34513),(#34514,#34515),(#34516,#34517),
(#34518,#34519),(#34520,#34521),(#34522,#34523),(#34524,#34525),(#34526,
#34527),(#34528,#34529),(#34530,#34531),(#34532,#34533),(#34534,#34535),
(#34536,#34537),(#34538,#34539),(#34540,#34541),(#34542,#34543),(#34544,
#34545),(#34546,#34547),(#34548,#34549),(#34550,#34551),(#34552,#34553),
(#34554,#34555),(#34556,#34557),(#34558,#34559),(#34560,#34561),(#34562,
#34563),(#34564,#34565),(#34566,#34567),(#34568,#34569),(#34570,#34571),
(#34572,#34573),(#34574,#34575),(#34576,#34577),(#34578,#34579),(#34580,
#34581),(#34582,#34583),(#34584,#34585),(#34586,#34587),(#34588,#34589),
(#34590,#34591),(#34592,#34593),(#34594,#34595),(#34596,#34597),(#34598,
#34599),(#34600,#34601),(#34602,#34603),(#34604,#34605),(#34606,#34607),
(#34608,#34609),(#34610,#34611),(#34612,#34613),(#34614,#34615),(#34616,
#34617),(#34618,#34619),(#34620,#34621),(#34622,#34623)),.UNSPECIFIED.,
 .F.,.F.,.F.)
B_SPLINE_SURFACE_WITH_KNOTS((6,1,1,1,1,1,1,1,1,1,1,1,1,1,1,1,1,1,1,1,1,
1,1,1,1,1,1,1,1,1,1,1,1,1,1,1,1,1,1,1,1,1,1,1,1,1,1,1,1,1,1,1,1,1,1,1,1,
1,1,1,1,1,1,1,1,6),(2,2),(-1.,-0.984615384615383,-0.969230769230768,-0.953846153846152,
-0.938461538461537,-0.923076923076922,-0.907692307692306,-0.892307692307691,
-0.876923076923076,-0.86153846153846,-0.846153846153845,-0.83076923076923,
-0.815384615384614,-0.799999999999999,-0.784615384615384,-0.769230769230768,
-0.753846153846153,-0.738461538461538,-0.723076923076922,-0.707692307692307,
-0.692307692307692,-0.676923076923076,-0.661538461538461,-0.646153846153846,
-0.63076923076923,-0.615384615384615,-0.6,-0.584615384615384,-0.569230769230769,
-0.553846153846154,-0.538461538461538,-0.523076923076923,-0.507692307692308,
-0.492307692307692,-0.476923076923077,-0.461538461538462,-0.446153846153846,
-0.430769230769231,-0.415384615384615,-0.4,-0.384615384615385,-0.369230769230769,
-0.353846153846154,-0.338461538461538,-0.323076923076923,-0.307692307692308,
-0.292307692307692,-0.276923076923077,-0.261538461538462,-0.246153846153846,
-0.230769230769231,-0.215384615384615,-0.2,-0.184615384615385,-0.169230769230769,
-0.153846153846154,-0.138461538461538,-0.123076923076923,-0.107692307692308,
-0.0923076923076923,-0.0769230769230769,-0.0615384615384615,-0.0461538461538462,
-0.0307692307692308,-0.0153846153846154,0.),(-1.,1.),.UNSPECIFIED.)
GEOMETRIC_REPRESENTATION_ITEM()
RATIONAL_B_SPLINE_SURFACE(((1.,1.),(1.,1.),(1.,1.),(1.,1.),(1.,1.),(1.,
1.),(1.,1.),(1.,1.),(1.,1.),(1.,1.),(1.,1.),(1.,1.),(1.,1.),(1.,1.),(1.,
1.),(1.,1.),(1.,1.),(1.,1.),(1.,1.),(1.,1.),(1.,1.),(1.,1.),(1.,1.),(1.,
1.),(1.,1.),(1.,1.),(1.,1.),(1.,1.),(1.,1.),(1.,1.),(1.,1.),(1.,1.),(1.,
1.),(1.,1.),(1.,1.),(1.,1.),(1.,1.),(1.,1.),(1.,1.),(1.,1.),(1.,1.),(1.,
1.),(1.,1.),(1.,1.),(1.,1.),(1.,1.),(1.,1.),(1.,1.),(1.,1.),(1.,1.),(1.,
1.),(1.,1.),(1.,1.),(1.,1.),(1.,1.),(1.,1.),(1.,1.),(1.,1.),(1.,1.),(1.,
1.),(1.,1.),(1.,1.),(1.,1.),(1.,1.),(1.,1.),(1.,1.),(1.,1.),(1.,1.),(1.,
1.),(1.,1.)))
REPRESENTATION_ITEM('')
SURFACE()
);
#34=(
BOUNDED_SURFACE()
B_SPLINE_SURFACE(5,1,((#34700,#34701),(#34702,#34703),(#34704,#34705),(#34706,
#34707),(#34708,#34709),(#34710,#34711),(#34712,#34713),(#34714,#34715),
(#34716,#34717),(#34718,#34719),(#34720,#34721),(#34722,#34723),(#34724,
#34725),(#34726,#34727),(#34728,#34729),(#34730,#34731),(#34732,#34733),
(#34734,#34735),(#34736,#34737),(#34738,#34739),(#34740,#34741),(#34742,
#34743),(#34744,#34745),(#34746,#34747),(#34748,#34749),(#34750,#34751),
(#34752,#34753),(#34754,#34755),(#34756,#34757),(#34758,#34759),(#34760,
#34761),(#34762,#34763),(#34764,#34765),(#34766,#34767),(#34768,#34769),
(#34770,#34771),(#34772,#34773),(#34774,#34775),(#34776,#34777),(#34778,
#34779),(#34780,#34781),(#34782,#34783),(#34784,#34785),(#34786,#34787),
(#34788,#34789),(#34790,#34791),(#34792,#34793),(#34794,#34795),(#34796,
#34797),(#34798,#34799),(#34800,#34801),(#34802,#34803),(#34804,#34805),
(#34806,#34807),(#34808,#34809),(#34810,#34811),(#34812,#34813),(#34814,
#34815),(#34816,#34817),(#34818,#34819),(#34820,#34821),(#34822,#34823),
(#34824,#34825),(#34826,#34827),(#34828,#34829),(#34830,#34831),(#34832,
#34833),(#34834,#34835),(#34836,#34837),(#34838,#34839)),.UNSPECIFIED.,
 .F.,.F.,.F.)
B_SPLINE_SURFACE_WITH_KNOTS((6,1,1,1,1,1,1,1,1,1,1,1,1,1,1,1,1,1,1,1,1,
1,1,1,1,1,1,1,1,1,1,1,1,1,1,1,1,1,1,1,1,1,1,1,1,1,1,1,1,1,1,1,1,1,1,1,1,
1,1,1,1,1,1,1,1,6),(2,2),(-1.,-0.984615384615383,-0.969230769230768,-0.953846153846152,
-0.938461538461537,-0.923076923076922,-0.907692307692306,-0.892307692307691,
-0.876923076923076,-0.86153846153846,-0.846153846153845,-0.83076923076923,
-0.815384615384614,-0.799999999999999,-0.784615384615384,-0.769230769230768,
-0.753846153846153,-0.738461538461538,-0.723076923076922,-0.707692307692307,
-0.692307692307692,-0.676923076923076,-0.661538461538461,-0.646153846153846,
-0.63076923076923,-0.615384615384615,-0.6,-0.584615384615384,-0.569230769230769,
-0.553846153846154,-0.538461538461538,-0.523076923076923,-0.507692307692308,
-0.492307692307692,-0.476923076923077,-0.461538461538462,-0.446153846153846,
-0.430769230769231,-0.415384615384615,-0.4,-0.384615384615385,-0.369230769230769,
-0.353846153846154,-0.338461538461538,-0.323076923076923,-0.307692307692308,
-0.292307692307692,-0.276923076923077,-0.261538461538462,-0.246153846153846,
-0.230769230769231,-0.215384615384615,-0.2,-0.184615384615385,-0.169230769230769,
-0.153846153846154,-0.138461538461538,-0.123076923076923,-0.107692307692308,
-0.0923076923076923,-0.0769230769230769,-0.0615384615384615,-0.0461538461538462,
-0.0307692307692308,-0.0153846153846154,0.),(-1.,1.),.UNSPECIFIED.)
GEOMETRIC_REPRESENTATION_ITEM()
RATIONAL_B_SPLINE_SURFACE(((1.,1.),(1.,1.),(1.,1.),(1.,1.),(1.,1.),(1.,
1.),(1.,1.),(1.,1.),(1.,1.),(1.,1.),(1.,1.),(1.,1.),(1.,1.),(1.,1.),(1.,
1.),(1.,1.),(1.,1.),(1.,1.),(1.,1.),(1.,1.),(1.,1.),(1.,1.),(1.,1.),(1.,
1.),(1.,1.),(1.,1.),(1.,1.),(1.,1.),(1.,1.),(1.,1.),(1.,1.),(1.,1.),(1.,
1.),(1.,1.),(1.,1.),(1.,1.),(1.,1.),(1.,1.),(1.,1.),(1.,1.),(1.,1.),(1.,
1.),(1.,1.),(1.,1.),(1.,1.),(1.,1.),(1.,1.),(1.,1.),(1.,1.),(1.,1.),(1.,
1.),(1.,1.),(1.,1.),(1.,1.),(1.,1.),(1.,1.),(1.,1.),(1.,1.),(1.,1.),(1.,
1.),(1.,1.),(1.,1.),(1.,1.),(1.,1.),(1.,1.),(1.,1.),(1.,1.),(1.,1.),(1.,
1.),(1.,1.)))
REPRESENTATION_ITEM('')
SURFACE()
);
#35=(
BOUNDED_SURFACE()
B_SPLINE_SURFACE(5,1,((#34916,#34917),(#34918,#34919),(#34920,#34921),(#34922,
#34923),(#34924,#34925),(#34926,#34927),(#34928,#34929),(#34930,#34931),
(#34932,#34933),(#34934,#34935),(#34936,#34937),(#34938,#34939),(#34940,
#34941),(#34942,#34943),(#34944,#34945),(#34946,#34947),(#34948,#34949),
(#34950,#34951),(#34952,#34953),(#34954,#34955),(#34956,#34957),(#34958,
#34959),(#34960,#34961),(#34962,#34963),(#34964,#34965),(#34966,#34967),
(#34968,#34969),(#34970,#34971),(#34972,#34973),(#34974,#34975),(#34976,
#34977),(#34978,#34979),(#34980,#34981),(#34982,#34983),(#34984,#34985),
(#34986,#34987),(#34988,#34989),(#34990,#34991),(#34992,#34993),(#34994,
#34995),(#34996,#34997),(#34998,#34999),(#35000,#35001),(#35002,#35003),
(#35004,#35005),(#35006,#35007),(#35008,#35009),(#35010,#35011),(#35012,
#35013),(#35014,#35015),(#35016,#35017),(#35018,#35019),(#35020,#35021),
(#35022,#35023),(#35024,#35025),(#35026,#35027),(#35028,#35029),(#35030,
#35031),(#35032,#35033),(#35034,#35035),(#35036,#35037),(#35038,#35039),
(#35040,#35041),(#35042,#35043),(#35044,#35045),(#35046,#35047),(#35048,
#35049),(#35050,#35051),(#35052,#35053),(#35054,#35055)),.UNSPECIFIED.,
 .F.,.F.,.F.)
B_SPLINE_SURFACE_WITH_KNOTS((6,1,1,1,1,1,1,1,1,1,1,1,1,1,1,1,1,1,1,1,1,
1,1,1,1,1,1,1,1,1,1,1,1,1,1,1,1,1,1,1,1,1,1,1,1,1,1,1,1,1,1,1,1,1,1,1,1,
1,1,1,1,1,1,1,1,6),(2,2),(-1.,-0.984615384615383,-0.969230769230768,-0.953846153846152,
-0.938461538461537,-0.923076923076922,-0.907692307692306,-0.892307692307691,
-0.876923076923076,-0.86153846153846,-0.846153846153845,-0.83076923076923,
-0.815384615384614,-0.799999999999999,-0.784615384615384,-0.769230769230768,
-0.753846153846153,-0.738461538461538,-0.723076923076922,-0.707692307692307,
-0.692307692307692,-0.676923076923076,-0.661538461538461,-0.646153846153846,
-0.63076923076923,-0.615384615384615,-0.6,-0.584615384615384,-0.569230769230769,
-0.553846153846154,-0.538461538461538,-0.523076923076923,-0.507692307692308,
-0.492307692307692,-0.476923076923077,-0.461538461538462,-0.446153846153846,
-0.430769230769231,-0.415384615384615,-0.4,-0.384615384615385,-0.369230769230769,
-0.353846153846154,-0.338461538461538,-0.323076923076923,-0.307692307692308,
-0.292307692307692,-0.276923076923077,-0.261538461538462,-0.246153846153846,
-0.230769230769231,-0.215384615384615,-0.2,-0.184615384615385,-0.169230769230769,
-0.153846153846154,-0.138461538461538,-0.123076923076923,-0.107692307692308,
-0.0923076923076923,-0.0769230769230769,-0.0615384615384615,-0.0461538461538462,
-0.0307692307692308,-0.0153846153846154,0.),(-1.,1.),.UNSPECIFIED.)
GEOMETRIC_REPRESENTATION_ITEM()
RATIONAL_B_SPLINE_SURFACE(((1.,1.),(1.,1.),(1.,1.),(1.,1.),(1.,1.),(1.,
1.),(1.,1.),(1.,1.),(1.,1.),(1.,1.),(1.,1.),(1.,1.),(1.,1.),(1.,1.),(1.,
1.),(1.,1.),(1.,1.),(1.,1.),(1.,1.),(1.,1.),(1.,1.),(1.,1.),(1.,1.),(1.,
1.),(1.,1.),(1.,1.),(1.,1.),(1.,1.),(1.,1.),(1.,1.),(1.,1.),(1.,1.),(1.,
1.),(1.,1.),(1.,1.),(1.,1.),(1.,1.),(1.,1.),(1.,1.),(1.,1.),(1.,1.),(1.,
1.),(1.,1.),(1.,1.),(1.,1.),(1.,1.),(1.,1.),(1.,1.),(1.,1.),(1.,1.),(1.,
1.),(1.,1.),(1.,1.),(1.,1.),(1.,1.),(1.,1.),(1.,1.),(1.,1.),(1.,1.),(1.,
1.),(1.,1.),(1.,1.),(1.,1.),(1.,1.),(1.,1.),(1.,1.),(1.,1.),(1.,1.),(1.,
1.),(1.,1.)))
REPRESENTATION_ITEM('')
SURFACE()
);
#36=(
BOUNDED_SURFACE()
B_SPLINE_SURFACE(5,1,((#35132,#35133),(#35134,#35135),(#35136,#35137),(#35138,
#35139),(#35140,#35141),(#35142,#35143),(#35144,#35145),(#35146,#35147),
(#35148,#35149),(#35150,#35151),(#35152,#35153),(#35154,#35155),(#35156,
#35157),(#35158,#35159),(#35160,#35161),(#35162,#35163),(#35164,#35165),
(#35166,#35167),(#35168,#35169),(#35170,#35171),(#35172,#35173),(#35174,
#35175),(#35176,#35177),(#35178,#35179),(#35180,#35181),(#35182,#35183),
(#35184,#35185),(#35186,#35187),(#35188,#35189),(#35190,#35191),(#35192,
#35193),(#35194,#35195),(#35196,#35197),(#35198,#35199),(#35200,#35201),
(#35202,#35203),(#35204,#35205),(#35206,#35207),(#35208,#35209),(#35210,
#35211),(#35212,#35213),(#35214,#35215),(#35216,#35217),(#35218,#35219),
(#35220,#35221),(#35222,#35223),(#35224,#35225),(#35226,#35227),(#35228,
#35229),(#35230,#35231),(#35232,#35233),(#35234,#35235),(#35236,#35237),
(#35238,#35239),(#35240,#35241),(#35242,#35243),(#35244,#35245),(#35246,
#35247),(#35248,#35249),(#35250,#35251),(#35252,#35253),(#35254,#35255),
(#35256,#35257),(#35258,#35259),(#35260,#35261),(#35262,#35263),(#35264,
#35265),(#35266,#35267),(#35268,#35269),(#35270,#35271)),.UNSPECIFIED.,
 .F.,.F.,.F.)
B_SPLINE_SURFACE_WITH_KNOTS((6,1,1,1,1,1,1,1,1,1,1,1,1,1,1,1,1,1,1,1,1,
1,1,1,1,1,1,1,1,1,1,1,1,1,1,1,1,1,1,1,1,1,1,1,1,1,1,1,1,1,1,1,1,1,1,1,1,
1,1,1,1,1,1,1,1,6),(2,2),(-1.,-0.984615384615383,-0.969230769230768,-0.953846153846152,
-0.938461538461537,-0.923076923076922,-0.907692307692306,-0.892307692307691,
-0.876923076923076,-0.86153846153846,-0.846153846153845,-0.83076923076923,
-0.815384615384614,-0.799999999999999,-0.784615384615384,-0.769230769230768,
-0.753846153846153,-0.738461538461538,-0.723076923076922,-0.707692307692307,
-0.692307692307692,-0.676923076923076,-0.661538461538461,-0.646153846153846,
-0.63076923076923,-0.615384615384615,-0.6,-0.584615384615384,-0.569230769230769,
-0.553846153846154,-0.538461538461538,-0.523076923076923,-0.507692307692308,
-0.492307692307692,-0.476923076923077,-0.461538461538462,-0.446153846153846,
-0.430769230769231,-0.415384615384615,-0.4,-0.384615384615385,-0.369230769230769,
-0.353846153846154,-0.338461538461538,-0.323076923076923,-0.307692307692308,
-0.292307692307692,-0.276923076923077,-0.261538461538462,-0.246153846153846,
-0.230769230769231,-0.215384615384615,-0.2,-0.184615384615385,-0.169230769230769,
-0.153846153846154,-0.138461538461538,-0.123076923076923,-0.107692307692308,
-0.0923076923076923,-0.0769230769230769,-0.0615384615384615,-0.0461538461538462,
-0.0307692307692308,-0.0153846153846154,0.),(-1.,1.),.UNSPECIFIED.)
GEOMETRIC_REPRESENTATION_ITEM()
RATIONAL_B_SPLINE_SURFACE(((1.,1.),(1.,1.),(1.,1.),(1.,1.),(1.,1.),(1.,
1.),(1.,1.),(1.,1.),(1.,1.),(1.,1.),(1.,1.),(1.,1.),(1.,1.),(1.,1.),(1.,
1.),(1.,1.),(1.,1.),(1.,1.),(1.,1.),(1.,1.),(1.,1.),(1.,1.),(1.,1.),(1.,
1.),(1.,1.),(1.,1.),(1.,1.),(1.,1.),(1.,1.),(1.,1.),(1.,1.),(1.,1.),(1.,
1.),(1.,1.),(1.,1.),(1.,1.),(1.,1.),(1.,1.),(1.,1.),(1.,1.),(1.,1.),(1.,
1.),(1.,1.),(1.,1.),(1.,1.),(1.,1.),(1.,1.),(1.,1.),(1.,1.),(1.,1.),(1.,
1.),(1.,1.),(1.,1.),(1.,1.),(1.,1.),(1.,1.),(1.,1.),(1.,1.),(1.,1.),(1.,
1.),(1.,1.),(1.,1.),(1.,1.),(1.,1.),(1.,1.),(1.,1.),(1.,1.),(1.,1.),(1.,
1.),(1.,1.)))
REPRESENTATION_ITEM('')
SURFACE()
);
#37=(
BOUNDED_SURFACE()
B_SPLINE_SURFACE(5,1,((#35348,#35349),(#35350,#35351),(#35352,#35353),(#35354,
#35355),(#35356,#35357),(#35358,#35359),(#35360,#35361),(#35362,#35363),
(#35364,#35365),(#35366,#35367),(#35368,#35369),(#35370,#35371),(#35372,
#35373),(#35374,#35375),(#35376,#35377),(#35378,#35379),(#35380,#35381),
(#35382,#35383),(#35384,#35385),(#35386,#35387),(#35388,#35389),(#35390,
#35391),(#35392,#35393),(#35394,#35395),(#35396,#35397),(#35398,#35399),
(#35400,#35401),(#35402,#35403),(#35404,#35405),(#35406,#35407),(#35408,
#35409),(#35410,#35411),(#35412,#35413),(#35414,#35415),(#35416,#35417),
(#35418,#35419),(#35420,#35421),(#35422,#35423),(#35424,#35425),(#35426,
#35427),(#35428,#35429),(#35430,#35431),(#35432,#35433),(#35434,#35435),
(#35436,#35437),(#35438,#35439),(#35440,#35441),(#35442,#35443),(#35444,
#35445),(#35446,#35447),(#35448,#35449),(#35450,#35451),(#35452,#35453),
(#35454,#35455),(#35456,#35457),(#35458,#35459),(#35460,#35461),(#35462,
#35463),(#35464,#35465),(#35466,#35467),(#35468,#35469),(#35470,#35471),
(#35472,#35473),(#35474,#35475),(#35476,#35477),(#35478,#35479),(#35480,
#35481),(#35482,#35483),(#35484,#35485),(#35486,#35487)),.UNSPECIFIED.,
 .F.,.F.,.F.)
B_SPLINE_SURFACE_WITH_KNOTS((6,1,1,1,1,1,1,1,1,1,1,1,1,1,1,1,1,1,1,1,1,
1,1,1,1,1,1,1,1,1,1,1,1,1,1,1,1,1,1,1,1,1,1,1,1,1,1,1,1,1,1,1,1,1,1,1,1,
1,1,1,1,1,1,1,1,6),(2,2),(-1.,-0.984615384615383,-0.969230769230768,-0.953846153846152,
-0.938461538461537,-0.923076923076922,-0.907692307692306,-0.892307692307691,
-0.876923076923076,-0.86153846153846,-0.846153846153845,-0.83076923076923,
-0.815384615384614,-0.799999999999999,-0.784615384615384,-0.769230769230768,
-0.753846153846153,-0.738461538461538,-0.723076923076922,-0.707692307692307,
-0.692307692307692,-0.676923076923076,-0.661538461538461,-0.646153846153846,
-0.63076923076923,-0.615384615384615,-0.6,-0.584615384615384,-0.569230769230769,
-0.553846153846154,-0.538461538461538,-0.523076923076923,-0.507692307692308,
-0.492307692307692,-0.476923076923077,-0.461538461538462,-0.446153846153846,
-0.430769230769231,-0.415384615384615,-0.4,-0.384615384615385,-0.369230769230769,
-0.353846153846154,-0.338461538461538,-0.323076923076923,-0.307692307692308,
-0.292307692307692,-0.276923076923077,-0.261538461538462,-0.246153846153846,
-0.230769230769231,-0.215384615384615,-0.2,-0.184615384615385,-0.169230769230769,
-0.153846153846154,-0.138461538461538,-0.123076923076923,-0.107692307692308,
-0.0923076923076923,-0.0769230769230769,-0.0615384615384615,-0.0461538461538462,
-0.0307692307692308,-0.0153846153846154,0.),(-1.,1.),.UNSPECIFIED.)
GEOMETRIC_REPRESENTATION_ITEM()
RATIONAL_B_SPLINE_SURFACE(((1.,1.),(1.,1.),(1.,1.),(1.,1.),(1.,1.),(1.,
1.),(1.,1.),(1.,1.),(1.,1.),(1.,1.),(1.,1.),(1.,1.),(1.,1.),(1.,1.),(1.,
1.),(1.,1.),(1.,1.),(1.,1.),(1.,1.),(1.,1.),(1.,1.),(1.,1.),(1.,1.),(1.,
1.),(1.,1.),(1.,1.),(1.,1.),(1.,1.),(1.,1.),(1.,1.),(1.,1.),(1.,1.),(1.,
1.),(1.,1.),(1.,1.),(1.,1.),(1.,1.),(1.,1.),(1.,1.),(1.,1.),(1.,1.),(1.,
1.),(1.,1.),(1.,1.),(1.,1.),(1.,1.),(1.,1.),(1.,1.),(1.,1.),(1.,1.),(1.,
1.),(1.,1.),(1.,1.),(1.,1.),(1.,1.),(1.,1.),(1.,1.),(1.,1.),(1.,1.),(1.,
1.),(1.,1.),(1.,1.),(1.,1.),(1.,1.),(1.,1.),(1.,1.),(1.,1.),(1.,1.),(1.,
1.),(1.,1.)))
REPRESENTATION_ITEM('')
SURFACE()
);
#38=(
BOUNDED_SURFACE()
B_SPLINE_SURFACE(5,1,((#35564,#35565),(#35566,#35567),(#35568,#35569),(#35570,
#35571),(#35572,#35573),(#35574,#35575),(#35576,#35577),(#35578,#35579),
(#35580,#35581),(#35582,#35583),(#35584,#35585),(#35586,#35587),(#35588,
#35589),(#35590,#35591),(#35592,#35593),(#35594,#35595),(#35596,#35597),
(#35598,#35599),(#35600,#35601),(#35602,#35603),(#35604,#35605),(#35606,
#35607),(#35608,#35609),(#35610,#35611),(#35612,#35613),(#35614,#35615),
(#35616,#35617),(#35618,#35619),(#35620,#35621),(#35622,#35623),(#35624,
#35625),(#35626,#35627),(#35628,#35629),(#35630,#35631),(#35632,#35633),
(#35634,#35635),(#35636,#35637),(#35638,#35639),(#35640,#35641),(#35642,
#35643),(#35644,#35645),(#35646,#35647),(#35648,#35649),(#35650,#35651),
(#35652,#35653),(#35654,#35655),(#35656,#35657),(#35658,#35659),(#35660,
#35661),(#35662,#35663),(#35664,#35665),(#35666,#35667),(#35668,#35669),
(#35670,#35671),(#35672,#35673),(#35674,#35675),(#35676,#35677),(#35678,
#35679),(#35680,#35681),(#35682,#35683),(#35684,#35685),(#35686,#35687),
(#35688,#35689),(#35690,#35691),(#35692,#35693),(#35694,#35695),(#35696,
#35697),(#35698,#35699),(#35700,#35701),(#35702,#35703)),.UNSPECIFIED.,
 .F.,.F.,.F.)
B_SPLINE_SURFACE_WITH_KNOTS((6,1,1,1,1,1,1,1,1,1,1,1,1,1,1,1,1,1,1,1,1,
1,1,1,1,1,1,1,1,1,1,1,1,1,1,1,1,1,1,1,1,1,1,1,1,1,1,1,1,1,1,1,1,1,1,1,1,
1,1,1,1,1,1,1,1,6),(2,2),(-1.,-0.984615384615383,-0.969230769230768,-0.953846153846152,
-0.938461538461537,-0.923076923076922,-0.907692307692306,-0.892307692307691,
-0.876923076923076,-0.86153846153846,-0.846153846153845,-0.83076923076923,
-0.815384615384614,-0.799999999999999,-0.784615384615384,-0.769230769230768,
-0.753846153846153,-0.738461538461538,-0.723076923076922,-0.707692307692307,
-0.692307692307692,-0.676923076923076,-0.661538461538461,-0.646153846153846,
-0.63076923076923,-0.615384615384615,-0.6,-0.584615384615384,-0.569230769230769,
-0.553846153846154,-0.538461538461538,-0.523076923076923,-0.507692307692308,
-0.492307692307692,-0.476923076923077,-0.461538461538462,-0.446153846153846,
-0.430769230769231,-0.415384615384615,-0.4,-0.384615384615385,-0.369230769230769,
-0.353846153846154,-0.338461538461538,-0.323076923076923,-0.307692307692308,
-0.292307692307692,-0.276923076923077,-0.261538461538462,-0.246153846153846,
-0.230769230769231,-0.215384615384615,-0.2,-0.184615384615385,-0.169230769230769,
-0.153846153846154,-0.138461538461538,-0.123076923076923,-0.107692307692308,
-0.0923076923076923,-0.0769230769230769,-0.0615384615384615,-0.0461538461538462,
-0.0307692307692308,-0.0153846153846154,0.),(-1.,1.),.UNSPECIFIED.)
GEOMETRIC_REPRESENTATION_ITEM()
RATIONAL_B_SPLINE_SURFACE(((1.,1.),(1.,1.),(1.,1.),(1.,1.),(1.,1.),(1.,
1.),(1.,1.),(1.,1.),(1.,1.),(1.,1.),(1.,1.),(1.,1.),(1.,1.),(1.,1.),(1.,
1.),(1.,1.),(1.,1.),(1.,1.),(1.,1.),(1.,1.),(1.,1.),(1.,1.),(1.,1.),(1.,
1.),(1.,1.),(1.,1.),(1.,1.),(1.,1.),(1.,1.),(1.,1.),(1.,1.),(1.,1.),(1.,
1.),(1.,1.),(1.,1.),(1.,1.),(1.,1.),(1.,1.),(1.,1.),(1.,1.),(1.,1.),(1.,
1.),(1.,1.),(1.,1.),(1.,1.),(1.,1.),(1.,1.),(1.,1.),(1.,1.),(1.,1.),(1.,
1.),(1.,1.),(1.,1.),(1.,1.),(1.,1.),(1.,1.),(1.,1.),(1.,1.),(1.,1.),(1.,
1.),(1.,1.),(1.,1.),(1.,1.),(1.,1.),(1.,1.),(1.,1.),(1.,1.),(1.,1.),(1.,
1.),(1.,1.)))
REPRESENTATION_ITEM('')
SURFACE()
);
#39=(
BOUNDED_SURFACE()
B_SPLINE_SURFACE(5,1,((#35780,#35781),(#35782,#35783),(#35784,#35785),(#35786,
#35787),(#35788,#35789),(#35790,#35791),(#35792,#35793),(#35794,#35795),
(#35796,#35797),(#35798,#35799),(#35800,#35801),(#35802,#35803),(#35804,
#35805),(#35806,#35807),(#35808,#35809),(#35810,#35811),(#35812,#35813),
(#35814,#35815),(#35816,#35817),(#35818,#35819),(#35820,#35821),(#35822,
#35823),(#35824,#35825),(#35826,#35827),(#35828,#35829),(#35830,#35831),
(#35832,#35833),(#35834,#35835),(#35836,#35837),(#35838,#35839),(#35840,
#35841),(#35842,#35843),(#35844,#35845),(#35846,#35847),(#35848,#35849),
(#35850,#35851),(#35852,#35853),(#35854,#35855),(#35856,#35857),(#35858,
#35859),(#35860,#35861),(#35862,#35863),(#35864,#35865),(#35866,#35867),
(#35868,#35869),(#35870,#35871),(#35872,#35873),(#35874,#35875),(#35876,
#35877),(#35878,#35879),(#35880,#35881),(#35882,#35883),(#35884,#35885),
(#35886,#35887),(#35888,#35889),(#35890,#35891),(#35892,#35893),(#35894,
#35895),(#35896,#35897),(#35898,#35899),(#35900,#35901),(#35902,#35903),
(#35904,#35905),(#35906,#35907),(#35908,#35909),(#35910,#35911),(#35912,
#35913),(#35914,#35915),(#35916,#35917),(#35918,#35919)),.UNSPECIFIED.,
 .F.,.F.,.F.)
B_SPLINE_SURFACE_WITH_KNOTS((6,1,1,1,1,1,1,1,1,1,1,1,1,1,1,1,1,1,1,1,1,
1,1,1,1,1,1,1,1,1,1,1,1,1,1,1,1,1,1,1,1,1,1,1,1,1,1,1,1,1,1,1,1,1,1,1,1,
1,1,1,1,1,1,1,1,6),(2,2),(-1.,-0.984615384615383,-0.969230769230768,-0.953846153846152,
-0.938461538461537,-0.923076923076922,-0.907692307692306,-0.892307692307691,
-0.876923076923076,-0.86153846153846,-0.846153846153845,-0.83076923076923,
-0.815384615384614,-0.799999999999999,-0.784615384615384,-0.769230769230768,
-0.753846153846153,-0.738461538461538,-0.723076923076922,-0.707692307692307,
-0.692307692307692,-0.676923076923076,-0.661538461538461,-0.646153846153846,
-0.63076923076923,-0.615384615384615,-0.6,-0.584615384615384,-0.569230769230769,
-0.553846153846154,-0.538461538461538,-0.523076923076923,-0.507692307692308,
-0.492307692307692,-0.476923076923077,-0.461538461538462,-0.446153846153846,
-0.430769230769231,-0.415384615384615,-0.4,-0.384615384615385,-0.369230769230769,
-0.353846153846154,-0.338461538461538,-0.323076923076923,-0.307692307692308,
-0.292307692307692,-0.276923076923077,-0.261538461538462,-0.246153846153846,
-0.230769230769231,-0.215384615384615,-0.2,-0.184615384615385,-0.169230769230769,
-0.153846153846154,-0.138461538461538,-0.123076923076923,-0.107692307692308,
-0.0923076923076923,-0.0769230769230769,-0.0615384615384615,-0.0461538461538462,
-0.0307692307692308,-0.0153846153846154,0.),(-1.,1.),.UNSPECIFIED.)
GEOMETRIC_REPRESENTATION_ITEM()
RATIONAL_B_SPLINE_SURFACE(((1.,1.),(1.,1.),(1.,1.),(1.,1.),(1.,1.),(1.,
1.),(1.,1.),(1.,1.),(1.,1.),(1.,1.),(1.,1.),(1.,1.),(1.,1.),(1.,1.),(1.,
1.),(1.,1.),(1.,1.),(1.,1.),(1.,1.),(1.,1.),(1.,1.),(1.,1.),(1.,1.),(1.,
1.),(1.,1.),(1.,1.),(1.,1.),(1.,1.),(1.,1.),(1.,1.),(1.,1.),(1.,1.),(1.,
1.),(1.,1.),(1.,1.),(1.,1.),(1.,1.),(1.,1.),(1.,1.),(1.,1.),(1.,1.),(1.,
1.),(1.,1.),(1.,1.),(1.,1.),(1.,1.),(1.,1.),(1.,1.),(1.,1.),(1.,1.),(1.,
1.),(1.,1.),(1.,1.),(1.,1.),(1.,1.),(1.,1.),(1.,1.),(1.,1.),(1.,1.),(1.,
1.),(1.,1.),(1.,1.),(1.,1.),(1.,1.),(1.,1.),(1.,1.),(1.,1.),(1.,1.),(1.,
1.),(1.,1.)))
REPRESENTATION_ITEM('')
SURFACE()
);
#40=(
BOUNDED_SURFACE()
B_SPLINE_SURFACE(5,1,((#35996,#35997),(#35998,#35999),(#36000,#36001),(#36002,
#36003),(#36004,#36005),(#36006,#36007),(#36008,#36009),(#36010,#36011),
(#36012,#36013),(#36014,#36015),(#36016,#36017),(#36018,#36019),(#36020,
#36021),(#36022,#36023),(#36024,#36025),(#36026,#36027),(#36028,#36029),
(#36030,#36031),(#36032,#36033),(#36034,#36035),(#36036,#36037),(#36038,
#36039),(#36040,#36041),(#36042,#36043),(#36044,#36045),(#36046,#36047),
(#36048,#36049),(#36050,#36051),(#36052,#36053),(#36054,#36055),(#36056,
#36057),(#36058,#36059),(#36060,#36061),(#36062,#36063),(#36064,#36065),
(#36066,#36067),(#36068,#36069),(#36070,#36071),(#36072,#36073),(#36074,
#36075),(#36076,#36077),(#36078,#36079),(#36080,#36081),(#36082,#36083),
(#36084,#36085),(#36086,#36087),(#36088,#36089),(#36090,#36091),(#36092,
#36093),(#36094,#36095),(#36096,#36097),(#36098,#36099),(#36100,#36101),
(#36102,#36103),(#36104,#36105),(#36106,#36107),(#36108,#36109),(#36110,
#36111),(#36112,#36113),(#36114,#36115),(#36116,#36117),(#36118,#36119),
(#36120,#36121),(#36122,#36123),(#36124,#36125),(#36126,#36127),(#36128,
#36129),(#36130,#36131),(#36132,#36133),(#36134,#36135)),.UNSPECIFIED.,
 .F.,.F.,.F.)
B_SPLINE_SURFACE_WITH_KNOTS((6,1,1,1,1,1,1,1,1,1,1,1,1,1,1,1,1,1,1,1,1,
1,1,1,1,1,1,1,1,1,1,1,1,1,1,1,1,1,1,1,1,1,1,1,1,1,1,1,1,1,1,1,1,1,1,1,1,
1,1,1,1,1,1,1,1,6),(2,2),(-1.,-0.984615384615383,-0.969230769230768,-0.953846153846152,
-0.938461538461537,-0.923076923076922,-0.907692307692306,-0.892307692307691,
-0.876923076923076,-0.86153846153846,-0.846153846153845,-0.83076923076923,
-0.815384615384614,-0.799999999999999,-0.784615384615384,-0.769230769230768,
-0.753846153846153,-0.738461538461538,-0.723076923076922,-0.707692307692307,
-0.692307692307692,-0.676923076923076,-0.661538461538461,-0.646153846153846,
-0.63076923076923,-0.615384615384615,-0.6,-0.584615384615384,-0.569230769230769,
-0.553846153846154,-0.538461538461538,-0.523076923076923,-0.507692307692308,
-0.492307692307692,-0.476923076923077,-0.461538461538462,-0.446153846153846,
-0.430769230769231,-0.415384615384615,-0.4,-0.384615384615385,-0.369230769230769,
-0.353846153846154,-0.338461538461538,-0.323076923076923,-0.307692307692308,
-0.292307692307692,-0.276923076923077,-0.261538461538462,-0.246153846153846,
-0.230769230769231,-0.215384615384615,-0.2,-0.184615384615385,-0.169230769230769,
-0.153846153846154,-0.138461538461538,-0.123076923076923,-0.107692307692308,
-0.0923076923076923,-0.0769230769230769,-0.0615384615384615,-0.0461538461538462,
-0.0307692307692308,-0.0153846153846154,0.),(-1.,1.),.UNSPECIFIED.)
GEOMETRIC_REPRESENTATION_ITEM()
RATIONAL_B_SPLINE_SURFACE(((1.,1.),(1.,1.),(1.,1.),(1.,1.),(1.,1.),(1.,
1.),(1.,1.),(1.,1.),(1.,1.),(1.,1.),(1.,1.),(1.,1.),(1.,1.),(1.,1.),(1.,
1.),(1.,1.),(1.,1.),(1.,1.),(1.,1.),(1.,1.),(1.,1.),(1.,1.),(1.,1.),(1.,
1.),(1.,1.),(1.,1.),(1.,1.),(1.,1.),(1.,1.),(1.,1.),(1.,1.),(1.,1.),(1.,
1.),(1.,1.),(1.,1.),(1.,1.),(1.,1.),(1.,1.),(1.,1.),(1.,1.),(1.,1.),(1.,
1.),(1.,1.),(1.,1.),(1.,1.),(1.,1.),(1.,1.),(1.,1.),(1.,1.),(1.,1.),(1.,
1.),(1.,1.),(1.,1.),(1.,1.),(1.,1.),(1.,1.),(1.,1.),(1.,1.),(1.,1.),(1.,
1.),(1.,1.),(1.,1.),(1.,1.),(1.,1.),(1.,1.),(1.,1.),(1.,1.),(1.,1.),(1.,
1.),(1.,1.)))
REPRESENTATION_ITEM('')
SURFACE()
);
#41=(
BOUNDED_SURFACE()
B_SPLINE_SURFACE(5,1,((#36212,#36213),(#36214,#36215),(#36216,#36217),(#36218,
#36219),(#36220,#36221),(#36222,#36223),(#36224,#36225),(#36226,#36227),
(#36228,#36229),(#36230,#36231),(#36232,#36233),(#36234,#36235),(#36236,
#36237),(#36238,#36239),(#36240,#36241),(#36242,#36243),(#36244,#36245),
(#36246,#36247),(#36248,#36249),(#36250,#36251),(#36252,#36253),(#36254,
#36255),(#36256,#36257),(#36258,#36259),(#36260,#36261),(#36262,#36263),
(#36264,#36265),(#36266,#36267),(#36268,#36269),(#36270,#36271),(#36272,
#36273),(#36274,#36275),(#36276,#36277),(#36278,#36279),(#36280,#36281),
(#36282,#36283),(#36284,#36285),(#36286,#36287),(#36288,#36289),(#36290,
#36291),(#36292,#36293),(#36294,#36295),(#36296,#36297),(#36298,#36299),
(#36300,#36301),(#36302,#36303),(#36304,#36305),(#36306,#36307),(#36308,
#36309),(#36310,#36311),(#36312,#36313),(#36314,#36315),(#36316,#36317),
(#36318,#36319),(#36320,#36321),(#36322,#36323),(#36324,#36325),(#36326,
#36327),(#36328,#36329),(#36330,#36331),(#36332,#36333),(#36334,#36335),
(#36336,#36337),(#36338,#36339),(#36340,#36341),(#36342,#36343),(#36344,
#36345),(#36346,#36347),(#36348,#36349),(#36350,#36351)),.UNSPECIFIED.,
 .F.,.F.,.F.)
B_SPLINE_SURFACE_WITH_KNOTS((6,1,1,1,1,1,1,1,1,1,1,1,1,1,1,1,1,1,1,1,1,
1,1,1,1,1,1,1,1,1,1,1,1,1,1,1,1,1,1,1,1,1,1,1,1,1,1,1,1,1,1,1,1,1,1,1,1,
1,1,1,1,1,1,1,1,6),(2,2),(-1.,-0.984615384615383,-0.969230769230768,-0.953846153846152,
-0.938461538461537,-0.923076923076922,-0.907692307692306,-0.892307692307691,
-0.876923076923076,-0.86153846153846,-0.846153846153845,-0.83076923076923,
-0.815384615384614,-0.799999999999999,-0.784615384615384,-0.769230769230768,
-0.753846153846153,-0.738461538461538,-0.723076923076922,-0.707692307692307,
-0.692307692307692,-0.676923076923076,-0.661538461538461,-0.646153846153846,
-0.63076923076923,-0.615384615384615,-0.6,-0.584615384615384,-0.569230769230769,
-0.553846153846154,-0.538461538461538,-0.523076923076923,-0.507692307692308,
-0.492307692307692,-0.476923076923077,-0.461538461538462,-0.446153846153846,
-0.430769230769231,-0.415384615384615,-0.4,-0.384615384615385,-0.369230769230769,
-0.353846153846154,-0.338461538461538,-0.323076923076923,-0.307692307692308,
-0.292307692307692,-0.276923076923077,-0.261538461538462,-0.246153846153846,
-0.230769230769231,-0.215384615384615,-0.2,-0.184615384615385,-0.169230769230769,
-0.153846153846154,-0.138461538461538,-0.123076923076923,-0.107692307692308,
-0.0923076923076923,-0.0769230769230769,-0.0615384615384615,-0.0461538461538462,
-0.0307692307692308,-0.0153846153846154,0.),(-1.,1.),.UNSPECIFIED.)
GEOMETRIC_REPRESENTATION_ITEM()
RATIONAL_B_SPLINE_SURFACE(((1.,1.),(1.,1.),(1.,1.),(1.,1.),(1.,1.),(1.,
1.),(1.,1.),(1.,1.),(1.,1.),(1.,1.),(1.,1.),(1.,1.),(1.,1.),(1.,1.),(1.,
1.),(1.,1.),(1.,1.),(1.,1.),(1.,1.),(1.,1.),(1.,1.),(1.,1.),(1.,1.),(1.,
1.),(1.,1.),(1.,1.),(1.,1.),(1.,1.),(1.,1.),(1.,1.),(1.,1.),(1.,1.),(1.,
1.),(1.,1.),(1.,1.),(1.,1.),(1.,1.),(1.,1.),(1.,1.),(1.,1.),(1.,1.),(1.,
1.),(1.,1.),(1.,1.),(1.,1.),(1.,1.),(1.,1.),(1.,1.),(1.,1.),(1.,1.),(1.,
1.),(1.,1.),(1.,1.),(1.,1.),(1.,1.),(1.,1.),(1.,1.),(1.,1.),(1.,1.),(1.,
1.),(1.,1.),(1.,1.),(1.,1.),(1.,1.),(1.,1.),(1.,1.),(1.,1.),(1.,1.),(1.,
1.),(1.,1.)))
REPRESENTATION_ITEM('')
SURFACE()
);
#42=(
BOUNDED_SURFACE()
B_SPLINE_SURFACE(5,1,((#36428,#36429),(#36430,#36431),(#36432,#36433),(#36434,
#36435),(#36436,#36437),(#36438,#36439),(#36440,#36441),(#36442,#36443),
(#36444,#36445),(#36446,#36447),(#36448,#36449),(#36450,#36451),(#36452,
#36453),(#36454,#36455),(#36456,#36457),(#36458,#36459),(#36460,#36461),
(#36462,#36463),(#36464,#36465),(#36466,#36467),(#36468,#36469),(#36470,
#36471),(#36472,#36473),(#36474,#36475),(#36476,#36477),(#36478,#36479),
(#36480,#36481),(#36482,#36483),(#36484,#36485),(#36486,#36487),(#36488,
#36489),(#36490,#36491),(#36492,#36493),(#36494,#36495),(#36496,#36497),
(#36498,#36499),(#36500,#36501),(#36502,#36503),(#36504,#36505),(#36506,
#36507),(#36508,#36509),(#36510,#36511),(#36512,#36513),(#36514,#36515),
(#36516,#36517),(#36518,#36519),(#36520,#36521),(#36522,#36523),(#36524,
#36525),(#36526,#36527),(#36528,#36529),(#36530,#36531),(#36532,#36533),
(#36534,#36535),(#36536,#36537),(#36538,#36539),(#36540,#36541),(#36542,
#36543),(#36544,#36545),(#36546,#36547),(#36548,#36549),(#36550,#36551),
(#36552,#36553),(#36554,#36555),(#36556,#36557),(#36558,#36559),(#36560,
#36561),(#36562,#36563),(#36564,#36565),(#36566,#36567)),.UNSPECIFIED.,
 .F.,.F.,.F.)
B_SPLINE_SURFACE_WITH_KNOTS((6,1,1,1,1,1,1,1,1,1,1,1,1,1,1,1,1,1,1,1,1,
1,1,1,1,1,1,1,1,1,1,1,1,1,1,1,1,1,1,1,1,1,1,1,1,1,1,1,1,1,1,1,1,1,1,1,1,
1,1,1,1,1,1,1,1,6),(2,2),(-1.,-0.984615384615383,-0.969230769230768,-0.953846153846152,
-0.938461538461537,-0.923076923076922,-0.907692307692306,-0.892307692307691,
-0.876923076923076,-0.86153846153846,-0.846153846153845,-0.83076923076923,
-0.815384615384614,-0.799999999999999,-0.784615384615384,-0.769230769230768,
-0.753846153846153,-0.738461538461538,-0.723076923076922,-0.707692307692307,
-0.692307692307692,-0.676923076923076,-0.661538461538461,-0.646153846153846,
-0.63076923076923,-0.615384615384615,-0.6,-0.584615384615384,-0.569230769230769,
-0.553846153846154,-0.538461538461538,-0.523076923076923,-0.507692307692308,
-0.492307692307692,-0.476923076923077,-0.461538461538462,-0.446153846153846,
-0.430769230769231,-0.415384615384615,-0.4,-0.384615384615385,-0.369230769230769,
-0.353846153846154,-0.338461538461538,-0.323076923076923,-0.307692307692308,
-0.292307692307692,-0.276923076923077,-0.261538461538462,-0.246153846153846,
-0.230769230769231,-0.215384615384615,-0.2,-0.184615384615385,-0.169230769230769,
-0.153846153846154,-0.138461538461538,-0.123076923076923,-0.107692307692308,
-0.0923076923076923,-0.0769230769230769,-0.0615384615384615,-0.0461538461538462,
-0.0307692307692308,-0.0153846153846154,0.),(-1.,1.),.UNSPECIFIED.)
GEOMETRIC_REPRESENTATION_ITEM()
RATIONAL_B_SPLINE_SURFACE(((1.,1.),(1.,1.),(1.,1.),(1.,1.),(1.,1.),(1.,
1.),(1.,1.),(1.,1.),(1.,1.),(1.,1.),(1.,1.),(1.,1.),(1.,1.),(1.,1.),(1.,
1.),(1.,1.),(1.,1.),(1.,1.),(1.,1.),(1.,1.),(1.,1.),(1.,1.),(1.,1.),(1.,
1.),(1.,1.),(1.,1.),(1.,1.),(1.,1.),(1.,1.),(1.,1.),(1.,1.),(1.,1.),(1.,
1.),(1.,1.),(1.,1.),(1.,1.),(1.,1.),(1.,1.),(1.,1.),(1.,1.),(1.,1.),(1.,
1.),(1.,1.),(1.,1.),(1.,1.),(1.,1.),(1.,1.),(1.,1.),(1.,1.),(1.,1.),(1.,
1.),(1.,1.),(1.,1.),(1.,1.),(1.,1.),(1.,1.),(1.,1.),(1.,1.),(1.,1.),(1.,
1.),(1.,1.),(1.,1.),(1.,1.),(1.,1.),(1.,1.),(1.,1.),(1.,1.),(1.,1.),(1.,
1.),(1.,1.)))
REPRESENTATION_ITEM('')
SURFACE()
);
#43=(
BOUNDED_SURFACE()
B_SPLINE_SURFACE(5,1,((#36644,#36645),(#36646,#36647),(#36648,#36649),(#36650,
#36651),(#36652,#36653),(#36654,#36655),(#36656,#36657),(#36658,#36659),
(#36660,#36661),(#36662,#36663),(#36664,#36665),(#36666,#36667),(#36668,
#36669),(#36670,#36671),(#36672,#36673),(#36674,#36675),(#36676,#36677),
(#36678,#36679),(#36680,#36681),(#36682,#36683),(#36684,#36685),(#36686,
#36687),(#36688,#36689),(#36690,#36691),(#36692,#36693),(#36694,#36695),
(#36696,#36697),(#36698,#36699),(#36700,#36701),(#36702,#36703),(#36704,
#36705),(#36706,#36707),(#36708,#36709),(#36710,#36711),(#36712,#36713),
(#36714,#36715),(#36716,#36717),(#36718,#36719),(#36720,#36721),(#36722,
#36723),(#36724,#36725),(#36726,#36727),(#36728,#36729),(#36730,#36731),
(#36732,#36733),(#36734,#36735),(#36736,#36737),(#36738,#36739),(#36740,
#36741),(#36742,#36743),(#36744,#36745),(#36746,#36747),(#36748,#36749),
(#36750,#36751),(#36752,#36753),(#36754,#36755),(#36756,#36757),(#36758,
#36759),(#36760,#36761),(#36762,#36763),(#36764,#36765),(#36766,#36767),
(#36768,#36769),(#36770,#36771),(#36772,#36773),(#36774,#36775),(#36776,
#36777),(#36778,#36779),(#36780,#36781),(#36782,#36783)),.UNSPECIFIED.,
 .F.,.F.,.F.)
B_SPLINE_SURFACE_WITH_KNOTS((6,1,1,1,1,1,1,1,1,1,1,1,1,1,1,1,1,1,1,1,1,
1,1,1,1,1,1,1,1,1,1,1,1,1,1,1,1,1,1,1,1,1,1,1,1,1,1,1,1,1,1,1,1,1,1,1,1,
1,1,1,1,1,1,1,1,6),(2,2),(-1.,-0.984615384615383,-0.969230769230768,-0.953846153846152,
-0.938461538461537,-0.923076923076922,-0.907692307692306,-0.892307692307691,
-0.876923076923076,-0.86153846153846,-0.846153846153845,-0.83076923076923,
-0.815384615384614,-0.799999999999999,-0.784615384615384,-0.769230769230768,
-0.753846153846153,-0.738461538461538,-0.723076923076922,-0.707692307692307,
-0.692307692307692,-0.676923076923076,-0.661538461538461,-0.646153846153846,
-0.63076923076923,-0.615384615384615,-0.6,-0.584615384615384,-0.569230769230769,
-0.553846153846154,-0.538461538461538,-0.523076923076923,-0.507692307692308,
-0.492307692307692,-0.476923076923077,-0.461538461538462,-0.446153846153846,
-0.430769230769231,-0.415384615384615,-0.4,-0.384615384615385,-0.369230769230769,
-0.353846153846154,-0.338461538461538,-0.323076923076923,-0.307692307692308,
-0.292307692307692,-0.276923076923077,-0.261538461538462,-0.246153846153846,
-0.230769230769231,-0.215384615384615,-0.2,-0.184615384615385,-0.169230769230769,
-0.153846153846154,-0.138461538461538,-0.123076923076923,-0.107692307692308,
-0.0923076923076923,-0.0769230769230769,-0.0615384615384615,-0.0461538461538462,
-0.0307692307692308,-0.0153846153846154,0.),(-1.,1.),.UNSPECIFIED.)
GEOMETRIC_REPRESENTATION_ITEM()
RATIONAL_B_SPLINE_SURFACE(((1.,1.),(1.,1.),(1.,1.),(1.,1.),(1.,1.),(1.,
1.),(1.,1.),(1.,1.),(1.,1.),(1.,1.),(1.,1.),(1.,1.),(1.,1.),(1.,1.),(1.,
1.),(1.,1.),(1.,1.),(1.,1.),(1.,1.),(1.,1.),(1.,1.),(1.,1.),(1.,1.),(1.,
1.),(1.,1.),(1.,1.),(1.,1.),(1.,1.),(1.,1.),(1.,1.),(1.,1.),(1.,1.),(1.,
1.),(1.,1.),(1.,1.),(1.,1.),(1.,1.),(1.,1.),(1.,1.),(1.,1.),(1.,1.),(1.,
1.),(1.,1.),(1.,1.),(1.,1.),(1.,1.),(1.,1.),(1.,1.),(1.,1.),(1.,1.),(1.,
1.),(1.,1.),(1.,1.),(1.,1.),(1.,1.),(1.,1.),(1.,1.),(1.,1.),(1.,1.),(1.,
1.),(1.,1.),(1.,1.),(1.,1.),(1.,1.),(1.,1.),(1.,1.),(1.,1.),(1.,1.),(1.,
1.),(1.,1.)))
REPRESENTATION_ITEM('')
SURFACE()
);
#44=(
BOUNDED_SURFACE()
B_SPLINE_SURFACE(5,1,((#36860,#36861),(#36862,#36863),(#36864,#36865),(#36866,
#36867),(#36868,#36869),(#36870,#36871),(#36872,#36873),(#36874,#36875),
(#36876,#36877),(#36878,#36879),(#36880,#36881),(#36882,#36883),(#36884,
#36885),(#36886,#36887),(#36888,#36889),(#36890,#36891),(#36892,#36893),
(#36894,#36895),(#36896,#36897),(#36898,#36899),(#36900,#36901),(#36902,
#36903),(#36904,#36905),(#36906,#36907),(#36908,#36909),(#36910,#36911),
(#36912,#36913),(#36914,#36915),(#36916,#36917),(#36918,#36919),(#36920,
#36921),(#36922,#36923),(#36924,#36925),(#36926,#36927),(#36928,#36929),
(#36930,#36931),(#36932,#36933),(#36934,#36935),(#36936,#36937),(#36938,
#36939),(#36940,#36941),(#36942,#36943),(#36944,#36945),(#36946,#36947),
(#36948,#36949),(#36950,#36951),(#36952,#36953),(#36954,#36955),(#36956,
#36957),(#36958,#36959),(#36960,#36961),(#36962,#36963),(#36964,#36965),
(#36966,#36967),(#36968,#36969),(#36970,#36971),(#36972,#36973),(#36974,
#36975),(#36976,#36977),(#36978,#36979),(#36980,#36981),(#36982,#36983),
(#36984,#36985),(#36986,#36987),(#36988,#36989),(#36990,#36991),(#36992,
#36993),(#36994,#36995),(#36996,#36997),(#36998,#36999)),.UNSPECIFIED.,
 .F.,.F.,.F.)
B_SPLINE_SURFACE_WITH_KNOTS((6,1,1,1,1,1,1,1,1,1,1,1,1,1,1,1,1,1,1,1,1,
1,1,1,1,1,1,1,1,1,1,1,1,1,1,1,1,1,1,1,1,1,1,1,1,1,1,1,1,1,1,1,1,1,1,1,1,
1,1,1,1,1,1,1,1,6),(2,2),(-1.,-0.984615384615383,-0.969230769230768,-0.953846153846152,
-0.938461538461537,-0.923076923076922,-0.907692307692306,-0.892307692307691,
-0.876923076923076,-0.86153846153846,-0.846153846153845,-0.83076923076923,
-0.815384615384614,-0.799999999999999,-0.784615384615384,-0.769230769230768,
-0.753846153846153,-0.738461538461538,-0.723076923076922,-0.707692307692307,
-0.692307692307692,-0.676923076923076,-0.661538461538461,-0.646153846153846,
-0.63076923076923,-0.615384615384615,-0.6,-0.584615384615384,-0.569230769230769,
-0.553846153846154,-0.538461538461538,-0.523076923076923,-0.507692307692308,
-0.492307692307692,-0.476923076923077,-0.461538461538462,-0.446153846153846,
-0.430769230769231,-0.415384615384615,-0.4,-0.384615384615385,-0.369230769230769,
-0.353846153846154,-0.338461538461538,-0.323076923076923,-0.307692307692308,
-0.292307692307692,-0.276923076923077,-0.261538461538462,-0.246153846153846,
-0.230769230769231,-0.215384615384615,-0.2,-0.184615384615385,-0.169230769230769,
-0.153846153846154,-0.138461538461538,-0.123076923076923,-0.107692307692308,
-0.0923076923076923,-0.0769230769230769,-0.0615384615384615,-0.0461538461538462,
-0.0307692307692308,-0.0153846153846154,0.),(-1.,1.),.UNSPECIFIED.)
GEOMETRIC_REPRESENTATION_ITEM()
RATIONAL_B_SPLINE_SURFACE(((1.,1.),(1.,1.),(1.,1.),(1.,1.),(1.,1.),(1.,
1.),(1.,1.),(1.,1.),(1.,1.),(1.,1.),(1.,1.),(1.,1.),(1.,1.),(1.,1.),(1.,
1.),(1.,1.),(1.,1.),(1.,1.),(1.,1.),(1.,1.),(1.,1.),(1.,1.),(1.,1.),(1.,
1.),(1.,1.),(1.,1.),(1.,1.),(1.,1.),(1.,1.),(1.,1.),(1.,1.),(1.,1.),(1.,
1.),(1.,1.),(1.,1.),(1.,1.),(1.,1.),(1.,1.),(1.,1.),(1.,1.),(1.,1.),(1.,
1.),(1.,1.),(1.,1.),(1.,1.),(1.,1.),(1.,1.),(1.,1.),(1.,1.),(1.,1.),(1.,
1.),(1.,1.),(1.,1.),(1.,1.),(1.,1.),(1.,1.),(1.,1.),(1.,1.),(1.,1.),(1.,
1.),(1.,1.),(1.,1.),(1.,1.),(1.,1.),(1.,1.),(1.,1.),(1.,1.),(1.,1.),(1.,
1.),(1.,1.)))
REPRESENTATION_ITEM('')
SURFACE()
);
#45=(
BOUNDED_SURFACE()
B_SPLINE_SURFACE(5,1,((#37076,#37077),(#37078,#37079),(#37080,#37081),(#37082,
#37083),(#37084,#37085),(#37086,#37087),(#37088,#37089),(#37090,#37091),
(#37092,#37093),(#37094,#37095),(#37096,#37097),(#37098,#37099),(#37100,
#37101),(#37102,#37103),(#37104,#37105),(#37106,#37107),(#37108,#37109),
(#37110,#37111),(#37112,#37113),(#37114,#37115),(#37116,#37117),(#37118,
#37119),(#37120,#37121),(#37122,#37123),(#37124,#37125),(#37126,#37127),
(#37128,#37129),(#37130,#37131),(#37132,#37133),(#37134,#37135),(#37136,
#37137),(#37138,#37139),(#37140,#37141),(#37142,#37143),(#37144,#37145),
(#37146,#37147),(#37148,#37149),(#37150,#37151),(#37152,#37153),(#37154,
#37155),(#37156,#37157),(#37158,#37159),(#37160,#37161),(#37162,#37163),
(#37164,#37165),(#37166,#37167),(#37168,#37169),(#37170,#37171),(#37172,
#37173),(#37174,#37175),(#37176,#37177),(#37178,#37179),(#37180,#37181),
(#37182,#37183),(#37184,#37185),(#37186,#37187),(#37188,#37189),(#37190,
#37191),(#37192,#37193),(#37194,#37195),(#37196,#37197),(#37198,#37199),
(#37200,#37201),(#37202,#37203),(#37204,#37205),(#37206,#37207),(#37208,
#37209),(#37210,#37211),(#37212,#37213),(#37214,#37215)),.UNSPECIFIED.,
 .F.,.F.,.F.)
B_SPLINE_SURFACE_WITH_KNOTS((6,1,1,1,1,1,1,1,1,1,1,1,1,1,1,1,1,1,1,1,1,
1,1,1,1,1,1,1,1,1,1,1,1,1,1,1,1,1,1,1,1,1,1,1,1,1,1,1,1,1,1,1,1,1,1,1,1,
1,1,1,1,1,1,1,1,6),(2,2),(-1.,-0.984615384615383,-0.969230769230768,-0.953846153846152,
-0.938461538461537,-0.923076923076922,-0.907692307692306,-0.892307692307691,
-0.876923076923076,-0.86153846153846,-0.846153846153845,-0.83076923076923,
-0.815384615384614,-0.799999999999999,-0.784615384615384,-0.769230769230768,
-0.753846153846153,-0.738461538461538,-0.723076923076922,-0.707692307692307,
-0.692307692307692,-0.676923076923076,-0.661538461538461,-0.646153846153846,
-0.63076923076923,-0.615384615384615,-0.6,-0.584615384615384,-0.569230769230769,
-0.553846153846154,-0.538461538461538,-0.523076923076923,-0.507692307692308,
-0.492307692307692,-0.476923076923077,-0.461538461538462,-0.446153846153846,
-0.430769230769231,-0.415384615384615,-0.4,-0.384615384615385,-0.369230769230769,
-0.353846153846154,-0.338461538461538,-0.323076923076923,-0.307692307692308,
-0.292307692307692,-0.276923076923077,-0.261538461538462,-0.246153846153846,
-0.230769230769231,-0.215384615384615,-0.2,-0.184615384615385,-0.169230769230769,
-0.153846153846154,-0.138461538461538,-0.123076923076923,-0.107692307692308,
-0.0923076923076923,-0.0769230769230769,-0.0615384615384615,-0.0461538461538462,
-0.0307692307692308,-0.0153846153846154,0.),(-1.,1.),.UNSPECIFIED.)
GEOMETRIC_REPRESENTATION_ITEM()
RATIONAL_B_SPLINE_SURFACE(((1.,1.),(1.,1.),(1.,1.),(1.,1.),(1.,1.),(1.,
1.),(1.,1.),(1.,1.),(1.,1.),(1.,1.),(1.,1.),(1.,1.),(1.,1.),(1.,1.),(1.,
1.),(1.,1.),(1.,1.),(1.,1.),(1.,1.),(1.,1.),(1.,1.),(1.,1.),(1.,1.),(1.,
1.),(1.,1.),(1.,1.),(1.,1.),(1.,1.),(1.,1.),(1.,1.),(1.,1.),(1.,1.),(1.,
1.),(1.,1.),(1.,1.),(1.,1.),(1.,1.),(1.,1.),(1.,1.),(1.,1.),(1.,1.),(1.,
1.),(1.,1.),(1.,1.),(1.,1.),(1.,1.),(1.,1.),(1.,1.),(1.,1.),(1.,1.),(1.,
1.),(1.,1.),(1.,1.),(1.,1.),(1.,1.),(1.,1.),(1.,1.),(1.,1.),(1.,1.),(1.,
1.),(1.,1.),(1.,1.),(1.,1.),(1.,1.),(1.,1.),(1.,1.),(1.,1.),(1.,1.),(1.,
1.),(1.,1.)))
REPRESENTATION_ITEM('')
SURFACE()
);
#46=(
BOUNDED_SURFACE()
B_SPLINE_SURFACE(5,1,((#37292,#37293),(#37294,#37295),(#37296,#37297),(#37298,
#37299),(#37300,#37301),(#37302,#37303),(#37304,#37305),(#37306,#37307),
(#37308,#37309),(#37310,#37311),(#37312,#37313),(#37314,#37315),(#37316,
#37317),(#37318,#37319),(#37320,#37321),(#37322,#37323),(#37324,#37325),
(#37326,#37327),(#37328,#37329),(#37330,#37331),(#37332,#37333),(#37334,
#37335),(#37336,#37337),(#37338,#37339),(#37340,#37341),(#37342,#37343),
(#37344,#37345),(#37346,#37347),(#37348,#37349),(#37350,#37351),(#37352,
#37353),(#37354,#37355),(#37356,#37357),(#37358,#37359),(#37360,#37361),
(#37362,#37363),(#37364,#37365),(#37366,#37367),(#37368,#37369),(#37370,
#37371),(#37372,#37373),(#37374,#37375),(#37376,#37377),(#37378,#37379),
(#37380,#37381),(#37382,#37383),(#37384,#37385),(#37386,#37387),(#37388,
#37389),(#37390,#37391),(#37392,#37393),(#37394,#37395),(#37396,#37397),
(#37398,#37399),(#37400,#37401),(#37402,#37403),(#37404,#37405),(#37406,
#37407),(#37408,#37409),(#37410,#37411),(#37412,#37413),(#37414,#37415),
(#37416,#37417),(#37418,#37419),(#37420,#37421),(#37422,#37423),(#37424,
#37425),(#37426,#37427),(#37428,#37429),(#37430,#37431)),.UNSPECIFIED.,
 .F.,.F.,.F.)
B_SPLINE_SURFACE_WITH_KNOTS((6,1,1,1,1,1,1,1,1,1,1,1,1,1,1,1,1,1,1,1,1,
1,1,1,1,1,1,1,1,1,1,1,1,1,1,1,1,1,1,1,1,1,1,1,1,1,1,1,1,1,1,1,1,1,1,1,1,
1,1,1,1,1,1,1,1,6),(2,2),(-1.,-0.984615384615383,-0.969230769230768,-0.953846153846152,
-0.938461538461537,-0.923076923076922,-0.907692307692306,-0.892307692307691,
-0.876923076923076,-0.86153846153846,-0.846153846153845,-0.83076923076923,
-0.815384615384614,-0.799999999999999,-0.784615384615384,-0.769230769230768,
-0.753846153846153,-0.738461538461538,-0.723076923076922,-0.707692307692307,
-0.692307692307692,-0.676923076923076,-0.661538461538461,-0.646153846153846,
-0.63076923076923,-0.615384615384615,-0.6,-0.584615384615384,-0.569230769230769,
-0.553846153846154,-0.538461538461538,-0.523076923076923,-0.507692307692308,
-0.492307692307692,-0.476923076923077,-0.461538461538462,-0.446153846153846,
-0.430769230769231,-0.415384615384615,-0.4,-0.384615384615385,-0.369230769230769,
-0.353846153846154,-0.338461538461538,-0.323076923076923,-0.307692307692308,
-0.292307692307692,-0.276923076923077,-0.261538461538462,-0.246153846153846,
-0.230769230769231,-0.215384615384615,-0.2,-0.184615384615385,-0.169230769230769,
-0.153846153846154,-0.138461538461538,-0.123076923076923,-0.107692307692308,
-0.0923076923076923,-0.0769230769230769,-0.0615384615384615,-0.0461538461538462,
-0.0307692307692308,-0.0153846153846154,0.),(-1.,1.),.UNSPECIFIED.)
GEOMETRIC_REPRESENTATION_ITEM()
RATIONAL_B_SPLINE_SURFACE(((1.,1.),(1.,1.),(1.,1.),(1.,1.),(1.,1.),(1.,
1.),(1.,1.),(1.,1.),(1.,1.),(1.,1.),(1.,1.),(1.,1.),(1.,1.),(1.,1.),(1.,
1.),(1.,1.),(1.,1.),(1.,1.),(1.,1.),(1.,1.),(1.,1.),(1.,1.),(1.,1.),(1.,
1.),(1.,1.),(1.,1.),(1.,1.),(1.,1.),(1.,1.),(1.,1.),(1.,1.),(1.,1.),(1.,
1.),(1.,1.),(1.,1.),(1.,1.),(1.,1.),(1.,1.),(1.,1.),(1.,1.),(1.,1.),(1.,
1.),(1.,1.),(1.,1.),(1.,1.),(1.,1.),(1.,1.),(1.,1.),(1.,1.),(1.,1.),(1.,
1.),(1.,1.),(1.,1.),(1.,1.),(1.,1.),(1.,1.),(1.,1.),(1.,1.),(1.,1.),(1.,
1.),(1.,1.),(1.,1.),(1.,1.),(1.,1.),(1.,1.),(1.,1.),(1.,1.),(1.,1.),(1.,
1.),(1.,1.)))
REPRESENTATION_ITEM('')
SURFACE()
);
#47=(
BOUNDED_SURFACE()
B_SPLINE_SURFACE(5,1,((#37508,#37509),(#37510,#37511),(#37512,#37513),(#37514,
#37515),(#37516,#37517),(#37518,#37519),(#37520,#37521),(#37522,#37523),
(#37524,#37525),(#37526,#37527),(#37528,#37529),(#37530,#37531),(#37532,
#37533),(#37534,#37535),(#37536,#37537),(#37538,#37539),(#37540,#37541),
(#37542,#37543),(#37544,#37545),(#37546,#37547),(#37548,#37549),(#37550,
#37551),(#37552,#37553),(#37554,#37555),(#37556,#37557),(#37558,#37559),
(#37560,#37561),(#37562,#37563),(#37564,#37565),(#37566,#37567),(#37568,
#37569),(#37570,#37571),(#37572,#37573),(#37574,#37575),(#37576,#37577),
(#37578,#37579),(#37580,#37581),(#37582,#37583),(#37584,#37585),(#37586,
#37587),(#37588,#37589),(#37590,#37591),(#37592,#37593),(#37594,#37595),
(#37596,#37597),(#37598,#37599),(#37600,#37601),(#37602,#37603),(#37604,
#37605),(#37606,#37607),(#37608,#37609),(#37610,#37611),(#37612,#37613),
(#37614,#37615),(#37616,#37617),(#37618,#37619),(#37620,#37621),(#37622,
#37623),(#37624,#37625),(#37626,#37627),(#37628,#37629),(#37630,#37631),
(#37632,#37633),(#37634,#37635),(#37636,#37637),(#37638,#37639),(#37640,
#37641),(#37642,#37643),(#37644,#37645),(#37646,#37647)),.UNSPECIFIED.,
 .F.,.F.,.F.)
B_SPLINE_SURFACE_WITH_KNOTS((6,1,1,1,1,1,1,1,1,1,1,1,1,1,1,1,1,1,1,1,1,
1,1,1,1,1,1,1,1,1,1,1,1,1,1,1,1,1,1,1,1,1,1,1,1,1,1,1,1,1,1,1,1,1,1,1,1,
1,1,1,1,1,1,1,1,6),(2,2),(-1.,-0.984615384615383,-0.969230769230768,-0.953846153846152,
-0.938461538461537,-0.923076923076922,-0.907692307692306,-0.892307692307691,
-0.876923076923076,-0.86153846153846,-0.846153846153845,-0.83076923076923,
-0.815384615384614,-0.799999999999999,-0.784615384615384,-0.769230769230768,
-0.753846153846153,-0.738461538461538,-0.723076923076922,-0.707692307692307,
-0.692307692307692,-0.676923076923076,-0.661538461538461,-0.646153846153846,
-0.63076923076923,-0.615384615384615,-0.6,-0.584615384615384,-0.569230769230769,
-0.553846153846154,-0.538461538461538,-0.523076923076923,-0.507692307692308,
-0.492307692307692,-0.476923076923077,-0.461538461538462,-0.446153846153846,
-0.430769230769231,-0.415384615384615,-0.4,-0.384615384615385,-0.369230769230769,
-0.353846153846154,-0.338461538461538,-0.323076923076923,-0.307692307692308,
-0.292307692307692,-0.276923076923077,-0.261538461538462,-0.246153846153846,
-0.230769230769231,-0.215384615384615,-0.2,-0.184615384615385,-0.169230769230769,
-0.153846153846154,-0.138461538461538,-0.123076923076923,-0.107692307692308,
-0.0923076923076923,-0.0769230769230769,-0.0615384615384615,-0.0461538461538462,
-0.0307692307692308,-0.0153846153846154,0.),(-1.,1.),.UNSPECIFIED.)
GEOMETRIC_REPRESENTATION_ITEM()
RATIONAL_B_SPLINE_SURFACE(((1.,1.),(1.,1.),(1.,1.),(1.,1.),(1.,1.),(1.,
1.),(1.,1.),(1.,1.),(1.,1.),(1.,1.),(1.,1.),(1.,1.),(1.,1.),(1.,1.),(1.,
1.),(1.,1.),(1.,1.),(1.,1.),(1.,1.),(1.,1.),(1.,1.),(1.,1.),(1.,1.),(1.,
1.),(1.,1.),(1.,1.),(1.,1.),(1.,1.),(1.,1.),(1.,1.),(1.,1.),(1.,1.),(1.,
1.),(1.,1.),(1.,1.),(1.,1.),(1.,1.),(1.,1.),(1.,1.),(1.,1.),(1.,1.),(1.,
1.),(1.,1.),(1.,1.),(1.,1.),(1.,1.),(1.,1.),(1.,1.),(1.,1.),(1.,1.),(1.,
1.),(1.,1.),(1.,1.),(1.,1.),(1.,1.),(1.,1.),(1.,1.),(1.,1.),(1.,1.),(1.,
1.),(1.,1.),(1.,1.),(1.,1.),(1.,1.),(1.,1.),(1.,1.),(1.,1.),(1.,1.),(1.,
1.),(1.,1.)))
REPRESENTATION_ITEM('')
SURFACE()
);
#48=(
BOUNDED_SURFACE()
B_SPLINE_SURFACE(5,1,((#37724,#37725),(#37726,#37727),(#37728,#37729),(#37730,
#37731),(#37732,#37733),(#37734,#37735),(#37736,#37737),(#37738,#37739),
(#37740,#37741),(#37742,#37743),(#37744,#37745),(#37746,#37747),(#37748,
#37749),(#37750,#37751),(#37752,#37753),(#37754,#37755),(#37756,#37757),
(#37758,#37759),(#37760,#37761),(#37762,#37763),(#37764,#37765),(#37766,
#37767),(#37768,#37769),(#37770,#37771),(#37772,#37773),(#37774,#37775),
(#37776,#37777),(#37778,#37779),(#37780,#37781),(#37782,#37783),(#37784,
#37785),(#37786,#37787),(#37788,#37789),(#37790,#37791),(#37792,#37793),
(#37794,#37795),(#37796,#37797),(#37798,#37799),(#37800,#37801),(#37802,
#37803),(#37804,#37805),(#37806,#37807),(#37808,#37809),(#37810,#37811),
(#37812,#37813),(#37814,#37815),(#37816,#37817),(#37818,#37819),(#37820,
#37821),(#37822,#37823),(#37824,#37825),(#37826,#37827),(#37828,#37829),
(#37830,#37831),(#37832,#37833),(#37834,#37835),(#37836,#37837),(#37838,
#37839),(#37840,#37841),(#37842,#37843),(#37844,#37845),(#37846,#37847),
(#37848,#37849),(#37850,#37851),(#37852,#37853),(#37854,#37855),(#37856,
#37857),(#37858,#37859),(#37860,#37861),(#37862,#37863)),.UNSPECIFIED.,
 .F.,.F.,.F.)
B_SPLINE_SURFACE_WITH_KNOTS((6,1,1,1,1,1,1,1,1,1,1,1,1,1,1,1,1,1,1,1,1,
1,1,1,1,1,1,1,1,1,1,1,1,1,1,1,1,1,1,1,1,1,1,1,1,1,1,1,1,1,1,1,1,1,1,1,1,
1,1,1,1,1,1,1,1,6),(2,2),(-1.,-0.984615384615383,-0.969230769230768,-0.953846153846152,
-0.938461538461537,-0.923076923076922,-0.907692307692306,-0.892307692307691,
-0.876923076923076,-0.86153846153846,-0.846153846153845,-0.83076923076923,
-0.815384615384614,-0.799999999999999,-0.784615384615384,-0.769230769230768,
-0.753846153846153,-0.738461538461538,-0.723076923076922,-0.707692307692307,
-0.692307692307692,-0.676923076923076,-0.661538461538461,-0.646153846153846,
-0.63076923076923,-0.615384615384615,-0.6,-0.584615384615384,-0.569230769230769,
-0.553846153846154,-0.538461538461538,-0.523076923076923,-0.507692307692308,
-0.492307692307692,-0.476923076923077,-0.461538461538462,-0.446153846153846,
-0.430769230769231,-0.415384615384615,-0.4,-0.384615384615385,-0.369230769230769,
-0.353846153846154,-0.338461538461538,-0.323076923076923,-0.307692307692308,
-0.292307692307692,-0.276923076923077,-0.261538461538462,-0.246153846153846,
-0.230769230769231,-0.215384615384615,-0.2,-0.184615384615385,-0.169230769230769,
-0.153846153846154,-0.138461538461538,-0.123076923076923,-0.107692307692308,
-0.0923076923076923,-0.0769230769230769,-0.0615384615384615,-0.0461538461538462,
-0.0307692307692308,-0.0153846153846154,0.),(-1.,1.),.UNSPECIFIED.)
GEOMETRIC_REPRESENTATION_ITEM()
RATIONAL_B_SPLINE_SURFACE(((1.,1.),(1.,1.),(1.,1.),(1.,1.),(1.,1.),(1.,
1.),(1.,1.),(1.,1.),(1.,1.),(1.,1.),(1.,1.),(1.,1.),(1.,1.),(1.,1.),(1.,
1.),(1.,1.),(1.,1.),(1.,1.),(1.,1.),(1.,1.),(1.,1.),(1.,1.),(1.,1.),(1.,
1.),(1.,1.),(1.,1.),(1.,1.),(1.,1.),(1.,1.),(1.,1.),(1.,1.),(1.,1.),(1.,
1.),(1.,1.),(1.,1.),(1.,1.),(1.,1.),(1.,1.),(1.,1.),(1.,1.),(1.,1.),(1.,
1.),(1.,1.),(1.,1.),(1.,1.),(1.,1.),(1.,1.),(1.,1.),(1.,1.),(1.,1.),(1.,
1.),(1.,1.),(1.,1.),(1.,1.),(1.,1.),(1.,1.),(1.,1.),(1.,1.),(1.,1.),(1.,
1.),(1.,1.),(1.,1.),(1.,1.),(1.,1.),(1.,1.),(1.,1.),(1.,1.),(1.,1.),(1.,
1.),(1.,1.)))
REPRESENTATION_ITEM('')
SURFACE()
);
#49=(
BOUNDED_SURFACE()
B_SPLINE_SURFACE(5,1,((#37940,#37941),(#37942,#37943),(#37944,#37945),(#37946,
#37947),(#37948,#37949),(#37950,#37951),(#37952,#37953),(#37954,#37955),
(#37956,#37957),(#37958,#37959),(#37960,#37961),(#37962,#37963),(#37964,
#37965),(#37966,#37967),(#37968,#37969),(#37970,#37971),(#37972,#37973),
(#37974,#37975),(#37976,#37977),(#37978,#37979),(#37980,#37981),(#37982,
#37983),(#37984,#37985),(#37986,#37987),(#37988,#37989),(#37990,#37991),
(#37992,#37993),(#37994,#37995),(#37996,#37997),(#37998,#37999),(#38000,
#38001),(#38002,#38003),(#38004,#38005),(#38006,#38007),(#38008,#38009),
(#38010,#38011),(#38012,#38013),(#38014,#38015),(#38016,#38017),(#38018,
#38019),(#38020,#38021),(#38022,#38023),(#38024,#38025),(#38026,#38027),
(#38028,#38029),(#38030,#38031),(#38032,#38033),(#38034,#38035),(#38036,
#38037),(#38038,#38039),(#38040,#38041),(#38042,#38043),(#38044,#38045),
(#38046,#38047),(#38048,#38049),(#38050,#38051),(#38052,#38053),(#38054,
#38055),(#38056,#38057),(#38058,#38059),(#38060,#38061),(#38062,#38063),
(#38064,#38065),(#38066,#38067),(#38068,#38069),(#38070,#38071),(#38072,
#38073),(#38074,#38075),(#38076,#38077),(#38078,#38079)),.UNSPECIFIED.,
 .F.,.F.,.F.)
B_SPLINE_SURFACE_WITH_KNOTS((6,1,1,1,1,1,1,1,1,1,1,1,1,1,1,1,1,1,1,1,1,
1,1,1,1,1,1,1,1,1,1,1,1,1,1,1,1,1,1,1,1,1,1,1,1,1,1,1,1,1,1,1,1,1,1,1,1,
1,1,1,1,1,1,1,1,6),(2,2),(-1.,-0.984615384615383,-0.969230769230768,-0.953846153846152,
-0.938461538461537,-0.923076923076922,-0.907692307692306,-0.892307692307691,
-0.876923076923076,-0.86153846153846,-0.846153846153845,-0.83076923076923,
-0.815384615384614,-0.799999999999999,-0.784615384615384,-0.769230769230768,
-0.753846153846153,-0.738461538461538,-0.723076923076922,-0.707692307692307,
-0.692307692307692,-0.676923076923076,-0.661538461538461,-0.646153846153846,
-0.63076923076923,-0.615384615384615,-0.6,-0.584615384615384,-0.569230769230769,
-0.553846153846154,-0.538461538461538,-0.523076923076923,-0.507692307692308,
-0.492307692307692,-0.476923076923077,-0.461538461538462,-0.446153846153846,
-0.430769230769231,-0.415384615384615,-0.4,-0.384615384615385,-0.369230769230769,
-0.353846153846154,-0.338461538461538,-0.323076923076923,-0.307692307692308,
-0.292307692307692,-0.276923076923077,-0.261538461538462,-0.246153846153846,
-0.230769230769231,-0.215384615384615,-0.2,-0.184615384615385,-0.169230769230769,
-0.153846153846154,-0.138461538461538,-0.123076923076923,-0.107692307692308,
-0.0923076923076923,-0.0769230769230769,-0.0615384615384615,-0.0461538461538462,
-0.0307692307692308,-0.0153846153846154,0.),(-1.,1.),.UNSPECIFIED.)
GEOMETRIC_REPRESENTATION_ITEM()
RATIONAL_B_SPLINE_SURFACE(((1.,1.),(1.,1.),(1.,1.),(1.,1.),(1.,1.),(1.,
1.),(1.,1.),(1.,1.),(1.,1.),(1.,1.),(1.,1.),(1.,1.),(1.,1.),(1.,1.),(1.,
1.),(1.,1.),(1.,1.),(1.,1.),(1.,1.),(1.,1.),(1.,1.),(1.,1.),(1.,1.),(1.,
1.),(1.,1.),(1.,1.),(1.,1.),(1.,1.),(1.,1.),(1.,1.),(1.,1.),(1.,1.),(1.,
1.),(1.,1.),(1.,1.),(1.,1.),(1.,1.),(1.,1.),(1.,1.),(1.,1.),(1.,1.),(1.,
1.),(1.,1.),(1.,1.),(1.,1.),(1.,1.),(1.,1.),(1.,1.),(1.,1.),(1.,1.),(1.,
1.),(1.,1.),(1.,1.),(1.,1.),(1.,1.),(1.,1.),(1.,1.),(1.,1.),(1.,1.),(1.,
1.),(1.,1.),(1.,1.),(1.,1.),(1.,1.),(1.,1.),(1.,1.),(1.,1.),(1.,1.),(1.,
1.),(1.,1.)))
REPRESENTATION_ITEM('')
SURFACE()
);
#50=(
BOUNDED_SURFACE()
B_SPLINE_SURFACE(5,1,((#38156,#38157),(#38158,#38159),(#38160,#38161),(#38162,
#38163),(#38164,#38165),(#38166,#38167),(#38168,#38169),(#38170,#38171),
(#38172,#38173),(#38174,#38175),(#38176,#38177),(#38178,#38179),(#38180,
#38181),(#38182,#38183),(#38184,#38185),(#38186,#38187),(#38188,#38189),
(#38190,#38191),(#38192,#38193),(#38194,#38195),(#38196,#38197),(#38198,
#38199),(#38200,#38201),(#38202,#38203),(#38204,#38205),(#38206,#38207),
(#38208,#38209),(#38210,#38211),(#38212,#38213),(#38214,#38215),(#38216,
#38217),(#38218,#38219),(#38220,#38221),(#38222,#38223),(#38224,#38225),
(#38226,#38227),(#38228,#38229),(#38230,#38231),(#38232,#38233),(#38234,
#38235),(#38236,#38237),(#38238,#38239),(#38240,#38241),(#38242,#38243),
(#38244,#38245),(#38246,#38247),(#38248,#38249),(#38250,#38251),(#38252,
#38253),(#38254,#38255),(#38256,#38257),(#38258,#38259),(#38260,#38261),
(#38262,#38263),(#38264,#38265),(#38266,#38267),(#38268,#38269),(#38270,
#38271),(#38272,#38273),(#38274,#38275),(#38276,#38277),(#38278,#38279),
(#38280,#38281),(#38282,#38283),(#38284,#38285),(#38286,#38287),(#38288,
#38289),(#38290,#38291),(#38292,#38293),(#38294,#38295)),.UNSPECIFIED.,
 .F.,.F.,.F.)
B_SPLINE_SURFACE_WITH_KNOTS((6,1,1,1,1,1,1,1,1,1,1,1,1,1,1,1,1,1,1,1,1,
1,1,1,1,1,1,1,1,1,1,1,1,1,1,1,1,1,1,1,1,1,1,1,1,1,1,1,1,1,1,1,1,1,1,1,1,
1,1,1,1,1,1,1,1,6),(2,2),(-1.,-0.984615384615383,-0.969230769230768,-0.953846153846152,
-0.938461538461537,-0.923076923076922,-0.907692307692306,-0.892307692307691,
-0.876923076923076,-0.86153846153846,-0.846153846153845,-0.83076923076923,
-0.815384615384614,-0.799999999999999,-0.784615384615384,-0.769230769230768,
-0.753846153846153,-0.738461538461538,-0.723076923076922,-0.707692307692307,
-0.692307692307692,-0.676923076923076,-0.661538461538461,-0.646153846153846,
-0.63076923076923,-0.615384615384615,-0.6,-0.584615384615384,-0.569230769230769,
-0.553846153846154,-0.538461538461538,-0.523076923076923,-0.507692307692308,
-0.492307692307692,-0.476923076923077,-0.461538461538462,-0.446153846153846,
-0.430769230769231,-0.415384615384615,-0.4,-0.384615384615385,-0.369230769230769,
-0.353846153846154,-0.338461538461538,-0.323076923076923,-0.307692307692308,
-0.292307692307692,-0.276923076923077,-0.261538461538462,-0.246153846153846,
-0.230769230769231,-0.215384615384615,-0.2,-0.184615384615385,-0.169230769230769,
-0.153846153846154,-0.138461538461538,-0.123076923076923,-0.107692307692308,
-0.0923076923076923,-0.0769230769230769,-0.0615384615384615,-0.0461538461538462,
-0.0307692307692308,-0.0153846153846154,0.),(-1.,1.),.UNSPECIFIED.)
GEOMETRIC_REPRESENTATION_ITEM()
RATIONAL_B_SPLINE_SURFACE(((1.,1.),(1.,1.),(1.,1.),(1.,1.),(1.,1.),(1.,
1.),(1.,1.),(1.,1.),(1.,1.),(1.,1.),(1.,1.),(1.,1.),(1.,1.),(1.,1.),(1.,
1.),(1.,1.),(1.,1.),(1.,1.),(1.,1.),(1.,1.),(1.,1.),(1.,1.),(1.,1.),(1.,
1.),(1.,1.),(1.,1.),(1.,1.),(1.,1.),(1.,1.),(1.,1.),(1.,1.),(1.,1.),(1.,
1.),(1.,1.),(1.,1.),(1.,1.),(1.,1.),(1.,1.),(1.,1.),(1.,1.),(1.,1.),(1.,
1.),(1.,1.),(1.,1.),(1.,1.),(1.,1.),(1.,1.),(1.,1.),(1.,1.),(1.,1.),(1.,
1.),(1.,1.),(1.,1.),(1.,1.),(1.,1.),(1.,1.),(1.,1.),(1.,1.),(1.,1.),(1.,
1.),(1.,1.),(1.,1.),(1.,1.),(1.,1.),(1.,1.),(1.,1.),(1.,1.),(1.,1.),(1.,
1.),(1.,1.)))
REPRESENTATION_ITEM('')
SURFACE()
);
#131=(
BOUNDED_CURVE()
B_SPLINE_CURVE(5,(#26804,#26805,#26806,#26807,#26808,#26809,#26810,#26811,
#26812,#26813,#26814,#26815,#26816,#26817,#26818,#26819,#26820,#26821,#26822,
#26823,#26824,#26825,#26826,#26827,#26828,#26829,#26830,#26831,#26832,#26833,
#26834,#26835,#26836,#26837,#26838,#26839,#26840,#26841,#26842,#26843,#26844,
#26845,#26846,#26847,#26848,#26849,#26850,#26851,#26852,#26853,#26854,#26855,
#26856,#26857,#26858,#26859,#26860,#26861,#26862,#26863,#26864,#26865,#26866,
#26867,#26868,#26869,#26870,#26871,#26872,#26873),.UNSPECIFIED.,.F.,.F.)
B_SPLINE_CURVE_WITH_KNOTS((6,1,1,1,1,1,1,1,1,1,1,1,1,1,1,1,1,1,1,1,1,1,
1,1,1,1,1,1,1,1,1,1,1,1,1,1,1,1,1,1,1,1,1,1,1,1,1,1,1,1,1,1,1,1,1,1,1,1,
1,1,1,1,1,1,1,6),(0.,0.0153846153846154,0.0307692307692308,0.0461538461538462,
0.0615384615384615,0.0769230769230769,0.0923076923076923,0.107692307692308,
0.123076923076923,0.138461538461538,0.153846153846154,0.169230769230769,
0.184615384615385,0.2,0.215384615384615,0.230769230769231,0.246153846153846,
0.261538461538462,0.276923076923077,0.292307692307692,0.307692307692308,
0.323076923076923,0.338461538461538,0.353846153846154,0.369230769230769,
0.384615384615385,0.4,0.415384615384615,0.430769230769231,0.446153846153846,
0.461538461538462,0.476923076923077,0.492307692307692,0.507692307692308,
0.523076923076923,0.538461538461538,0.553846153846154,0.569230769230769,
0.584615384615384,0.6,0.615384615384615,0.63076923076923,0.646153846153846,
0.661538461538461,0.676923076923076,0.692307692307692,0.707692307692307,
0.723076923076922,0.738461538461538,0.753846153846153,0.769230769230768,
0.784615384615384,0.799999999999999,0.815384615384614,0.83076923076923,
0.846153846153845,0.86153846153846,0.876923076923076,0.892307692307691,
0.907692307692306,0.923076923076922,0.938461538461537,0.953846153846152,
0.969230769230768,0.984615384615383,1.),.UNSPECIFIED.)
CURVE()
GEOMETRIC_REPRESENTATION_ITEM()
RATIONAL_B_SPLINE_CURVE((1.,1.,1.,1.,1.,1.,1.,1.,1.,1.,1.,1.,1.,1.,1.,1.,
1.,1.,1.,1.,1.,1.,1.,1.,1.,1.,1.,1.,1.,1.,1.,1.,1.,1.,1.,1.,1.,1.,1.,1.,
1.,1.,1.,1.,1.,1.,1.,1.,1.,1.,1.,1.,1.,1.,1.,1.,1.,1.,1.,1.,1.,1.,1.,1.,
1.,1.,1.,1.,1.,1.))
REPRESENTATION_ITEM('')
);
#132=(
BOUNDED_CURVE()
B_SPLINE_CURVE(5,(#26877,#26878,#26879,#26880,#26881,#26882,#26883,#26884,
#26885,#26886,#26887,#26888,#26889,#26890,#26891,#26892,#26893,#26894,#26895,
#26896,#26897,#26898,#26899,#26900,#26901,#26902,#26903,#26904,#26905,#26906,
#26907,#26908,#26909,#26910,#26911,#26912,#26913,#26914,#26915,#26916,#26917,
#26918,#26919,#26920,#26921,#26922,#26923,#26924,#26925,#26926,#26927,#26928,
#26929,#26930,#26931,#26932,#26933,#26934,#26935,#26936,#26937,#26938,#26939,
#26940,#26941,#26942,#26943,#26944,#26945,#26946),.UNSPECIFIED.,.F.,.F.)
B_SPLINE_CURVE_WITH_KNOTS((6,1,1,1,1,1,1,1,1,1,1,1,1,1,1,1,1,1,1,1,1,1,
1,1,1,1,1,1,1,1,1,1,1,1,1,1,1,1,1,1,1,1,1,1,1,1,1,1,1,1,1,1,1,1,1,1,1,1,
1,1,1,1,1,1,1,6),(0.,0.0153846153846154,0.0307692307692308,0.0461538461538462,
0.0615384615384615,0.0769230769230769,0.0923076923076923,0.107692307692308,
0.123076923076923,0.138461538461538,0.153846153846154,0.169230769230769,
0.184615384615385,0.2,0.215384615384615,0.230769230769231,0.246153846153846,
0.261538461538462,0.276923076923077,0.292307692307692,0.307692307692308,
0.323076923076923,0.338461538461538,0.353846153846154,0.369230769230769,
0.384615384615385,0.4,0.415384615384615,0.430769230769231,0.446153846153846,
0.461538461538462,0.476923076923077,0.492307692307692,0.507692307692308,
0.523076923076923,0.538461538461538,0.553846153846154,0.569230769230769,
0.584615384615384,0.6,0.615384615384615,0.63076923076923,0.646153846153846,
0.661538461538461,0.676923076923076,0.692307692307692,0.707692307692307,
0.723076923076922,0.738461538461538,0.753846153846153,0.769230769230768,
0.784615384615384,0.799999999999999,0.815384615384614,0.83076923076923,
0.846153846153845,0.86153846153846,0.876923076923076,0.892307692307691,
0.907692307692306,0.923076923076922,0.938461538461537,0.953846153846152,
0.969230769230768,0.984615384615383,1.),.UNSPECIFIED.)
CURVE()
GEOMETRIC_REPRESENTATION_ITEM()
RATIONAL_B_SPLINE_CURVE((1.,1.,1.,1.,1.,1.,1.,1.,1.,1.,1.,1.,1.,1.,1.,1.,
1.,1.,1.,1.,1.,1.,1.,1.,1.,1.,1.,1.,1.,1.,1.,1.,1.,1.,1.,1.,1.,1.,1.,1.,
1.,1.,1.,1.,1.,1.,1.,1.,1.,1.,1.,1.,1.,1.,1.,1.,1.,1.,1.,1.,1.,1.,1.,1.,
1.,1.,1.,1.,1.,1.))
REPRESENTATION_ITEM('')
);
#133=(
BOUNDED_CURVE()
B_SPLINE_CURVE(5,(#26950,#26951,#26952,#26953,#26954,#26955,#26956,#26957,
#26958,#26959,#26960,#26961,#26962,#26963,#26964,#26965,#26966,#26967,#26968,
#26969,#26970,#26971,#26972,#26973,#26974,#26975,#26976,#26977,#26978,#26979,
#26980,#26981,#26982,#26983,#26984,#26985,#26986,#26987,#26988,#26989,#26990,
#26991,#26992,#26993,#26994,#26995,#26996,#26997,#26998,#26999,#27000,#27001,
#27002,#27003,#27004,#27005,#27006,#27007,#27008,#27009,#27010,#27011,#27012,
#27013,#27014,#27015,#27016,#27017,#27018,#27019),.UNSPECIFIED.,.F.,.F.)
B_SPLINE_CURVE_WITH_KNOTS((6,1,1,1,1,1,1,1,1,1,1,1,1,1,1,1,1,1,1,1,1,1,
1,1,1,1,1,1,1,1,1,1,1,1,1,1,1,1,1,1,1,1,1,1,1,1,1,1,1,1,1,1,1,1,1,1,1,1,
1,1,1,1,1,1,1,6),(0.,0.0153846153846154,0.0307692307692308,0.0461538461538462,
0.0615384615384615,0.0769230769230769,0.0923076923076923,0.107692307692308,
0.123076923076923,0.138461538461538,0.153846153846154,0.169230769230769,
0.184615384615385,0.2,0.215384615384615,0.230769230769231,0.246153846153846,
0.261538461538462,0.276923076923077,0.292307692307692,0.307692307692308,
0.323076923076923,0.338461538461538,0.353846153846154,0.369230769230769,
0.384615384615385,0.4,0.415384615384615,0.430769230769231,0.446153846153846,
0.461538461538462,0.476923076923077,0.492307692307692,0.507692307692308,
0.523076923076923,0.538461538461538,0.553846153846154,0.569230769230769,
0.584615384615384,0.6,0.615384615384615,0.63076923076923,0.646153846153846,
0.661538461538461,0.676923076923076,0.692307692307692,0.707692307692307,
0.723076923076922,0.738461538461538,0.753846153846153,0.769230769230768,
0.784615384615384,0.799999999999999,0.815384615384614,0.83076923076923,
0.846153846153845,0.86153846153846,0.876923076923076,0.892307692307691,
0.907692307692306,0.923076923076922,0.938461538461537,0.953846153846152,
0.969230769230768,0.984615384615383,1.),.UNSPECIFIED.)
CURVE()
GEOMETRIC_REPRESENTATION_ITEM()
RATIONAL_B_SPLINE_CURVE((1.,1.,1.,1.,1.,1.,1.,1.,1.,1.,1.,1.,1.,1.,1.,1.,
1.,1.,1.,1.,1.,1.,1.,1.,1.,1.,1.,1.,1.,1.,1.,1.,1.,1.,1.,1.,1.,1.,1.,1.,
1.,1.,1.,1.,1.,1.,1.,1.,1.,1.,1.,1.,1.,1.,1.,1.,1.,1.,1.,1.,1.,1.,1.,1.,
1.,1.,1.,1.,1.,1.))
REPRESENTATION_ITEM('')
);
#134=(
BOUNDED_CURVE()
B_SPLINE_CURVE(5,(#27023,#27024,#27025,#27026,#27027,#27028,#27029,#27030,
#27031,#27032,#27033,#27034,#27035,#27036,#27037,#27038,#27039,#27040,#27041,
#27042,#27043,#27044,#27045,#27046,#27047,#27048,#27049,#27050,#27051,#27052,
#27053,#27054,#27055,#27056,#27057,#27058,#27059,#27060,#27061,#27062,#27063,
#27064,#27065,#27066,#27067,#27068,#27069,#27070,#27071,#27072,#27073,#27074,
#27075,#27076,#27077,#27078,#27079,#27080,#27081,#27082,#27083,#27084,#27085,
#27086,#27087,#27088,#27089,#27090,#27091,#27092),.UNSPECIFIED.,.F.,.F.)
B_SPLINE_CURVE_WITH_KNOTS((6,1,1,1,1,1,1,1,1,1,1,1,1,1,1,1,1,1,1,1,1,1,
1,1,1,1,1,1,1,1,1,1,1,1,1,1,1,1,1,1,1,1,1,1,1,1,1,1,1,1,1,1,1,1,1,1,1,1,
1,1,1,1,1,1,1,6),(0.,0.0153846153846154,0.0307692307692308,0.0461538461538462,
0.0615384615384615,0.0769230769230769,0.0923076923076923,0.107692307692308,
0.123076923076923,0.138461538461538,0.153846153846154,0.169230769230769,
0.184615384615385,0.2,0.215384615384615,0.230769230769231,0.246153846153846,
0.261538461538462,0.276923076923077,0.292307692307692,0.307692307692308,
0.323076923076923,0.338461538461538,0.353846153846154,0.369230769230769,
0.384615384615385,0.4,0.415384615384615,0.430769230769231,0.446153846153846,
0.461538461538462,0.476923076923077,0.492307692307692,0.507692307692308,
0.523076923076923,0.538461538461538,0.553846153846154,0.569230769230769,
0.584615384615384,0.6,0.615384615384615,0.63076923076923,0.646153846153846,
0.661538461538461,0.676923076923076,0.692307692307692,0.707692307692307,
0.723076923076922,0.738461538461538,0.753846153846153,0.769230769230768,
0.784615384615384,0.799999999999999,0.815384615384614,0.83076923076923,
0.846153846153845,0.86153846153846,0.876923076923076,0.892307692307691,
0.907692307692306,0.923076923076922,0.938461538461537,0.953846153846152,
0.969230769230768,0.984615384615383,1.),.UNSPECIFIED.)
CURVE()
GEOMETRIC_REPRESENTATION_ITEM()
RATIONAL_B_SPLINE_CURVE((1.,1.,1.,1.,1.,1.,1.,1.,1.,1.,1.,1.,1.,1.,1.,1.,
1.,1.,1.,1.,1.,1.,1.,1.,1.,1.,1.,1.,1.,1.,1.,1.,1.,1.,1.,1.,1.,1.,1.,1.,
1.,1.,1.,1.,1.,1.,1.,1.,1.,1.,1.,1.,1.,1.,1.,1.,1.,1.,1.,1.,1.,1.,1.,1.,
1.,1.,1.,1.,1.,1.))
REPRESENTATION_ITEM('')
);
#135=(
BOUNDED_CURVE()
B_SPLINE_CURVE(5,(#27096,#27097,#27098,#27099,#27100,#27101,#27102,#27103,
#27104,#27105,#27106,#27107,#27108,#27109,#27110,#27111,#27112,#27113,#27114,
#27115,#27116,#27117,#27118,#27119,#27120,#27121,#27122,#27123,#27124,#27125,
#27126,#27127,#27128,#27129,#27130,#27131,#27132,#27133,#27134,#27135,#27136,
#27137,#27138,#27139,#27140,#27141,#27142,#27143,#27144,#27145,#27146,#27147,
#27148,#27149,#27150,#27151,#27152,#27153,#27154,#27155,#27156,#27157,#27158,
#27159,#27160,#27161,#27162,#27163,#27164,#27165),.UNSPECIFIED.,.F.,.F.)
B_SPLINE_CURVE_WITH_KNOTS((6,1,1,1,1,1,1,1,1,1,1,1,1,1,1,1,1,1,1,1,1,1,
1,1,1,1,1,1,1,1,1,1,1,1,1,1,1,1,1,1,1,1,1,1,1,1,1,1,1,1,1,1,1,1,1,1,1,1,
1,1,1,1,1,1,1,6),(0.,0.0153846153846154,0.0307692307692308,0.0461538461538462,
0.0615384615384615,0.0769230769230769,0.0923076923076923,0.107692307692308,
0.123076923076923,0.138461538461538,0.153846153846154,0.169230769230769,
0.184615384615385,0.2,0.215384615384615,0.230769230769231,0.246153846153846,
0.261538461538462,0.276923076923077,0.292307692307692,0.307692307692308,
0.323076923076923,0.338461538461538,0.353846153846154,0.369230769230769,
0.384615384615385,0.4,0.415384615384615,0.430769230769231,0.446153846153846,
0.461538461538462,0.476923076923077,0.492307692307692,0.507692307692308,
0.523076923076923,0.538461538461538,0.553846153846154,0.569230769230769,
0.584615384615384,0.6,0.615384615384615,0.63076923076923,0.646153846153846,
0.661538461538461,0.676923076923076,0.692307692307692,0.707692307692307,
0.723076923076922,0.738461538461538,0.753846153846153,0.769230769230768,
0.784615384615384,0.799999999999999,0.815384615384614,0.83076923076923,
0.846153846153845,0.86153846153846,0.876923076923076,0.892307692307691,
0.907692307692306,0.923076923076922,0.938461538461537,0.953846153846152,
0.969230769230768,0.984615384615383,1.),.UNSPECIFIED.)
CURVE()
GEOMETRIC_REPRESENTATION_ITEM()
RATIONAL_B_SPLINE_CURVE((1.,1.,1.,1.,1.,1.,1.,1.,1.,1.,1.,1.,1.,1.,1.,1.,
1.,1.,1.,1.,1.,1.,1.,1.,1.,1.,1.,1.,1.,1.,1.,1.,1.,1.,1.,1.,1.,1.,1.,1.,
1.,1.,1.,1.,1.,1.,1.,1.,1.,1.,1.,1.,1.,1.,1.,1.,1.,1.,1.,1.,1.,1.,1.,1.,
1.,1.,1.,1.,1.,1.))
REPRESENTATION_ITEM('')
);
#136=(
BOUNDED_CURVE()
B_SPLINE_CURVE(5,(#27169,#27170,#27171,#27172,#27173,#27174,#27175,#27176,
#27177,#27178,#27179,#27180,#27181,#27182,#27183,#27184,#27185,#27186,#27187,
#27188,#27189,#27190,#27191,#27192,#27193,#27194,#27195,#27196,#27197,#27198,
#27199,#27200,#27201,#27202,#27203,#27204,#27205,#27206,#27207,#27208,#27209,
#27210,#27211,#27212,#27213,#27214,#27215,#27216,#27217,#27218,#27219,#27220,
#27221,#27222,#27223,#27224,#27225,#27226,#27227,#27228,#27229,#27230,#27231,
#27232,#27233,#27234,#27235,#27236,#27237,#27238),.UNSPECIFIED.,.F.,.F.)
B_SPLINE_CURVE_WITH_KNOTS((6,1,1,1,1,1,1,1,1,1,1,1,1,1,1,1,1,1,1,1,1,1,
1,1,1,1,1,1,1,1,1,1,1,1,1,1,1,1,1,1,1,1,1,1,1,1,1,1,1,1,1,1,1,1,1,1,1,1,
1,1,1,1,1,1,1,6),(0.,0.0153846153846154,0.0307692307692308,0.0461538461538462,
0.0615384615384615,0.0769230769230769,0.0923076923076923,0.107692307692308,
0.123076923076923,0.138461538461538,0.153846153846154,0.169230769230769,
0.184615384615385,0.2,0.215384615384615,0.230769230769231,0.246153846153846,
0.261538461538462,0.276923076923077,0.292307692307692,0.307692307692308,
0.323076923076923,0.338461538461538,0.353846153846154,0.369230769230769,
0.384615384615385,0.4,0.415384615384615,0.430769230769231,0.446153846153846,
0.461538461538462,0.476923076923077,0.492307692307692,0.507692307692308,
0.523076923076923,0.538461538461538,0.553846153846154,0.569230769230769,
0.584615384615384,0.6,0.615384615384615,0.63076923076923,0.646153846153846,
0.661538461538461,0.676923076923076,0.692307692307692,0.707692307692307,
0.723076923076922,0.738461538461538,0.753846153846153,0.769230769230768,
0.784615384615384,0.799999999999999,0.815384615384614,0.83076923076923,
0.846153846153845,0.86153846153846,0.876923076923076,0.892307692307691,
0.907692307692306,0.923076923076922,0.938461538461537,0.953846153846152,
0.969230769230768,0.984615384615383,1.),.UNSPECIFIED.)
CURVE()
GEOMETRIC_REPRESENTATION_ITEM()
RATIONAL_B_SPLINE_CURVE((1.,1.,1.,1.,1.,1.,1.,1.,1.,1.,1.,1.,1.,1.,1.,1.,
1.,1.,1.,1.,1.,1.,1.,1.,1.,1.,1.,1.,1.,1.,1.,1.,1.,1.,1.,1.,1.,1.,1.,1.,
1.,1.,1.,1.,1.,1.,1.,1.,1.,1.,1.,1.,1.,1.,1.,1.,1.,1.,1.,1.,1.,1.,1.,1.,
1.,1.,1.,1.,1.,1.))
REPRESENTATION_ITEM('')
);
#137=(
BOUNDED_CURVE()
B_SPLINE_CURVE(5,(#27242,#27243,#27244,#27245,#27246,#27247,#27248,#27249,
#27250,#27251,#27252,#27253,#27254,#27255,#27256,#27257,#27258,#27259,#27260,
#27261,#27262,#27263,#27264,#27265,#27266,#27267,#27268,#27269,#27270,#27271,
#27272,#27273,#27274,#27275,#27276,#27277,#27278,#27279,#27280,#27281,#27282,
#27283,#27284,#27285,#27286,#27287,#27288,#27289,#27290,#27291,#27292,#27293,
#27294,#27295,#27296,#27297,#27298,#27299,#27300,#27301,#27302,#27303,#27304,
#27305,#27306,#27307,#27308,#27309,#27310,#27311),.UNSPECIFIED.,.F.,.F.)
B_SPLINE_CURVE_WITH_KNOTS((6,1,1,1,1,1,1,1,1,1,1,1,1,1,1,1,1,1,1,1,1,1,
1,1,1,1,1,1,1,1,1,1,1,1,1,1,1,1,1,1,1,1,1,1,1,1,1,1,1,1,1,1,1,1,1,1,1,1,
1,1,1,1,1,1,1,6),(0.,0.0153846153846154,0.0307692307692308,0.0461538461538462,
0.0615384615384615,0.0769230769230769,0.0923076923076923,0.107692307692308,
0.123076923076923,0.138461538461538,0.153846153846154,0.169230769230769,
0.184615384615385,0.2,0.215384615384615,0.230769230769231,0.246153846153846,
0.261538461538462,0.276923076923077,0.292307692307692,0.307692307692308,
0.323076923076923,0.338461538461538,0.353846153846154,0.369230769230769,
0.384615384615385,0.4,0.415384615384615,0.430769230769231,0.446153846153846,
0.461538461538462,0.476923076923077,0.492307692307692,0.507692307692308,
0.523076923076923,0.538461538461538,0.553846153846154,0.569230769230769,
0.584615384615384,0.6,0.615384615384615,0.63076923076923,0.646153846153846,
0.661538461538461,0.676923076923076,0.692307692307692,0.707692307692307,
0.723076923076922,0.738461538461538,0.753846153846153,0.769230769230768,
0.784615384615384,0.799999999999999,0.815384615384614,0.83076923076923,
0.846153846153845,0.86153846153846,0.876923076923076,0.892307692307691,
0.907692307692306,0.923076923076922,0.938461538461537,0.953846153846152,
0.969230769230768,0.984615384615383,1.),.UNSPECIFIED.)
CURVE()
GEOMETRIC_REPRESENTATION_ITEM()
RATIONAL_B_SPLINE_CURVE((1.,1.,1.,1.,1.,1.,1.,1.,1.,1.,1.,1.,1.,1.,1.,1.,
1.,1.,1.,1.,1.,1.,1.,1.,1.,1.,1.,1.,1.,1.,1.,1.,1.,1.,1.,1.,1.,1.,1.,1.,
1.,1.,1.,1.,1.,1.,1.,1.,1.,1.,1.,1.,1.,1.,1.,1.,1.,1.,1.,1.,1.,1.,1.,1.,
1.,1.,1.,1.,1.,1.))
REPRESENTATION_ITEM('')
);
#138=(
BOUNDED_CURVE()
B_SPLINE_CURVE(5,(#27315,#27316,#27317,#27318,#27319,#27320,#27321,#27322,
#27323,#27324,#27325,#27326,#27327,#27328,#27329,#27330,#27331,#27332,#27333,
#27334,#27335,#27336,#27337,#27338,#27339,#27340,#27341,#27342,#27343,#27344,
#27345,#27346,#27347,#27348,#27349,#27350,#27351,#27352,#27353,#27354,#27355,
#27356,#27357,#27358,#27359,#27360,#27361,#27362,#27363,#27364,#27365,#27366,
#27367,#27368,#27369,#27370,#27371,#27372,#27373,#27374,#27375,#27376,#27377,
#27378,#27379,#27380,#27381,#27382,#27383,#27384),.UNSPECIFIED.,.F.,.F.)
B_SPLINE_CURVE_WITH_KNOTS((6,1,1,1,1,1,1,1,1,1,1,1,1,1,1,1,1,1,1,1,1,1,
1,1,1,1,1,1,1,1,1,1,1,1,1,1,1,1,1,1,1,1,1,1,1,1,1,1,1,1,1,1,1,1,1,1,1,1,
1,1,1,1,1,1,1,6),(0.,0.0153846153846154,0.0307692307692308,0.0461538461538462,
0.0615384615384615,0.0769230769230769,0.0923076923076923,0.107692307692308,
0.123076923076923,0.138461538461538,0.153846153846154,0.169230769230769,
0.184615384615385,0.2,0.215384615384615,0.230769230769231,0.246153846153846,
0.261538461538462,0.276923076923077,0.292307692307692,0.307692307692308,
0.323076923076923,0.338461538461538,0.353846153846154,0.369230769230769,
0.384615384615385,0.4,0.415384615384615,0.430769230769231,0.446153846153846,
0.461538461538462,0.476923076923077,0.492307692307692,0.507692307692308,
0.523076923076923,0.538461538461538,0.553846153846154,0.569230769230769,
0.584615384615384,0.6,0.615384615384615,0.63076923076923,0.646153846153846,
0.661538461538461,0.676923076923076,0.692307692307692,0.707692307692307,
0.723076923076922,0.738461538461538,0.753846153846153,0.769230769230768,
0.784615384615384,0.799999999999999,0.815384615384614,0.83076923076923,
0.846153846153845,0.86153846153846,0.876923076923076,0.892307692307691,
0.907692307692306,0.923076923076922,0.938461538461537,0.953846153846152,
0.969230769230768,0.984615384615383,1.),.UNSPECIFIED.)
CURVE()
GEOMETRIC_REPRESENTATION_ITEM()
RATIONAL_B_SPLINE_CURVE((1.,1.,1.,1.,1.,1.,1.,1.,1.,1.,1.,1.,1.,1.,1.,1.,
1.,1.,1.,1.,1.,1.,1.,1.,1.,1.,1.,1.,1.,1.,1.,1.,1.,1.,1.,1.,1.,1.,1.,1.,
1.,1.,1.,1.,1.,1.,1.,1.,1.,1.,1.,1.,1.,1.,1.,1.,1.,1.,1.,1.,1.,1.,1.,1.,
1.,1.,1.,1.,1.,1.))
REPRESENTATION_ITEM('')
);
#139=(
BOUNDED_CURVE()
B_SPLINE_CURVE(5,(#27388,#27389,#27390,#27391,#27392,#27393,#27394,#27395,
#27396,#27397,#27398,#27399,#27400,#27401,#27402,#27403,#27404,#27405,#27406,
#27407,#27408,#27409,#27410,#27411,#27412,#27413,#27414,#27415,#27416,#27417,
#27418,#27419,#27420,#27421,#27422,#27423,#27424,#27425,#27426,#27427,#27428,
#27429,#27430,#27431,#27432,#27433,#27434,#27435,#27436,#27437,#27438,#27439,
#27440,#27441,#27442,#27443,#27444,#27445,#27446,#27447,#27448,#27449,#27450,
#27451,#27452,#27453,#27454,#27455,#27456,#27457),.UNSPECIFIED.,.F.,.F.)
B_SPLINE_CURVE_WITH_KNOTS((6,1,1,1,1,1,1,1,1,1,1,1,1,1,1,1,1,1,1,1,1,1,
1,1,1,1,1,1,1,1,1,1,1,1,1,1,1,1,1,1,1,1,1,1,1,1,1,1,1,1,1,1,1,1,1,1,1,1,
1,1,1,1,1,1,1,6),(0.,0.0153846153846154,0.0307692307692308,0.0461538461538462,
0.0615384615384615,0.0769230769230769,0.0923076923076923,0.107692307692308,
0.123076923076923,0.138461538461538,0.153846153846154,0.169230769230769,
0.184615384615385,0.2,0.215384615384615,0.230769230769231,0.246153846153846,
0.261538461538462,0.276923076923077,0.292307692307692,0.307692307692308,
0.323076923076923,0.338461538461538,0.353846153846154,0.369230769230769,
0.384615384615385,0.4,0.415384615384615,0.430769230769231,0.446153846153846,
0.461538461538462,0.476923076923077,0.492307692307692,0.507692307692308,
0.523076923076923,0.538461538461538,0.553846153846154,0.569230769230769,
0.584615384615384,0.6,0.615384615384615,0.63076923076923,0.646153846153846,
0.661538461538461,0.676923076923076,0.692307692307692,0.707692307692307,
0.723076923076922,0.738461538461538,0.753846153846153,0.769230769230768,
0.784615384615384,0.799999999999999,0.815384615384614,0.83076923076923,
0.846153846153845,0.86153846153846,0.876923076923076,0.892307692307691,
0.907692307692306,0.923076923076922,0.938461538461537,0.953846153846152,
0.969230769230768,0.984615384615383,1.),.UNSPECIFIED.)
CURVE()
GEOMETRIC_REPRESENTATION_ITEM()
RATIONAL_B_SPLINE_CURVE((1.,1.,1.,1.,1.,1.,1.,1.,1.,1.,1.,1.,1.,1.,1.,1.,
1.,1.,1.,1.,1.,1.,1.,1.,1.,1.,1.,1.,1.,1.,1.,1.,1.,1.,1.,1.,1.,1.,1.,1.,
1.,1.,1.,1.,1.,1.,1.,1.,1.,1.,1.,1.,1.,1.,1.,1.,1.,1.,1.,1.,1.,1.,1.,1.,
1.,1.,1.,1.,1.,1.))
REPRESENTATION_ITEM('')
);
#140=(
BOUNDED_CURVE()
B_SPLINE_CURVE(5,(#27461,#27462,#27463,#27464,#27465,#27466,#27467,#27468,
#27469,#27470,#27471,#27472,#27473,#27474,#27475,#27476,#27477,#27478,#27479,
#27480,#27481,#27482,#27483,#27484,#27485,#27486,#27487,#27488,#27489,#27490,
#27491,#27492,#27493,#27494,#27495,#27496,#27497,#27498,#27499,#27500,#27501,
#27502,#27503,#27504,#27505,#27506,#27507,#27508,#27509,#27510,#27511,#27512,
#27513,#27514,#27515,#27516,#27517,#27518,#27519,#27520,#27521,#27522,#27523,
#27524,#27525,#27526,#27527,#27528,#27529,#27530),.UNSPECIFIED.,.F.,.F.)
B_SPLINE_CURVE_WITH_KNOTS((6,1,1,1,1,1,1,1,1,1,1,1,1,1,1,1,1,1,1,1,1,1,
1,1,1,1,1,1,1,1,1,1,1,1,1,1,1,1,1,1,1,1,1,1,1,1,1,1,1,1,1,1,1,1,1,1,1,1,
1,1,1,1,1,1,1,6),(0.,0.0153846153846154,0.0307692307692308,0.0461538461538462,
0.0615384615384615,0.0769230769230769,0.0923076923076923,0.107692307692308,
0.123076923076923,0.138461538461538,0.153846153846154,0.169230769230769,
0.184615384615385,0.2,0.215384615384615,0.230769230769231,0.246153846153846,
0.261538461538462,0.276923076923077,0.292307692307692,0.307692307692308,
0.323076923076923,0.338461538461538,0.353846153846154,0.369230769230769,
0.384615384615385,0.4,0.415384615384615,0.430769230769231,0.446153846153846,
0.461538461538462,0.476923076923077,0.492307692307692,0.507692307692308,
0.523076923076923,0.538461538461538,0.553846153846154,0.569230769230769,
0.584615384615384,0.6,0.615384615384615,0.63076923076923,0.646153846153846,
0.661538461538461,0.676923076923076,0.692307692307692,0.707692307692307,
0.723076923076922,0.738461538461538,0.753846153846153,0.769230769230768,
0.784615384615384,0.799999999999999,0.815384615384614,0.83076923076923,
0.846153846153845,0.86153846153846,0.876923076923076,0.892307692307691,
0.907692307692306,0.923076923076922,0.938461538461537,0.953846153846152,
0.969230769230768,0.984615384615383,1.),.UNSPECIFIED.)
CURVE()
GEOMETRIC_REPRESENTATION_ITEM()
RATIONAL_B_SPLINE_CURVE((1.,1.,1.,1.,1.,1.,1.,1.,1.,1.,1.,1.,1.,1.,1.,1.,
1.,1.,1.,1.,1.,1.,1.,1.,1.,1.,1.,1.,1.,1.,1.,1.,1.,1.,1.,1.,1.,1.,1.,1.,
1.,1.,1.,1.,1.,1.,1.,1.,1.,1.,1.,1.,1.,1.,1.,1.,1.,1.,1.,1.,1.,1.,1.,1.,
1.,1.,1.,1.,1.,1.))
REPRESENTATION_ITEM('')
);
#141=(
BOUNDED_CURVE()
B_SPLINE_CURVE(5,(#27534,#27535,#27536,#27537,#27538,#27539,#27540,#27541,
#27542,#27543,#27544,#27545,#27546,#27547,#27548,#27549,#27550,#27551,#27552,
#27553,#27554,#27555,#27556,#27557,#27558,#27559,#27560,#27561,#27562,#27563,
#27564,#27565,#27566,#27567,#27568,#27569,#27570,#27571,#27572,#27573,#27574,
#27575,#27576,#27577,#27578,#27579,#27580,#27581,#27582,#27583,#27584,#27585,
#27586,#27587,#27588,#27589,#27590,#27591,#27592,#27593,#27594,#27595,#27596,
#27597,#27598,#27599,#27600,#27601,#27602,#27603),.UNSPECIFIED.,.F.,.F.)
B_SPLINE_CURVE_WITH_KNOTS((6,1,1,1,1,1,1,1,1,1,1,1,1,1,1,1,1,1,1,1,1,1,
1,1,1,1,1,1,1,1,1,1,1,1,1,1,1,1,1,1,1,1,1,1,1,1,1,1,1,1,1,1,1,1,1,1,1,1,
1,1,1,1,1,1,1,6),(0.,0.0153846153846154,0.0307692307692308,0.0461538461538462,
0.0615384615384615,0.0769230769230769,0.0923076923076923,0.107692307692308,
0.123076923076923,0.138461538461538,0.153846153846154,0.169230769230769,
0.184615384615385,0.2,0.215384615384615,0.230769230769231,0.246153846153846,
0.261538461538462,0.276923076923077,0.292307692307692,0.307692307692308,
0.323076923076923,0.338461538461538,0.353846153846154,0.369230769230769,
0.384615384615385,0.4,0.415384615384615,0.430769230769231,0.446153846153846,
0.461538461538462,0.476923076923077,0.492307692307692,0.507692307692308,
0.523076923076923,0.538461538461538,0.553846153846154,0.569230769230769,
0.584615384615384,0.6,0.615384615384615,0.63076923076923,0.646153846153846,
0.661538461538461,0.676923076923076,0.692307692307692,0.707692307692307,
0.723076923076922,0.738461538461538,0.753846153846153,0.769230769230768,
0.784615384615384,0.799999999999999,0.815384615384614,0.83076923076923,
0.846153846153845,0.86153846153846,0.876923076923076,0.892307692307691,
0.907692307692306,0.923076923076922,0.938461538461537,0.953846153846152,
0.969230769230768,0.984615384615383,1.),.UNSPECIFIED.)
CURVE()
GEOMETRIC_REPRESENTATION_ITEM()
RATIONAL_B_SPLINE_CURVE((1.,1.,1.,1.,1.,1.,1.,1.,1.,1.,1.,1.,1.,1.,1.,1.,
1.,1.,1.,1.,1.,1.,1.,1.,1.,1.,1.,1.,1.,1.,1.,1.,1.,1.,1.,1.,1.,1.,1.,1.,
1.,1.,1.,1.,1.,1.,1.,1.,1.,1.,1.,1.,1.,1.,1.,1.,1.,1.,1.,1.,1.,1.,1.,1.,
1.,1.,1.,1.,1.,1.))
REPRESENTATION_ITEM('')
);
#142=(
BOUNDED_CURVE()
B_SPLINE_CURVE(5,(#27607,#27608,#27609,#27610,#27611,#27612,#27613,#27614,
#27615,#27616,#27617,#27618,#27619,#27620,#27621,#27622,#27623,#27624,#27625,
#27626,#27627,#27628,#27629,#27630,#27631,#27632,#27633,#27634,#27635,#27636,
#27637,#27638,#27639,#27640,#27641,#27642,#27643,#27644,#27645,#27646,#27647,
#27648,#27649,#27650,#27651,#27652,#27653,#27654,#27655,#27656,#27657,#27658,
#27659,#27660,#27661,#27662,#27663,#27664,#27665,#27666,#27667,#27668,#27669,
#27670,#27671,#27672,#27673,#27674,#27675,#27676),.UNSPECIFIED.,.F.,.F.)
B_SPLINE_CURVE_WITH_KNOTS((6,1,1,1,1,1,1,1,1,1,1,1,1,1,1,1,1,1,1,1,1,1,
1,1,1,1,1,1,1,1,1,1,1,1,1,1,1,1,1,1,1,1,1,1,1,1,1,1,1,1,1,1,1,1,1,1,1,1,
1,1,1,1,1,1,1,6),(0.,0.0153846153846154,0.0307692307692308,0.0461538461538462,
0.0615384615384615,0.0769230769230769,0.0923076923076923,0.107692307692308,
0.123076923076923,0.138461538461538,0.153846153846154,0.169230769230769,
0.184615384615385,0.2,0.215384615384615,0.230769230769231,0.246153846153846,
0.261538461538462,0.276923076923077,0.292307692307692,0.307692307692308,
0.323076923076923,0.338461538461538,0.353846153846154,0.369230769230769,
0.384615384615385,0.4,0.415384615384615,0.430769230769231,0.446153846153846,
0.461538461538462,0.476923076923077,0.492307692307692,0.507692307692308,
0.523076923076923,0.538461538461538,0.553846153846154,0.569230769230769,
0.584615384615384,0.6,0.615384615384615,0.63076923076923,0.646153846153846,
0.661538461538461,0.676923076923076,0.692307692307692,0.707692307692307,
0.723076923076922,0.738461538461538,0.753846153846153,0.769230769230768,
0.784615384615384,0.799999999999999,0.815384615384614,0.83076923076923,
0.846153846153845,0.86153846153846,0.876923076923076,0.892307692307691,
0.907692307692306,0.923076923076922,0.938461538461537,0.953846153846152,
0.969230769230768,0.984615384615383,1.),.UNSPECIFIED.)
CURVE()
GEOMETRIC_REPRESENTATION_ITEM()
RATIONAL_B_SPLINE_CURVE((1.,1.,1.,1.,1.,1.,1.,1.,1.,1.,1.,1.,1.,1.,1.,1.,
1.,1.,1.,1.,1.,1.,1.,1.,1.,1.,1.,1.,1.,1.,1.,1.,1.,1.,1.,1.,1.,1.,1.,1.,
1.,1.,1.,1.,1.,1.,1.,1.,1.,1.,1.,1.,1.,1.,1.,1.,1.,1.,1.,1.,1.,1.,1.,1.,
1.,1.,1.,1.,1.,1.))
REPRESENTATION_ITEM('')
);
#143=(
BOUNDED_CURVE()
B_SPLINE_CURVE(5,(#27680,#27681,#27682,#27683,#27684,#27685,#27686,#27687,
#27688,#27689,#27690,#27691,#27692,#27693,#27694,#27695,#27696,#27697,#27698,
#27699,#27700,#27701,#27702,#27703,#27704,#27705,#27706,#27707,#27708,#27709,
#27710,#27711,#27712,#27713,#27714,#27715,#27716,#27717,#27718,#27719,#27720,
#27721,#27722,#27723,#27724,#27725,#27726,#27727,#27728,#27729,#27730,#27731,
#27732,#27733,#27734,#27735,#27736,#27737,#27738,#27739,#27740,#27741,#27742,
#27743,#27744,#27745,#27746,#27747,#27748,#27749),.UNSPECIFIED.,.F.,.F.)
B_SPLINE_CURVE_WITH_KNOTS((6,1,1,1,1,1,1,1,1,1,1,1,1,1,1,1,1,1,1,1,1,1,
1,1,1,1,1,1,1,1,1,1,1,1,1,1,1,1,1,1,1,1,1,1,1,1,1,1,1,1,1,1,1,1,1,1,1,1,
1,1,1,1,1,1,1,6),(0.,0.0153846153846154,0.0307692307692308,0.0461538461538462,
0.0615384615384615,0.0769230769230769,0.0923076923076923,0.107692307692308,
0.123076923076923,0.138461538461538,0.153846153846154,0.169230769230769,
0.184615384615385,0.2,0.215384615384615,0.230769230769231,0.246153846153846,
0.261538461538462,0.276923076923077,0.292307692307692,0.307692307692308,
0.323076923076923,0.338461538461538,0.353846153846154,0.369230769230769,
0.384615384615385,0.4,0.415384615384615,0.430769230769231,0.446153846153846,
0.461538461538462,0.476923076923077,0.492307692307692,0.507692307692308,
0.523076923076923,0.538461538461538,0.553846153846154,0.569230769230769,
0.584615384615384,0.6,0.615384615384615,0.63076923076923,0.646153846153846,
0.661538461538461,0.676923076923076,0.692307692307692,0.707692307692307,
0.723076923076922,0.738461538461538,0.753846153846153,0.769230769230768,
0.784615384615384,0.799999999999999,0.815384615384614,0.83076923076923,
0.846153846153845,0.86153846153846,0.876923076923076,0.892307692307691,
0.907692307692306,0.923076923076922,0.938461538461537,0.953846153846152,
0.969230769230768,0.984615384615383,1.),.UNSPECIFIED.)
CURVE()
GEOMETRIC_REPRESENTATION_ITEM()
RATIONAL_B_SPLINE_CURVE((1.,1.,1.,1.,1.,1.,1.,1.,1.,1.,1.,1.,1.,1.,1.,1.,
1.,1.,1.,1.,1.,1.,1.,1.,1.,1.,1.,1.,1.,1.,1.,1.,1.,1.,1.,1.,1.,1.,1.,1.,
1.,1.,1.,1.,1.,1.,1.,1.,1.,1.,1.,1.,1.,1.,1.,1.,1.,1.,1.,1.,1.,1.,1.,1.,
1.,1.,1.,1.,1.,1.))
REPRESENTATION_ITEM('')
);
#144=(
BOUNDED_CURVE()
B_SPLINE_CURVE(5,(#27753,#27754,#27755,#27756,#27757,#27758,#27759,#27760,
#27761,#27762,#27763,#27764,#27765,#27766,#27767,#27768,#27769,#27770,#27771,
#27772,#27773,#27774,#27775,#27776,#27777,#27778,#27779,#27780,#27781,#27782,
#27783,#27784,#27785,#27786,#27787,#27788,#27789,#27790,#27791,#27792,#27793,
#27794,#27795,#27796,#27797,#27798,#27799,#27800,#27801,#27802,#27803,#27804,
#27805,#27806,#27807,#27808,#27809,#27810,#27811,#27812,#27813,#27814,#27815,
#27816,#27817,#27818,#27819,#27820,#27821,#27822),.UNSPECIFIED.,.F.,.F.)
B_SPLINE_CURVE_WITH_KNOTS((6,1,1,1,1,1,1,1,1,1,1,1,1,1,1,1,1,1,1,1,1,1,
1,1,1,1,1,1,1,1,1,1,1,1,1,1,1,1,1,1,1,1,1,1,1,1,1,1,1,1,1,1,1,1,1,1,1,1,
1,1,1,1,1,1,1,6),(0.,0.0153846153846154,0.0307692307692308,0.0461538461538462,
0.0615384615384615,0.0769230769230769,0.0923076923076923,0.107692307692308,
0.123076923076923,0.138461538461538,0.153846153846154,0.169230769230769,
0.184615384615385,0.2,0.215384615384615,0.230769230769231,0.246153846153846,
0.261538461538462,0.276923076923077,0.292307692307692,0.307692307692308,
0.323076923076923,0.338461538461538,0.353846153846154,0.369230769230769,
0.384615384615385,0.4,0.415384615384615,0.430769230769231,0.446153846153846,
0.461538461538462,0.476923076923077,0.492307692307692,0.507692307692308,
0.523076923076923,0.538461538461538,0.553846153846154,0.569230769230769,
0.584615384615384,0.6,0.615384615384615,0.63076923076923,0.646153846153846,
0.661538461538461,0.676923076923076,0.692307692307692,0.707692307692307,
0.723076923076922,0.738461538461538,0.753846153846153,0.769230769230768,
0.784615384615384,0.799999999999999,0.815384615384614,0.83076923076923,
0.846153846153845,0.86153846153846,0.876923076923076,0.892307692307691,
0.907692307692306,0.923076923076922,0.938461538461537,0.953846153846152,
0.969230769230768,0.984615384615383,1.),.UNSPECIFIED.)
CURVE()
GEOMETRIC_REPRESENTATION_ITEM()
RATIONAL_B_SPLINE_CURVE((1.,1.,1.,1.,1.,1.,1.,1.,1.,1.,1.,1.,1.,1.,1.,1.,
1.,1.,1.,1.,1.,1.,1.,1.,1.,1.,1.,1.,1.,1.,1.,1.,1.,1.,1.,1.,1.,1.,1.,1.,
1.,1.,1.,1.,1.,1.,1.,1.,1.,1.,1.,1.,1.,1.,1.,1.,1.,1.,1.,1.,1.,1.,1.,1.,
1.,1.,1.,1.,1.,1.))
REPRESENTATION_ITEM('')
);
#145=(
BOUNDED_CURVE()
B_SPLINE_CURVE(5,(#27826,#27827,#27828,#27829,#27830,#27831,#27832,#27833,
#27834,#27835,#27836,#27837,#27838,#27839,#27840,#27841,#27842,#27843,#27844,
#27845,#27846,#27847,#27848,#27849,#27850,#27851,#27852,#27853,#27854,#27855,
#27856,#27857,#27858,#27859,#27860,#27861,#27862,#27863,#27864,#27865,#27866,
#27867,#27868,#27869,#27870,#27871,#27872,#27873,#27874,#27875,#27876,#27877,
#27878,#27879,#27880,#27881,#27882,#27883,#27884,#27885,#27886,#27887,#27888,
#27889,#27890,#27891,#27892,#27893,#27894,#27895),.UNSPECIFIED.,.F.,.F.)
B_SPLINE_CURVE_WITH_KNOTS((6,1,1,1,1,1,1,1,1,1,1,1,1,1,1,1,1,1,1,1,1,1,
1,1,1,1,1,1,1,1,1,1,1,1,1,1,1,1,1,1,1,1,1,1,1,1,1,1,1,1,1,1,1,1,1,1,1,1,
1,1,1,1,1,1,1,6),(0.,0.0153846153846154,0.0307692307692308,0.0461538461538462,
0.0615384615384615,0.0769230769230769,0.0923076923076923,0.107692307692308,
0.123076923076923,0.138461538461538,0.153846153846154,0.169230769230769,
0.184615384615385,0.2,0.215384615384615,0.230769230769231,0.246153846153846,
0.261538461538462,0.276923076923077,0.292307692307692,0.307692307692308,
0.323076923076923,0.338461538461538,0.353846153846154,0.369230769230769,
0.384615384615385,0.4,0.415384615384615,0.430769230769231,0.446153846153846,
0.461538461538462,0.476923076923077,0.492307692307692,0.507692307692308,
0.523076923076923,0.538461538461538,0.553846153846154,0.569230769230769,
0.584615384615384,0.6,0.615384615384615,0.63076923076923,0.646153846153846,
0.661538461538461,0.676923076923076,0.692307692307692,0.707692307692307,
0.723076923076922,0.738461538461538,0.753846153846153,0.769230769230768,
0.784615384615384,0.799999999999999,0.815384615384614,0.83076923076923,
0.846153846153845,0.86153846153846,0.876923076923076,0.892307692307691,
0.907692307692306,0.923076923076922,0.938461538461537,0.953846153846152,
0.969230769230768,0.984615384615383,1.),.UNSPECIFIED.)
CURVE()
GEOMETRIC_REPRESENTATION_ITEM()
RATIONAL_B_SPLINE_CURVE((1.,1.,1.,1.,1.,1.,1.,1.,1.,1.,1.,1.,1.,1.,1.,1.,
1.,1.,1.,1.,1.,1.,1.,1.,1.,1.,1.,1.,1.,1.,1.,1.,1.,1.,1.,1.,1.,1.,1.,1.,
1.,1.,1.,1.,1.,1.,1.,1.,1.,1.,1.,1.,1.,1.,1.,1.,1.,1.,1.,1.,1.,1.,1.,1.,
1.,1.,1.,1.,1.,1.))
REPRESENTATION_ITEM('')
);
#146=(
BOUNDED_CURVE()
B_SPLINE_CURVE(5,(#27899,#27900,#27901,#27902,#27903,#27904,#27905,#27906,
#27907,#27908,#27909,#27910,#27911,#27912,#27913,#27914,#27915,#27916,#27917,
#27918,#27919,#27920,#27921,#27922,#27923,#27924,#27925,#27926,#27927,#27928,
#27929,#27930,#27931,#27932,#27933,#27934,#27935,#27936,#27937,#27938,#27939,
#27940,#27941,#27942,#27943,#27944,#27945,#27946,#27947,#27948,#27949,#27950,
#27951,#27952,#27953,#27954,#27955,#27956,#27957,#27958,#27959,#27960,#27961,
#27962,#27963,#27964,#27965,#27966,#27967,#27968),.UNSPECIFIED.,.F.,.F.)
B_SPLINE_CURVE_WITH_KNOTS((6,1,1,1,1,1,1,1,1,1,1,1,1,1,1,1,1,1,1,1,1,1,
1,1,1,1,1,1,1,1,1,1,1,1,1,1,1,1,1,1,1,1,1,1,1,1,1,1,1,1,1,1,1,1,1,1,1,1,
1,1,1,1,1,1,1,6),(0.,0.0153846153846154,0.0307692307692308,0.0461538461538462,
0.0615384615384615,0.0769230769230769,0.0923076923076923,0.107692307692308,
0.123076923076923,0.138461538461538,0.153846153846154,0.169230769230769,
0.184615384615385,0.2,0.215384615384615,0.230769230769231,0.246153846153846,
0.261538461538462,0.276923076923077,0.292307692307692,0.307692307692308,
0.323076923076923,0.338461538461538,0.353846153846154,0.369230769230769,
0.384615384615385,0.4,0.415384615384615,0.430769230769231,0.446153846153846,
0.461538461538462,0.476923076923077,0.492307692307692,0.507692307692308,
0.523076923076923,0.538461538461538,0.553846153846154,0.569230769230769,
0.584615384615384,0.6,0.615384615384615,0.63076923076923,0.646153846153846,
0.661538461538461,0.676923076923076,0.692307692307692,0.707692307692307,
0.723076923076922,0.738461538461538,0.753846153846153,0.769230769230768,
0.784615384615384,0.799999999999999,0.815384615384614,0.83076923076923,
0.846153846153845,0.86153846153846,0.876923076923076,0.892307692307691,
0.907692307692306,0.923076923076922,0.938461538461537,0.953846153846152,
0.969230769230768,0.984615384615383,1.),.UNSPECIFIED.)
CURVE()
GEOMETRIC_REPRESENTATION_ITEM()
RATIONAL_B_SPLINE_CURVE((1.,1.,1.,1.,1.,1.,1.,1.,1.,1.,1.,1.,1.,1.,1.,1.,
1.,1.,1.,1.,1.,1.,1.,1.,1.,1.,1.,1.,1.,1.,1.,1.,1.,1.,1.,1.,1.,1.,1.,1.,
1.,1.,1.,1.,1.,1.,1.,1.,1.,1.,1.,1.,1.,1.,1.,1.,1.,1.,1.,1.,1.,1.,1.,1.,
1.,1.,1.,1.,1.,1.))
REPRESENTATION_ITEM('')
);
#147=(
BOUNDED_CURVE()
B_SPLINE_CURVE(5,(#27972,#27973,#27974,#27975,#27976,#27977,#27978,#27979,
#27980,#27981,#27982,#27983,#27984,#27985,#27986,#27987,#27988,#27989,#27990,
#27991,#27992,#27993,#27994,#27995,#27996,#27997,#27998,#27999,#28000,#28001,
#28002,#28003,#28004,#28005,#28006,#28007,#28008,#28009,#28010,#28011,#28012,
#28013,#28014,#28015,#28016,#28017,#28018,#28019,#28020,#28021,#28022,#28023,
#28024,#28025,#28026,#28027,#28028,#28029,#28030,#28031,#28032,#28033,#28034,
#28035,#28036,#28037,#28038,#28039,#28040,#28041),.UNSPECIFIED.,.F.,.F.)
B_SPLINE_CURVE_WITH_KNOTS((6,1,1,1,1,1,1,1,1,1,1,1,1,1,1,1,1,1,1,1,1,1,
1,1,1,1,1,1,1,1,1,1,1,1,1,1,1,1,1,1,1,1,1,1,1,1,1,1,1,1,1,1,1,1,1,1,1,1,
1,1,1,1,1,1,1,6),(0.,0.0153846153846154,0.0307692307692308,0.0461538461538462,
0.0615384615384615,0.0769230769230769,0.0923076923076923,0.107692307692308,
0.123076923076923,0.138461538461538,0.153846153846154,0.169230769230769,
0.184615384615385,0.2,0.215384615384615,0.230769230769231,0.246153846153846,
0.261538461538462,0.276923076923077,0.292307692307692,0.307692307692308,
0.323076923076923,0.338461538461538,0.353846153846154,0.369230769230769,
0.384615384615385,0.4,0.415384615384615,0.430769230769231,0.446153846153846,
0.461538461538462,0.476923076923077,0.492307692307692,0.507692307692308,
0.523076923076923,0.538461538461538,0.553846153846154,0.569230769230769,
0.584615384615384,0.6,0.615384615384615,0.63076923076923,0.646153846153846,
0.661538461538461,0.676923076923076,0.692307692307692,0.707692307692307,
0.723076923076922,0.738461538461538,0.753846153846153,0.769230769230768,
0.784615384615384,0.799999999999999,0.815384615384614,0.83076923076923,
0.846153846153845,0.86153846153846,0.876923076923076,0.892307692307691,
0.907692307692306,0.923076923076922,0.938461538461537,0.953846153846152,
0.969230769230768,0.984615384615383,1.),.UNSPECIFIED.)
CURVE()
GEOMETRIC_REPRESENTATION_ITEM()
RATIONAL_B_SPLINE_CURVE((1.,1.,1.,1.,1.,1.,1.,1.,1.,1.,1.,1.,1.,1.,1.,1.,
1.,1.,1.,1.,1.,1.,1.,1.,1.,1.,1.,1.,1.,1.,1.,1.,1.,1.,1.,1.,1.,1.,1.,1.,
1.,1.,1.,1.,1.,1.,1.,1.,1.,1.,1.,1.,1.,1.,1.,1.,1.,1.,1.,1.,1.,1.,1.,1.,
1.,1.,1.,1.,1.,1.))
REPRESENTATION_ITEM('')
);
#148=(
BOUNDED_CURVE()
B_SPLINE_CURVE(5,(#28045,#28046,#28047,#28048,#28049,#28050,#28051,#28052,
#28053,#28054,#28055,#28056,#28057,#28058,#28059,#28060,#28061,#28062,#28063,
#28064,#28065,#28066,#28067,#28068,#28069,#28070,#28071,#28072,#28073,#28074,
#28075,#28076,#28077,#28078,#28079,#28080,#28081,#28082,#28083,#28084,#28085,
#28086,#28087,#28088,#28089,#28090,#28091,#28092,#28093,#28094,#28095,#28096,
#28097,#28098,#28099,#28100,#28101,#28102,#28103,#28104,#28105,#28106,#28107,
#28108,#28109,#28110,#28111,#28112,#28113,#28114),.UNSPECIFIED.,.F.,.F.)
B_SPLINE_CURVE_WITH_KNOTS((6,1,1,1,1,1,1,1,1,1,1,1,1,1,1,1,1,1,1,1,1,1,
1,1,1,1,1,1,1,1,1,1,1,1,1,1,1,1,1,1,1,1,1,1,1,1,1,1,1,1,1,1,1,1,1,1,1,1,
1,1,1,1,1,1,1,6),(0.,0.0153846153846154,0.0307692307692308,0.0461538461538462,
0.0615384615384615,0.0769230769230769,0.0923076923076923,0.107692307692308,
0.123076923076923,0.138461538461538,0.153846153846154,0.169230769230769,
0.184615384615385,0.2,0.215384615384615,0.230769230769231,0.246153846153846,
0.261538461538462,0.276923076923077,0.292307692307692,0.307692307692308,
0.323076923076923,0.338461538461538,0.353846153846154,0.369230769230769,
0.384615384615385,0.4,0.415384615384615,0.430769230769231,0.446153846153846,
0.461538461538462,0.476923076923077,0.492307692307692,0.507692307692308,
0.523076923076923,0.538461538461538,0.553846153846154,0.569230769230769,
0.584615384615384,0.6,0.615384615384615,0.63076923076923,0.646153846153846,
0.661538461538461,0.676923076923076,0.692307692307692,0.707692307692307,
0.723076923076922,0.738461538461538,0.753846153846153,0.769230769230768,
0.784615384615384,0.799999999999999,0.815384615384614,0.83076923076923,
0.846153846153845,0.86153846153846,0.876923076923076,0.892307692307691,
0.907692307692306,0.923076923076922,0.938461538461537,0.953846153846152,
0.969230769230768,0.984615384615383,1.),.UNSPECIFIED.)
CURVE()
GEOMETRIC_REPRESENTATION_ITEM()
RATIONAL_B_SPLINE_CURVE((1.,1.,1.,1.,1.,1.,1.,1.,1.,1.,1.,1.,1.,1.,1.,1.,
1.,1.,1.,1.,1.,1.,1.,1.,1.,1.,1.,1.,1.,1.,1.,1.,1.,1.,1.,1.,1.,1.,1.,1.,
1.,1.,1.,1.,1.,1.,1.,1.,1.,1.,1.,1.,1.,1.,1.,1.,1.,1.,1.,1.,1.,1.,1.,1.,
1.,1.,1.,1.,1.,1.))
REPRESENTATION_ITEM('')
);
#149=(
BOUNDED_CURVE()
B_SPLINE_CURVE(5,(#28118,#28119,#28120,#28121,#28122,#28123,#28124,#28125,
#28126,#28127,#28128,#28129,#28130,#28131,#28132,#28133,#28134,#28135,#28136,
#28137,#28138,#28139,#28140,#28141,#28142,#28143,#28144,#28145,#28146,#28147,
#28148,#28149,#28150,#28151,#28152,#28153,#28154,#28155,#28156,#28157,#28158,
#28159,#28160,#28161,#28162,#28163,#28164,#28165,#28166,#28167,#28168,#28169,
#28170,#28171,#28172,#28173,#28174,#28175,#28176,#28177,#28178,#28179,#28180,
#28181,#28182,#28183,#28184,#28185,#28186,#28187),.UNSPECIFIED.,.F.,.F.)
B_SPLINE_CURVE_WITH_KNOTS((6,1,1,1,1,1,1,1,1,1,1,1,1,1,1,1,1,1,1,1,1,1,
1,1,1,1,1,1,1,1,1,1,1,1,1,1,1,1,1,1,1,1,1,1,1,1,1,1,1,1,1,1,1,1,1,1,1,1,
1,1,1,1,1,1,1,6),(0.,0.0153846153846154,0.0307692307692308,0.0461538461538462,
0.0615384615384615,0.0769230769230769,0.0923076923076923,0.107692307692308,
0.123076923076923,0.138461538461538,0.153846153846154,0.169230769230769,
0.184615384615385,0.2,0.215384615384615,0.230769230769231,0.246153846153846,
0.261538461538462,0.276923076923077,0.292307692307692,0.307692307692308,
0.323076923076923,0.338461538461538,0.353846153846154,0.369230769230769,
0.384615384615385,0.4,0.415384615384615,0.430769230769231,0.446153846153846,
0.461538461538462,0.476923076923077,0.492307692307692,0.507692307692308,
0.523076923076923,0.538461538461538,0.553846153846154,0.569230769230769,
0.584615384615384,0.6,0.615384615384615,0.63076923076923,0.646153846153846,
0.661538461538461,0.676923076923076,0.692307692307692,0.707692307692307,
0.723076923076922,0.738461538461538,0.753846153846153,0.769230769230768,
0.784615384615384,0.799999999999999,0.815384615384614,0.83076923076923,
0.846153846153845,0.86153846153846,0.876923076923076,0.892307692307691,
0.907692307692306,0.923076923076922,0.938461538461537,0.953846153846152,
0.969230769230768,0.984615384615383,1.),.UNSPECIFIED.)
CURVE()
GEOMETRIC_REPRESENTATION_ITEM()
RATIONAL_B_SPLINE_CURVE((1.,1.,1.,1.,1.,1.,1.,1.,1.,1.,1.,1.,1.,1.,1.,1.,
1.,1.,1.,1.,1.,1.,1.,1.,1.,1.,1.,1.,1.,1.,1.,1.,1.,1.,1.,1.,1.,1.,1.,1.,
1.,1.,1.,1.,1.,1.,1.,1.,1.,1.,1.,1.,1.,1.,1.,1.,1.,1.,1.,1.,1.,1.,1.,1.,
1.,1.,1.,1.,1.,1.))
REPRESENTATION_ITEM('')
);
#150=(
BOUNDED_CURVE()
B_SPLINE_CURVE(5,(#28191,#28192,#28193,#28194,#28195,#28196,#28197,#28198,
#28199,#28200,#28201,#28202,#28203,#28204,#28205,#28206,#28207,#28208,#28209,
#28210,#28211,#28212,#28213,#28214,#28215,#28216,#28217,#28218,#28219,#28220,
#28221,#28222,#28223,#28224,#28225,#28226,#28227,#28228,#28229,#28230,#28231,
#28232,#28233,#28234,#28235,#28236,#28237,#28238,#28239,#28240,#28241,#28242,
#28243,#28244,#28245,#28246,#28247,#28248,#28249,#28250,#28251,#28252,#28253,
#28254,#28255,#28256,#28257,#28258,#28259,#28260),.UNSPECIFIED.,.F.,.F.)
B_SPLINE_CURVE_WITH_KNOTS((6,1,1,1,1,1,1,1,1,1,1,1,1,1,1,1,1,1,1,1,1,1,
1,1,1,1,1,1,1,1,1,1,1,1,1,1,1,1,1,1,1,1,1,1,1,1,1,1,1,1,1,1,1,1,1,1,1,1,
1,1,1,1,1,1,1,6),(0.,0.0153846153846154,0.0307692307692308,0.0461538461538462,
0.0615384615384615,0.0769230769230769,0.0923076923076923,0.107692307692308,
0.123076923076923,0.138461538461538,0.153846153846154,0.169230769230769,
0.184615384615385,0.2,0.215384615384615,0.230769230769231,0.246153846153846,
0.261538461538462,0.276923076923077,0.292307692307692,0.307692307692308,
0.323076923076923,0.338461538461538,0.353846153846154,0.369230769230769,
0.384615384615385,0.4,0.415384615384615,0.430769230769231,0.446153846153846,
0.461538461538462,0.476923076923077,0.492307692307692,0.507692307692308,
0.523076923076923,0.538461538461538,0.553846153846154,0.569230769230769,
0.584615384615384,0.6,0.615384615384615,0.63076923076923,0.646153846153846,
0.661538461538461,0.676923076923076,0.692307692307692,0.707692307692307,
0.723076923076922,0.738461538461538,0.753846153846153,0.769230769230768,
0.784615384615384,0.799999999999999,0.815384615384614,0.83076923076923,
0.846153846153845,0.86153846153846,0.876923076923076,0.892307692307691,
0.907692307692306,0.923076923076922,0.938461538461537,0.953846153846152,
0.969230769230768,0.984615384615383,1.),.UNSPECIFIED.)
CURVE()
GEOMETRIC_REPRESENTATION_ITEM()
RATIONAL_B_SPLINE_CURVE((1.,1.,1.,1.,1.,1.,1.,1.,1.,1.,1.,1.,1.,1.,1.,1.,
1.,1.,1.,1.,1.,1.,1.,1.,1.,1.,1.,1.,1.,1.,1.,1.,1.,1.,1.,1.,1.,1.,1.,1.,
1.,1.,1.,1.,1.,1.,1.,1.,1.,1.,1.,1.,1.,1.,1.,1.,1.,1.,1.,1.,1.,1.,1.,1.,
1.,1.,1.,1.,1.,1.))
REPRESENTATION_ITEM('')
);
#151=(
BOUNDED_CURVE()
B_SPLINE_CURVE(5,(#28264,#28265,#28266,#28267,#28268,#28269,#28270,#28271,
#28272,#28273,#28274,#28275,#28276,#28277,#28278,#28279,#28280,#28281,#28282,
#28283,#28284,#28285,#28286,#28287,#28288,#28289,#28290,#28291,#28292,#28293,
#28294,#28295,#28296,#28297,#28298,#28299,#28300,#28301,#28302,#28303,#28304,
#28305,#28306,#28307,#28308,#28309,#28310,#28311,#28312,#28313,#28314,#28315,
#28316,#28317,#28318,#28319,#28320,#28321,#28322,#28323,#28324,#28325,#28326,
#28327,#28328,#28329,#28330,#28331,#28332,#28333),.UNSPECIFIED.,.F.,.F.)
B_SPLINE_CURVE_WITH_KNOTS((6,1,1,1,1,1,1,1,1,1,1,1,1,1,1,1,1,1,1,1,1,1,
1,1,1,1,1,1,1,1,1,1,1,1,1,1,1,1,1,1,1,1,1,1,1,1,1,1,1,1,1,1,1,1,1,1,1,1,
1,1,1,1,1,1,1,6),(0.,0.0153846153846154,0.0307692307692308,0.0461538461538462,
0.0615384615384615,0.0769230769230769,0.0923076923076923,0.107692307692308,
0.123076923076923,0.138461538461538,0.153846153846154,0.169230769230769,
0.184615384615385,0.2,0.215384615384615,0.230769230769231,0.246153846153846,
0.261538461538462,0.276923076923077,0.292307692307692,0.307692307692308,
0.323076923076923,0.338461538461538,0.353846153846154,0.369230769230769,
0.384615384615385,0.4,0.415384615384615,0.430769230769231,0.446153846153846,
0.461538461538462,0.476923076923077,0.492307692307692,0.507692307692308,
0.523076923076923,0.538461538461538,0.553846153846154,0.569230769230769,
0.584615384615384,0.6,0.615384615384615,0.63076923076923,0.646153846153846,
0.661538461538461,0.676923076923076,0.692307692307692,0.707692307692307,
0.723076923076922,0.738461538461538,0.753846153846153,0.769230769230768,
0.784615384615384,0.799999999999999,0.815384615384614,0.83076923076923,
0.846153846153845,0.86153846153846,0.876923076923076,0.892307692307691,
0.907692307692306,0.923076923076922,0.938461538461537,0.953846153846152,
0.969230769230768,0.984615384615383,1.),.UNSPECIFIED.)
CURVE()
GEOMETRIC_REPRESENTATION_ITEM()
RATIONAL_B_SPLINE_CURVE((1.,1.,1.,1.,1.,1.,1.,1.,1.,1.,1.,1.,1.,1.,1.,1.,
1.,1.,1.,1.,1.,1.,1.,1.,1.,1.,1.,1.,1.,1.,1.,1.,1.,1.,1.,1.,1.,1.,1.,1.,
1.,1.,1.,1.,1.,1.,1.,1.,1.,1.,1.,1.,1.,1.,1.,1.,1.,1.,1.,1.,1.,1.,1.,1.,
1.,1.,1.,1.,1.,1.))
REPRESENTATION_ITEM('')
);
#152=(
BOUNDED_CURVE()
B_SPLINE_CURVE(5,(#28337,#28338,#28339,#28340,#28341,#28342,#28343,#28344,
#28345,#28346,#28347,#28348,#28349,#28350,#28351,#28352,#28353,#28354,#28355,
#28356,#28357,#28358,#28359,#28360,#28361,#28362,#28363,#28364,#28365,#28366,
#28367,#28368,#28369,#28370,#28371,#28372,#28373,#28374,#28375,#28376,#28377,
#28378,#28379,#28380,#28381,#28382,#28383,#28384,#28385,#28386,#28387,#28388,
#28389,#28390,#28391,#28392,#28393,#28394,#28395,#28396,#28397,#28398,#28399,
#28400,#28401,#28402,#28403,#28404,#28405,#28406),.UNSPECIFIED.,.F.,.F.)
B_SPLINE_CURVE_WITH_KNOTS((6,1,1,1,1,1,1,1,1,1,1,1,1,1,1,1,1,1,1,1,1,1,
1,1,1,1,1,1,1,1,1,1,1,1,1,1,1,1,1,1,1,1,1,1,1,1,1,1,1,1,1,1,1,1,1,1,1,1,
1,1,1,1,1,1,1,6),(0.,0.0153846153846154,0.0307692307692308,0.0461538461538462,
0.0615384615384615,0.0769230769230769,0.0923076923076923,0.107692307692308,
0.123076923076923,0.138461538461538,0.153846153846154,0.169230769230769,
0.184615384615385,0.2,0.215384615384615,0.230769230769231,0.246153846153846,
0.261538461538462,0.276923076923077,0.292307692307692,0.307692307692308,
0.323076923076923,0.338461538461538,0.353846153846154,0.369230769230769,
0.384615384615385,0.4,0.415384615384615,0.430769230769231,0.446153846153846,
0.461538461538462,0.476923076923077,0.492307692307692,0.507692307692308,
0.523076923076923,0.538461538461538,0.553846153846154,0.569230769230769,
0.584615384615384,0.6,0.615384615384615,0.63076923076923,0.646153846153846,
0.661538461538461,0.676923076923076,0.692307692307692,0.707692307692307,
0.723076923076922,0.738461538461538,0.753846153846153,0.769230769230768,
0.784615384615384,0.799999999999999,0.815384615384614,0.83076923076923,
0.846153846153845,0.86153846153846,0.876923076923076,0.892307692307691,
0.907692307692306,0.923076923076922,0.938461538461537,0.953846153846152,
0.969230769230768,0.984615384615383,1.),.UNSPECIFIED.)
CURVE()
GEOMETRIC_REPRESENTATION_ITEM()
RATIONAL_B_SPLINE_CURVE((1.,1.,1.,1.,1.,1.,1.,1.,1.,1.,1.,1.,1.,1.,1.,1.,
1.,1.,1.,1.,1.,1.,1.,1.,1.,1.,1.,1.,1.,1.,1.,1.,1.,1.,1.,1.,1.,1.,1.,1.,
1.,1.,1.,1.,1.,1.,1.,1.,1.,1.,1.,1.,1.,1.,1.,1.,1.,1.,1.,1.,1.,1.,1.,1.,
1.,1.,1.,1.,1.,1.))
REPRESENTATION_ITEM('')
);
#153=(
BOUNDED_CURVE()
B_SPLINE_CURVE(5,(#28410,#28411,#28412,#28413,#28414,#28415,#28416,#28417,
#28418,#28419,#28420,#28421,#28422,#28423,#28424,#28425,#28426,#28427,#28428,
#28429,#28430,#28431,#28432,#28433,#28434,#28435,#28436,#28437,#28438,#28439,
#28440,#28441,#28442,#28443,#28444,#28445,#28446,#28447,#28448,#28449,#28450,
#28451,#28452,#28453,#28454,#28455,#28456,#28457,#28458,#28459,#28460,#28461,
#28462,#28463,#28464,#28465,#28466,#28467,#28468,#28469,#28470,#28471,#28472,
#28473,#28474,#28475,#28476,#28477,#28478,#28479),.UNSPECIFIED.,.F.,.F.)
B_SPLINE_CURVE_WITH_KNOTS((6,1,1,1,1,1,1,1,1,1,1,1,1,1,1,1,1,1,1,1,1,1,
1,1,1,1,1,1,1,1,1,1,1,1,1,1,1,1,1,1,1,1,1,1,1,1,1,1,1,1,1,1,1,1,1,1,1,1,
1,1,1,1,1,1,1,6),(0.,0.0153846153846154,0.0307692307692308,0.0461538461538462,
0.0615384615384615,0.0769230769230769,0.0923076923076923,0.107692307692308,
0.123076923076923,0.138461538461538,0.153846153846154,0.169230769230769,
0.184615384615385,0.2,0.215384615384615,0.230769230769231,0.246153846153846,
0.261538461538462,0.276923076923077,0.292307692307692,0.307692307692308,
0.323076923076923,0.338461538461538,0.353846153846154,0.369230769230769,
0.384615384615385,0.4,0.415384615384615,0.430769230769231,0.446153846153846,
0.461538461538462,0.476923076923077,0.492307692307692,0.507692307692308,
0.523076923076923,0.538461538461538,0.553846153846154,0.569230769230769,
0.584615384615384,0.6,0.615384615384615,0.63076923076923,0.646153846153846,
0.661538461538461,0.676923076923076,0.692307692307692,0.707692307692307,
0.723076923076922,0.738461538461538,0.753846153846153,0.769230769230768,
0.784615384615384,0.799999999999999,0.815384615384614,0.83076923076923,
0.846153846153845,0.86153846153846,0.876923076923076,0.892307692307691,
0.907692307692306,0.923076923076922,0.938461538461537,0.953846153846152,
0.969230769230768,0.984615384615383,1.),.UNSPECIFIED.)
CURVE()
GEOMETRIC_REPRESENTATION_ITEM()
RATIONAL_B_SPLINE_CURVE((1.,1.,1.,1.,1.,1.,1.,1.,1.,1.,1.,1.,1.,1.,1.,1.,
1.,1.,1.,1.,1.,1.,1.,1.,1.,1.,1.,1.,1.,1.,1.,1.,1.,1.,1.,1.,1.,1.,1.,1.,
1.,1.,1.,1.,1.,1.,1.,1.,1.,1.,1.,1.,1.,1.,1.,1.,1.,1.,1.,1.,1.,1.,1.,1.,
1.,1.,1.,1.,1.,1.))
REPRESENTATION_ITEM('')
);
#154=(
BOUNDED_CURVE()
B_SPLINE_CURVE(5,(#28483,#28484,#28485,#28486,#28487,#28488,#28489,#28490,
#28491,#28492,#28493,#28494,#28495,#28496,#28497,#28498,#28499,#28500,#28501,
#28502,#28503,#28504,#28505,#28506,#28507,#28508,#28509,#28510,#28511,#28512,
#28513,#28514,#28515,#28516,#28517,#28518,#28519,#28520,#28521,#28522,#28523,
#28524,#28525,#28526,#28527,#28528,#28529,#28530,#28531,#28532,#28533,#28534,
#28535,#28536,#28537,#28538,#28539,#28540,#28541,#28542,#28543,#28544,#28545,
#28546,#28547,#28548,#28549,#28550,#28551,#28552),.UNSPECIFIED.,.F.,.F.)
B_SPLINE_CURVE_WITH_KNOTS((6,1,1,1,1,1,1,1,1,1,1,1,1,1,1,1,1,1,1,1,1,1,
1,1,1,1,1,1,1,1,1,1,1,1,1,1,1,1,1,1,1,1,1,1,1,1,1,1,1,1,1,1,1,1,1,1,1,1,
1,1,1,1,1,1,1,6),(0.,0.0153846153846154,0.0307692307692308,0.0461538461538462,
0.0615384615384615,0.0769230769230769,0.0923076923076923,0.107692307692308,
0.123076923076923,0.138461538461538,0.153846153846154,0.169230769230769,
0.184615384615385,0.2,0.215384615384615,0.230769230769231,0.246153846153846,
0.261538461538462,0.276923076923077,0.292307692307692,0.307692307692308,
0.323076923076923,0.338461538461538,0.353846153846154,0.369230769230769,
0.384615384615385,0.4,0.415384615384615,0.430769230769231,0.446153846153846,
0.461538461538462,0.476923076923077,0.492307692307692,0.507692307692308,
0.523076923076923,0.538461538461538,0.553846153846154,0.569230769230769,
0.584615384615384,0.6,0.615384615384615,0.63076923076923,0.646153846153846,
0.661538461538461,0.676923076923076,0.692307692307692,0.707692307692307,
0.723076923076922,0.738461538461538,0.753846153846153,0.769230769230768,
0.784615384615384,0.799999999999999,0.815384615384614,0.83076923076923,
0.846153846153845,0.86153846153846,0.876923076923076,0.892307692307691,
0.907692307692306,0.923076923076922,0.938461538461537,0.953846153846152,
0.969230769230768,0.984615384615383,1.),.UNSPECIFIED.)
CURVE()
GEOMETRIC_REPRESENTATION_ITEM()
RATIONAL_B_SPLINE_CURVE((1.,1.,1.,1.,1.,1.,1.,1.,1.,1.,1.,1.,1.,1.,1.,1.,
1.,1.,1.,1.,1.,1.,1.,1.,1.,1.,1.,1.,1.,1.,1.,1.,1.,1.,1.,1.,1.,1.,1.,1.,
1.,1.,1.,1.,1.,1.,1.,1.,1.,1.,1.,1.,1.,1.,1.,1.,1.,1.,1.,1.,1.,1.,1.,1.,
1.,1.,1.,1.,1.,1.))
REPRESENTATION_ITEM('')
);
#155=(
BOUNDED_CURVE()
B_SPLINE_CURVE(5,(#28556,#28557,#28558,#28559,#28560,#28561,#28562,#28563,
#28564,#28565,#28566,#28567,#28568,#28569,#28570,#28571,#28572,#28573,#28574,
#28575,#28576,#28577,#28578,#28579,#28580,#28581,#28582,#28583,#28584,#28585,
#28586,#28587,#28588,#28589,#28590,#28591,#28592,#28593,#28594,#28595,#28596,
#28597,#28598,#28599,#28600,#28601,#28602,#28603,#28604,#28605,#28606,#28607,
#28608,#28609,#28610,#28611,#28612,#28613,#28614,#28615,#28616,#28617,#28618,
#28619,#28620,#28621,#28622,#28623,#28624,#28625),.UNSPECIFIED.,.F.,.F.)
B_SPLINE_CURVE_WITH_KNOTS((6,1,1,1,1,1,1,1,1,1,1,1,1,1,1,1,1,1,1,1,1,1,
1,1,1,1,1,1,1,1,1,1,1,1,1,1,1,1,1,1,1,1,1,1,1,1,1,1,1,1,1,1,1,1,1,1,1,1,
1,1,1,1,1,1,1,6),(0.,0.0153846153846154,0.0307692307692308,0.0461538461538462,
0.0615384615384615,0.0769230769230769,0.0923076923076923,0.107692307692308,
0.123076923076923,0.138461538461538,0.153846153846154,0.169230769230769,
0.184615384615385,0.2,0.215384615384615,0.230769230769231,0.246153846153846,
0.261538461538462,0.276923076923077,0.292307692307692,0.307692307692308,
0.323076923076923,0.338461538461538,0.353846153846154,0.369230769230769,
0.384615384615385,0.4,0.415384615384615,0.430769230769231,0.446153846153846,
0.461538461538462,0.476923076923077,0.492307692307692,0.507692307692308,
0.523076923076923,0.538461538461538,0.553846153846154,0.569230769230769,
0.584615384615384,0.6,0.615384615384615,0.63076923076923,0.646153846153846,
0.661538461538461,0.676923076923076,0.692307692307692,0.707692307692307,
0.723076923076922,0.738461538461538,0.753846153846153,0.769230769230768,
0.784615384615384,0.799999999999999,0.815384615384614,0.83076923076923,
0.846153846153845,0.86153846153846,0.876923076923076,0.892307692307691,
0.907692307692306,0.923076923076922,0.938461538461537,0.953846153846152,
0.969230769230768,0.984615384615383,1.),.UNSPECIFIED.)
CURVE()
GEOMETRIC_REPRESENTATION_ITEM()
RATIONAL_B_SPLINE_CURVE((1.,1.,1.,1.,1.,1.,1.,1.,1.,1.,1.,1.,1.,1.,1.,1.,
1.,1.,1.,1.,1.,1.,1.,1.,1.,1.,1.,1.,1.,1.,1.,1.,1.,1.,1.,1.,1.,1.,1.,1.,
1.,1.,1.,1.,1.,1.,1.,1.,1.,1.,1.,1.,1.,1.,1.,1.,1.,1.,1.,1.,1.,1.,1.,1.,
1.,1.,1.,1.,1.,1.))
REPRESENTATION_ITEM('')
);
#156=(
BOUNDED_CURVE()
B_SPLINE_CURVE(5,(#28629,#28630,#28631,#28632,#28633,#28634,#28635,#28636,
#28637,#28638,#28639,#28640,#28641,#28642,#28643,#28644,#28645,#28646,#28647,
#28648,#28649,#28650,#28651,#28652,#28653,#28654,#28655,#28656,#28657,#28658,
#28659,#28660,#28661,#28662,#28663,#28664,#28665,#28666,#28667,#28668,#28669,
#28670,#28671,#28672,#28673,#28674,#28675,#28676,#28677,#28678,#28679,#28680,
#28681,#28682,#28683,#28684,#28685,#28686,#28687,#28688,#28689,#28690,#28691,
#28692,#28693,#28694,#28695,#28696,#28697,#28698),.UNSPECIFIED.,.F.,.F.)
B_SPLINE_CURVE_WITH_KNOTS((6,1,1,1,1,1,1,1,1,1,1,1,1,1,1,1,1,1,1,1,1,1,
1,1,1,1,1,1,1,1,1,1,1,1,1,1,1,1,1,1,1,1,1,1,1,1,1,1,1,1,1,1,1,1,1,1,1,1,
1,1,1,1,1,1,1,6),(0.,0.0153846153846154,0.0307692307692308,0.0461538461538462,
0.0615384615384615,0.0769230769230769,0.0923076923076923,0.107692307692308,
0.123076923076923,0.138461538461538,0.153846153846154,0.169230769230769,
0.184615384615385,0.2,0.215384615384615,0.230769230769231,0.246153846153846,
0.261538461538462,0.276923076923077,0.292307692307692,0.307692307692308,
0.323076923076923,0.338461538461538,0.353846153846154,0.369230769230769,
0.384615384615385,0.4,0.415384615384615,0.430769230769231,0.446153846153846,
0.461538461538462,0.476923076923077,0.492307692307692,0.507692307692308,
0.523076923076923,0.538461538461538,0.553846153846154,0.569230769230769,
0.584615384615384,0.6,0.615384615384615,0.63076923076923,0.646153846153846,
0.661538461538461,0.676923076923076,0.692307692307692,0.707692307692307,
0.723076923076922,0.738461538461538,0.753846153846153,0.769230769230768,
0.784615384615384,0.799999999999999,0.815384615384614,0.83076923076923,
0.846153846153845,0.86153846153846,0.876923076923076,0.892307692307691,
0.907692307692306,0.923076923076922,0.938461538461537,0.953846153846152,
0.969230769230768,0.984615384615383,1.),.UNSPECIFIED.)
CURVE()
GEOMETRIC_REPRESENTATION_ITEM()
RATIONAL_B_SPLINE_CURVE((1.,1.,1.,1.,1.,1.,1.,1.,1.,1.,1.,1.,1.,1.,1.,1.,
1.,1.,1.,1.,1.,1.,1.,1.,1.,1.,1.,1.,1.,1.,1.,1.,1.,1.,1.,1.,1.,1.,1.,1.,
1.,1.,1.,1.,1.,1.,1.,1.,1.,1.,1.,1.,1.,1.,1.,1.,1.,1.,1.,1.,1.,1.,1.,1.,
1.,1.,1.,1.,1.,1.))
REPRESENTATION_ITEM('')
);
#157=(
BOUNDED_CURVE()
B_SPLINE_CURVE(5,(#28702,#28703,#28704,#28705,#28706,#28707,#28708,#28709,
#28710,#28711,#28712,#28713,#28714,#28715,#28716,#28717,#28718,#28719,#28720,
#28721,#28722,#28723,#28724,#28725,#28726,#28727,#28728,#28729,#28730,#28731,
#28732,#28733,#28734,#28735,#28736,#28737,#28738,#28739,#28740,#28741,#28742,
#28743,#28744,#28745,#28746,#28747,#28748,#28749,#28750,#28751,#28752,#28753,
#28754,#28755,#28756,#28757,#28758,#28759,#28760,#28761,#28762,#28763,#28764,
#28765,#28766,#28767,#28768,#28769,#28770,#28771),.UNSPECIFIED.,.F.,.F.)
B_SPLINE_CURVE_WITH_KNOTS((6,1,1,1,1,1,1,1,1,1,1,1,1,1,1,1,1,1,1,1,1,1,
1,1,1,1,1,1,1,1,1,1,1,1,1,1,1,1,1,1,1,1,1,1,1,1,1,1,1,1,1,1,1,1,1,1,1,1,
1,1,1,1,1,1,1,6),(0.,0.0153846153846154,0.0307692307692308,0.0461538461538462,
0.0615384615384615,0.0769230769230769,0.0923076923076923,0.107692307692308,
0.123076923076923,0.138461538461538,0.153846153846154,0.169230769230769,
0.184615384615385,0.2,0.215384615384615,0.230769230769231,0.246153846153846,
0.261538461538462,0.276923076923077,0.292307692307692,0.307692307692308,
0.323076923076923,0.338461538461538,0.353846153846154,0.369230769230769,
0.384615384615385,0.4,0.415384615384615,0.430769230769231,0.446153846153846,
0.461538461538462,0.476923076923077,0.492307692307692,0.507692307692308,
0.523076923076923,0.538461538461538,0.553846153846154,0.569230769230769,
0.584615384615384,0.6,0.615384615384615,0.63076923076923,0.646153846153846,
0.661538461538461,0.676923076923076,0.692307692307692,0.707692307692307,
0.723076923076922,0.738461538461538,0.753846153846153,0.769230769230768,
0.784615384615384,0.799999999999999,0.815384615384614,0.83076923076923,
0.846153846153845,0.86153846153846,0.876923076923076,0.892307692307691,
0.907692307692306,0.923076923076922,0.938461538461537,0.953846153846152,
0.969230769230768,0.984615384615383,1.),.UNSPECIFIED.)
CURVE()
GEOMETRIC_REPRESENTATION_ITEM()
RATIONAL_B_SPLINE_CURVE((1.,1.,1.,1.,1.,1.,1.,1.,1.,1.,1.,1.,1.,1.,1.,1.,
1.,1.,1.,1.,1.,1.,1.,1.,1.,1.,1.,1.,1.,1.,1.,1.,1.,1.,1.,1.,1.,1.,1.,1.,
1.,1.,1.,1.,1.,1.,1.,1.,1.,1.,1.,1.,1.,1.,1.,1.,1.,1.,1.,1.,1.,1.,1.,1.,
1.,1.,1.,1.,1.,1.))
REPRESENTATION_ITEM('')
);
#158=(
BOUNDED_CURVE()
B_SPLINE_CURVE(5,(#28775,#28776,#28777,#28778,#28779,#28780,#28781,#28782,
#28783,#28784,#28785,#28786,#28787,#28788,#28789,#28790,#28791,#28792,#28793,
#28794,#28795,#28796,#28797,#28798,#28799,#28800,#28801,#28802,#28803,#28804,
#28805,#28806,#28807,#28808,#28809,#28810,#28811,#28812,#28813,#28814,#28815,
#28816,#28817,#28818,#28819,#28820,#28821,#28822,#28823,#28824,#28825,#28826,
#28827,#28828,#28829,#28830,#28831,#28832,#28833,#28834,#28835,#28836,#28837,
#28838,#28839,#28840,#28841,#28842,#28843,#28844),.UNSPECIFIED.,.F.,.F.)
B_SPLINE_CURVE_WITH_KNOTS((6,1,1,1,1,1,1,1,1,1,1,1,1,1,1,1,1,1,1,1,1,1,
1,1,1,1,1,1,1,1,1,1,1,1,1,1,1,1,1,1,1,1,1,1,1,1,1,1,1,1,1,1,1,1,1,1,1,1,
1,1,1,1,1,1,1,6),(0.,0.0153846153846154,0.0307692307692308,0.0461538461538462,
0.0615384615384615,0.0769230769230769,0.0923076923076923,0.107692307692308,
0.123076923076923,0.138461538461538,0.153846153846154,0.169230769230769,
0.184615384615385,0.2,0.215384615384615,0.230769230769231,0.246153846153846,
0.261538461538462,0.276923076923077,0.292307692307692,0.307692307692308,
0.323076923076923,0.338461538461538,0.353846153846154,0.369230769230769,
0.384615384615385,0.4,0.415384615384615,0.430769230769231,0.446153846153846,
0.461538461538462,0.476923076923077,0.492307692307692,0.507692307692308,
0.523076923076923,0.538461538461538,0.553846153846154,0.569230769230769,
0.584615384615384,0.6,0.615384615384615,0.63076923076923,0.646153846153846,
0.661538461538461,0.676923076923076,0.692307692307692,0.707692307692307,
0.723076923076922,0.738461538461538,0.753846153846153,0.769230769230768,
0.784615384615384,0.799999999999999,0.815384615384614,0.83076923076923,
0.846153846153845,0.86153846153846,0.876923076923076,0.892307692307691,
0.907692307692306,0.923076923076922,0.938461538461537,0.953846153846152,
0.969230769230768,0.984615384615383,1.),.UNSPECIFIED.)
CURVE()
GEOMETRIC_REPRESENTATION_ITEM()
RATIONAL_B_SPLINE_CURVE((1.,1.,1.,1.,1.,1.,1.,1.,1.,1.,1.,1.,1.,1.,1.,1.,
1.,1.,1.,1.,1.,1.,1.,1.,1.,1.,1.,1.,1.,1.,1.,1.,1.,1.,1.,1.,1.,1.,1.,1.,
1.,1.,1.,1.,1.,1.,1.,1.,1.,1.,1.,1.,1.,1.,1.,1.,1.,1.,1.,1.,1.,1.,1.,1.,
1.,1.,1.,1.,1.,1.))
REPRESENTATION_ITEM('')
);
#159=(
BOUNDED_CURVE()
B_SPLINE_CURVE(5,(#28848,#28849,#28850,#28851,#28852,#28853,#28854,#28855,
#28856,#28857,#28858,#28859,#28860,#28861,#28862,#28863,#28864,#28865,#28866,
#28867,#28868,#28869,#28870,#28871,#28872,#28873,#28874,#28875,#28876,#28877,
#28878,#28879,#28880,#28881,#28882,#28883,#28884,#28885,#28886,#28887,#28888,
#28889,#28890,#28891,#28892,#28893,#28894,#28895,#28896,#28897,#28898,#28899,
#28900,#28901,#28902,#28903,#28904,#28905,#28906,#28907,#28908,#28909,#28910,
#28911,#28912,#28913,#28914,#28915,#28916,#28917),.UNSPECIFIED.,.F.,.F.)
B_SPLINE_CURVE_WITH_KNOTS((6,1,1,1,1,1,1,1,1,1,1,1,1,1,1,1,1,1,1,1,1,1,
1,1,1,1,1,1,1,1,1,1,1,1,1,1,1,1,1,1,1,1,1,1,1,1,1,1,1,1,1,1,1,1,1,1,1,1,
1,1,1,1,1,1,1,6),(0.,0.0153846153846154,0.0307692307692308,0.0461538461538462,
0.0615384615384615,0.0769230769230769,0.0923076923076923,0.107692307692308,
0.123076923076923,0.138461538461538,0.153846153846154,0.169230769230769,
0.184615384615385,0.2,0.215384615384615,0.230769230769231,0.246153846153846,
0.261538461538462,0.276923076923077,0.292307692307692,0.307692307692308,
0.323076923076923,0.338461538461538,0.353846153846154,0.369230769230769,
0.384615384615385,0.4,0.415384615384615,0.430769230769231,0.446153846153846,
0.461538461538462,0.476923076923077,0.492307692307692,0.507692307692308,
0.523076923076923,0.538461538461538,0.553846153846154,0.569230769230769,
0.584615384615384,0.6,0.615384615384615,0.63076923076923,0.646153846153846,
0.661538461538461,0.676923076923076,0.692307692307692,0.707692307692307,
0.723076923076922,0.738461538461538,0.753846153846153,0.769230769230768,
0.784615384615384,0.799999999999999,0.815384615384614,0.83076923076923,
0.846153846153845,0.86153846153846,0.876923076923076,0.892307692307691,
0.907692307692306,0.923076923076922,0.938461538461537,0.953846153846152,
0.969230769230768,0.984615384615383,1.),.UNSPECIFIED.)
CURVE()
GEOMETRIC_REPRESENTATION_ITEM()
RATIONAL_B_SPLINE_CURVE((1.,1.,1.,1.,1.,1.,1.,1.,1.,1.,1.,1.,1.,1.,1.,1.,
1.,1.,1.,1.,1.,1.,1.,1.,1.,1.,1.,1.,1.,1.,1.,1.,1.,1.,1.,1.,1.,1.,1.,1.,
1.,1.,1.,1.,1.,1.,1.,1.,1.,1.,1.,1.,1.,1.,1.,1.,1.,1.,1.,1.,1.,1.,1.,1.,
1.,1.,1.,1.,1.,1.))
REPRESENTATION_ITEM('')
);
#160=(
BOUNDED_CURVE()
B_SPLINE_CURVE(5,(#28921,#28922,#28923,#28924,#28925,#28926,#28927,#28928,
#28929,#28930,#28931,#28932,#28933,#28934,#28935,#28936,#28937,#28938,#28939,
#28940,#28941,#28942,#28943,#28944,#28945,#28946,#28947,#28948,#28949,#28950,
#28951,#28952,#28953,#28954,#28955,#28956,#28957,#28958,#28959,#28960,#28961,
#28962,#28963,#28964,#28965,#28966,#28967,#28968,#28969,#28970,#28971,#28972,
#28973,#28974,#28975,#28976,#28977,#28978,#28979,#28980,#28981,#28982,#28983,
#28984,#28985,#28986,#28987,#28988,#28989,#28990),.UNSPECIFIED.,.F.,.F.)
B_SPLINE_CURVE_WITH_KNOTS((6,1,1,1,1,1,1,1,1,1,1,1,1,1,1,1,1,1,1,1,1,1,
1,1,1,1,1,1,1,1,1,1,1,1,1,1,1,1,1,1,1,1,1,1,1,1,1,1,1,1,1,1,1,1,1,1,1,1,
1,1,1,1,1,1,1,6),(0.,0.0153846153846154,0.0307692307692308,0.0461538461538462,
0.0615384615384615,0.0769230769230769,0.0923076923076923,0.107692307692308,
0.123076923076923,0.138461538461538,0.153846153846154,0.169230769230769,
0.184615384615385,0.2,0.215384615384615,0.230769230769231,0.246153846153846,
0.261538461538462,0.276923076923077,0.292307692307692,0.307692307692308,
0.323076923076923,0.338461538461538,0.353846153846154,0.369230769230769,
0.384615384615385,0.4,0.415384615384615,0.430769230769231,0.446153846153846,
0.461538461538462,0.476923076923077,0.492307692307692,0.507692307692308,
0.523076923076923,0.538461538461538,0.553846153846154,0.569230769230769,
0.584615384615384,0.6,0.615384615384615,0.63076923076923,0.646153846153846,
0.661538461538461,0.676923076923076,0.692307692307692,0.707692307692307,
0.723076923076922,0.738461538461538,0.753846153846153,0.769230769230768,
0.784615384615384,0.799999999999999,0.815384615384614,0.83076923076923,
0.846153846153845,0.86153846153846,0.876923076923076,0.892307692307691,
0.907692307692306,0.923076923076922,0.938461538461537,0.953846153846152,
0.969230769230768,0.984615384615383,1.),.UNSPECIFIED.)
CURVE()
GEOMETRIC_REPRESENTATION_ITEM()
RATIONAL_B_SPLINE_CURVE((1.,1.,1.,1.,1.,1.,1.,1.,1.,1.,1.,1.,1.,1.,1.,1.,
1.,1.,1.,1.,1.,1.,1.,1.,1.,1.,1.,1.,1.,1.,1.,1.,1.,1.,1.,1.,1.,1.,1.,1.,
1.,1.,1.,1.,1.,1.,1.,1.,1.,1.,1.,1.,1.,1.,1.,1.,1.,1.,1.,1.,1.,1.,1.,1.,
1.,1.,1.,1.,1.,1.))
REPRESENTATION_ITEM('')
);
#161=(
BOUNDED_CURVE()
B_SPLINE_CURVE(5,(#28994,#28995,#28996,#28997,#28998,#28999,#29000,#29001,
#29002,#29003,#29004,#29005,#29006,#29007,#29008,#29009,#29010,#29011,#29012,
#29013,#29014,#29015,#29016,#29017,#29018,#29019,#29020,#29021,#29022,#29023,
#29024,#29025,#29026,#29027,#29028,#29029,#29030,#29031,#29032,#29033,#29034,
#29035,#29036,#29037,#29038,#29039,#29040,#29041,#29042,#29043,#29044,#29045,
#29046,#29047,#29048,#29049,#29050,#29051,#29052,#29053,#29054,#29055,#29056,
#29057,#29058,#29059,#29060,#29061,#29062,#29063),.UNSPECIFIED.,.F.,.F.)
B_SPLINE_CURVE_WITH_KNOTS((6,1,1,1,1,1,1,1,1,1,1,1,1,1,1,1,1,1,1,1,1,1,
1,1,1,1,1,1,1,1,1,1,1,1,1,1,1,1,1,1,1,1,1,1,1,1,1,1,1,1,1,1,1,1,1,1,1,1,
1,1,1,1,1,1,1,6),(0.,0.0153846153846154,0.0307692307692308,0.0461538461538462,
0.0615384615384615,0.0769230769230769,0.0923076923076923,0.107692307692308,
0.123076923076923,0.138461538461538,0.153846153846154,0.169230769230769,
0.184615384615385,0.2,0.215384615384615,0.230769230769231,0.246153846153846,
0.261538461538462,0.276923076923077,0.292307692307692,0.307692307692308,
0.323076923076923,0.338461538461538,0.353846153846154,0.369230769230769,
0.384615384615385,0.4,0.415384615384615,0.430769230769231,0.446153846153846,
0.461538461538462,0.476923076923077,0.492307692307692,0.507692307692308,
0.523076923076923,0.538461538461538,0.553846153846154,0.569230769230769,
0.584615384615384,0.6,0.615384615384615,0.63076923076923,0.646153846153846,
0.661538461538461,0.676923076923076,0.692307692307692,0.707692307692307,
0.723076923076922,0.738461538461538,0.753846153846153,0.769230769230768,
0.784615384615384,0.799999999999999,0.815384615384614,0.83076923076923,
0.846153846153845,0.86153846153846,0.876923076923076,0.892307692307691,
0.907692307692306,0.923076923076922,0.938461538461537,0.953846153846152,
0.969230769230768,0.984615384615383,1.),.UNSPECIFIED.)
CURVE()
GEOMETRIC_REPRESENTATION_ITEM()
RATIONAL_B_SPLINE_CURVE((1.,1.,1.,1.,1.,1.,1.,1.,1.,1.,1.,1.,1.,1.,1.,1.,
1.,1.,1.,1.,1.,1.,1.,1.,1.,1.,1.,1.,1.,1.,1.,1.,1.,1.,1.,1.,1.,1.,1.,1.,
1.,1.,1.,1.,1.,1.,1.,1.,1.,1.,1.,1.,1.,1.,1.,1.,1.,1.,1.,1.,1.,1.,1.,1.,
1.,1.,1.,1.,1.,1.))
REPRESENTATION_ITEM('')
);
#162=(
BOUNDED_CURVE()
B_SPLINE_CURVE(5,(#29067,#29068,#29069,#29070,#29071,#29072,#29073,#29074,
#29075,#29076,#29077,#29078,#29079,#29080,#29081,#29082,#29083,#29084,#29085,
#29086,#29087,#29088,#29089,#29090,#29091,#29092,#29093,#29094,#29095,#29096,
#29097,#29098,#29099,#29100,#29101,#29102,#29103,#29104,#29105,#29106,#29107,
#29108,#29109,#29110,#29111,#29112,#29113,#29114,#29115,#29116,#29117,#29118,
#29119,#29120,#29121,#29122,#29123,#29124,#29125,#29126,#29127,#29128,#29129,
#29130,#29131,#29132,#29133,#29134,#29135,#29136),.UNSPECIFIED.,.F.,.F.)
B_SPLINE_CURVE_WITH_KNOTS((6,1,1,1,1,1,1,1,1,1,1,1,1,1,1,1,1,1,1,1,1,1,
1,1,1,1,1,1,1,1,1,1,1,1,1,1,1,1,1,1,1,1,1,1,1,1,1,1,1,1,1,1,1,1,1,1,1,1,
1,1,1,1,1,1,1,6),(0.,0.0153846153846154,0.0307692307692308,0.0461538461538462,
0.0615384615384615,0.0769230769230769,0.0923076923076923,0.107692307692308,
0.123076923076923,0.138461538461538,0.153846153846154,0.169230769230769,
0.184615384615385,0.2,0.215384615384615,0.230769230769231,0.246153846153846,
0.261538461538462,0.276923076923077,0.292307692307692,0.307692307692308,
0.323076923076923,0.338461538461538,0.353846153846154,0.369230769230769,
0.384615384615385,0.4,0.415384615384615,0.430769230769231,0.446153846153846,
0.461538461538462,0.476923076923077,0.492307692307692,0.507692307692308,
0.523076923076923,0.538461538461538,0.553846153846154,0.569230769230769,
0.584615384615384,0.6,0.615384615384615,0.63076923076923,0.646153846153846,
0.661538461538461,0.676923076923076,0.692307692307692,0.707692307692307,
0.723076923076922,0.738461538461538,0.753846153846153,0.769230769230768,
0.784615384615384,0.799999999999999,0.815384615384614,0.83076923076923,
0.846153846153845,0.86153846153846,0.876923076923076,0.892307692307691,
0.907692307692306,0.923076923076922,0.938461538461537,0.953846153846152,
0.969230769230768,0.984615384615383,1.),.UNSPECIFIED.)
CURVE()
GEOMETRIC_REPRESENTATION_ITEM()
RATIONAL_B_SPLINE_CURVE((1.,1.,1.,1.,1.,1.,1.,1.,1.,1.,1.,1.,1.,1.,1.,1.,
1.,1.,1.,1.,1.,1.,1.,1.,1.,1.,1.,1.,1.,1.,1.,1.,1.,1.,1.,1.,1.,1.,1.,1.,
1.,1.,1.,1.,1.,1.,1.,1.,1.,1.,1.,1.,1.,1.,1.,1.,1.,1.,1.,1.,1.,1.,1.,1.,
1.,1.,1.,1.,1.,1.))
REPRESENTATION_ITEM('')
);
#163=(
BOUNDED_CURVE()
B_SPLINE_CURVE(5,(#29140,#29141,#29142,#29143,#29144,#29145,#29146,#29147,
#29148,#29149,#29150,#29151,#29152,#29153,#29154,#29155,#29156,#29157,#29158,
#29159,#29160,#29161,#29162,#29163,#29164,#29165,#29166,#29167,#29168,#29169,
#29170,#29171,#29172,#29173,#29174,#29175,#29176,#29177,#29178,#29179,#29180,
#29181,#29182,#29183,#29184,#29185,#29186,#29187,#29188,#29189,#29190,#29191,
#29192,#29193,#29194,#29195,#29196,#29197,#29198,#29199,#29200,#29201,#29202,
#29203,#29204,#29205,#29206,#29207,#29208,#29209),.UNSPECIFIED.,.F.,.F.)
B_SPLINE_CURVE_WITH_KNOTS((6,1,1,1,1,1,1,1,1,1,1,1,1,1,1,1,1,1,1,1,1,1,
1,1,1,1,1,1,1,1,1,1,1,1,1,1,1,1,1,1,1,1,1,1,1,1,1,1,1,1,1,1,1,1,1,1,1,1,
1,1,1,1,1,1,1,6),(0.,0.0153846153846154,0.0307692307692308,0.0461538461538462,
0.0615384615384615,0.0769230769230769,0.0923076923076923,0.107692307692308,
0.123076923076923,0.138461538461538,0.153846153846154,0.169230769230769,
0.184615384615385,0.2,0.215384615384615,0.230769230769231,0.246153846153846,
0.261538461538462,0.276923076923077,0.292307692307692,0.307692307692308,
0.323076923076923,0.338461538461538,0.353846153846154,0.369230769230769,
0.384615384615385,0.4,0.415384615384615,0.430769230769231,0.446153846153846,
0.461538461538462,0.476923076923077,0.492307692307692,0.507692307692308,
0.523076923076923,0.538461538461538,0.553846153846154,0.569230769230769,
0.584615384615384,0.6,0.615384615384615,0.63076923076923,0.646153846153846,
0.661538461538461,0.676923076923076,0.692307692307692,0.707692307692307,
0.723076923076922,0.738461538461538,0.753846153846153,0.769230769230768,
0.784615384615384,0.799999999999999,0.815384615384614,0.83076923076923,
0.846153846153845,0.86153846153846,0.876923076923076,0.892307692307691,
0.907692307692306,0.923076923076922,0.938461538461537,0.953846153846152,
0.969230769230768,0.984615384615383,1.),.UNSPECIFIED.)
CURVE()
GEOMETRIC_REPRESENTATION_ITEM()
RATIONAL_B_SPLINE_CURVE((1.,1.,1.,1.,1.,1.,1.,1.,1.,1.,1.,1.,1.,1.,1.,1.,
1.,1.,1.,1.,1.,1.,1.,1.,1.,1.,1.,1.,1.,1.,1.,1.,1.,1.,1.,1.,1.,1.,1.,1.,
1.,1.,1.,1.,1.,1.,1.,1.,1.,1.,1.,1.,1.,1.,1.,1.,1.,1.,1.,1.,1.,1.,1.,1.,
1.,1.,1.,1.,1.,1.))
REPRESENTATION_ITEM('')
);
#164=(
BOUNDED_CURVE()
B_SPLINE_CURVE(5,(#29213,#29214,#29215,#29216,#29217,#29218,#29219,#29220,
#29221,#29222,#29223,#29224,#29225,#29226,#29227,#29228,#29229,#29230,#29231,
#29232,#29233,#29234,#29235,#29236,#29237,#29238,#29239,#29240,#29241,#29242,
#29243,#29244,#29245,#29246,#29247,#29248,#29249,#29250,#29251,#29252,#29253,
#29254,#29255,#29256,#29257,#29258,#29259,#29260,#29261,#29262,#29263,#29264,
#29265,#29266,#29267,#29268,#29269,#29270,#29271,#29272,#29273,#29274,#29275,
#29276,#29277,#29278,#29279,#29280,#29281,#29282),.UNSPECIFIED.,.F.,.F.)
B_SPLINE_CURVE_WITH_KNOTS((6,1,1,1,1,1,1,1,1,1,1,1,1,1,1,1,1,1,1,1,1,1,
1,1,1,1,1,1,1,1,1,1,1,1,1,1,1,1,1,1,1,1,1,1,1,1,1,1,1,1,1,1,1,1,1,1,1,1,
1,1,1,1,1,1,1,6),(0.,0.0153846153846154,0.0307692307692308,0.0461538461538462,
0.0615384615384615,0.0769230769230769,0.0923076923076923,0.107692307692308,
0.123076923076923,0.138461538461538,0.153846153846154,0.169230769230769,
0.184615384615385,0.2,0.215384615384615,0.230769230769231,0.246153846153846,
0.261538461538462,0.276923076923077,0.292307692307692,0.307692307692308,
0.323076923076923,0.338461538461538,0.353846153846154,0.369230769230769,
0.384615384615385,0.4,0.415384615384615,0.430769230769231,0.446153846153846,
0.461538461538462,0.476923076923077,0.492307692307692,0.507692307692308,
0.523076923076923,0.538461538461538,0.553846153846154,0.569230769230769,
0.584615384615384,0.6,0.615384615384615,0.63076923076923,0.646153846153846,
0.661538461538461,0.676923076923076,0.692307692307692,0.707692307692307,
0.723076923076922,0.738461538461538,0.753846153846153,0.769230769230768,
0.784615384615384,0.799999999999999,0.815384615384614,0.83076923076923,
0.846153846153845,0.86153846153846,0.876923076923076,0.892307692307691,
0.907692307692306,0.923076923076922,0.938461538461537,0.953846153846152,
0.969230769230768,0.984615384615383,1.),.UNSPECIFIED.)
CURVE()
GEOMETRIC_REPRESENTATION_ITEM()
RATIONAL_B_SPLINE_CURVE((1.,1.,1.,1.,1.,1.,1.,1.,1.,1.,1.,1.,1.,1.,1.,1.,
1.,1.,1.,1.,1.,1.,1.,1.,1.,1.,1.,1.,1.,1.,1.,1.,1.,1.,1.,1.,1.,1.,1.,1.,
1.,1.,1.,1.,1.,1.,1.,1.,1.,1.,1.,1.,1.,1.,1.,1.,1.,1.,1.,1.,1.,1.,1.,1.,
1.,1.,1.,1.,1.,1.))
REPRESENTATION_ITEM('')
);
#165=(
BOUNDED_CURVE()
B_SPLINE_CURVE(5,(#29286,#29287,#29288,#29289,#29290,#29291,#29292,#29293,
#29294,#29295,#29296,#29297,#29298,#29299,#29300,#29301,#29302,#29303,#29304,
#29305,#29306,#29307,#29308,#29309,#29310,#29311,#29312,#29313,#29314,#29315,
#29316,#29317,#29318,#29319,#29320,#29321,#29322,#29323,#29324,#29325,#29326,
#29327,#29328,#29329,#29330,#29331,#29332,#29333,#29334,#29335,#29336,#29337,
#29338,#29339,#29340,#29341,#29342,#29343,#29344,#29345,#29346,#29347,#29348,
#29349,#29350,#29351,#29352,#29353,#29354,#29355),.UNSPECIFIED.,.F.,.F.)
B_SPLINE_CURVE_WITH_KNOTS((6,1,1,1,1,1,1,1,1,1,1,1,1,1,1,1,1,1,1,1,1,1,
1,1,1,1,1,1,1,1,1,1,1,1,1,1,1,1,1,1,1,1,1,1,1,1,1,1,1,1,1,1,1,1,1,1,1,1,
1,1,1,1,1,1,1,6),(0.,0.0153846153846154,0.0307692307692308,0.0461538461538462,
0.0615384615384615,0.0769230769230769,0.0923076923076923,0.107692307692308,
0.123076923076923,0.138461538461538,0.153846153846154,0.169230769230769,
0.184615384615385,0.2,0.215384615384615,0.230769230769231,0.246153846153846,
0.261538461538462,0.276923076923077,0.292307692307692,0.307692307692308,
0.323076923076923,0.338461538461538,0.353846153846154,0.369230769230769,
0.384615384615385,0.4,0.415384615384615,0.430769230769231,0.446153846153846,
0.461538461538462,0.476923076923077,0.492307692307692,0.507692307692308,
0.523076923076923,0.538461538461538,0.553846153846154,0.569230769230769,
0.584615384615384,0.6,0.615384615384615,0.63076923076923,0.646153846153846,
0.661538461538461,0.676923076923076,0.692307692307692,0.707692307692307,
0.723076923076922,0.738461538461538,0.753846153846153,0.769230769230768,
0.784615384615384,0.799999999999999,0.815384615384614,0.83076923076923,
0.846153846153845,0.86153846153846,0.876923076923076,0.892307692307691,
0.907692307692306,0.923076923076922,0.938461538461537,0.953846153846152,
0.969230769230768,0.984615384615383,1.),.UNSPECIFIED.)
CURVE()
GEOMETRIC_REPRESENTATION_ITEM()
RATIONAL_B_SPLINE_CURVE((1.,1.,1.,1.,1.,1.,1.,1.,1.,1.,1.,1.,1.,1.,1.,1.,
1.,1.,1.,1.,1.,1.,1.,1.,1.,1.,1.,1.,1.,1.,1.,1.,1.,1.,1.,1.,1.,1.,1.,1.,
1.,1.,1.,1.,1.,1.,1.,1.,1.,1.,1.,1.,1.,1.,1.,1.,1.,1.,1.,1.,1.,1.,1.,1.,
1.,1.,1.,1.,1.,1.))
REPRESENTATION_ITEM('')
);
#166=(
BOUNDED_CURVE()
B_SPLINE_CURVE(5,(#29359,#29360,#29361,#29362,#29363,#29364,#29365,#29366,
#29367,#29368,#29369,#29370,#29371,#29372,#29373,#29374,#29375,#29376,#29377,
#29378,#29379,#29380,#29381,#29382,#29383,#29384,#29385,#29386,#29387,#29388,
#29389,#29390,#29391,#29392,#29393,#29394,#29395,#29396,#29397,#29398,#29399,
#29400,#29401,#29402,#29403,#29404,#29405,#29406,#29407,#29408,#29409,#29410,
#29411,#29412,#29413,#29414,#29415,#29416,#29417,#29418,#29419,#29420,#29421,
#29422,#29423,#29424,#29425,#29426,#29427,#29428),.UNSPECIFIED.,.F.,.F.)
B_SPLINE_CURVE_WITH_KNOTS((6,1,1,1,1,1,1,1,1,1,1,1,1,1,1,1,1,1,1,1,1,1,
1,1,1,1,1,1,1,1,1,1,1,1,1,1,1,1,1,1,1,1,1,1,1,1,1,1,1,1,1,1,1,1,1,1,1,1,
1,1,1,1,1,1,1,6),(0.,0.0153846153846154,0.0307692307692308,0.0461538461538462,
0.0615384615384615,0.0769230769230769,0.0923076923076923,0.107692307692308,
0.123076923076923,0.138461538461538,0.153846153846154,0.169230769230769,
0.184615384615385,0.2,0.215384615384615,0.230769230769231,0.246153846153846,
0.261538461538462,0.276923076923077,0.292307692307692,0.307692307692308,
0.323076923076923,0.338461538461538,0.353846153846154,0.369230769230769,
0.384615384615385,0.4,0.415384615384615,0.430769230769231,0.446153846153846,
0.461538461538462,0.476923076923077,0.492307692307692,0.507692307692308,
0.523076923076923,0.538461538461538,0.553846153846154,0.569230769230769,
0.584615384615384,0.6,0.615384615384615,0.63076923076923,0.646153846153846,
0.661538461538461,0.676923076923076,0.692307692307692,0.707692307692307,
0.723076923076922,0.738461538461538,0.753846153846153,0.769230769230768,
0.784615384615384,0.799999999999999,0.815384615384614,0.83076923076923,
0.846153846153845,0.86153846153846,0.876923076923076,0.892307692307691,
0.907692307692306,0.923076923076922,0.938461538461537,0.953846153846152,
0.969230769230768,0.984615384615383,1.),.UNSPECIFIED.)
CURVE()
GEOMETRIC_REPRESENTATION_ITEM()
RATIONAL_B_SPLINE_CURVE((1.,1.,1.,1.,1.,1.,1.,1.,1.,1.,1.,1.,1.,1.,1.,1.,
1.,1.,1.,1.,1.,1.,1.,1.,1.,1.,1.,1.,1.,1.,1.,1.,1.,1.,1.,1.,1.,1.,1.,1.,
1.,1.,1.,1.,1.,1.,1.,1.,1.,1.,1.,1.,1.,1.,1.,1.,1.,1.,1.,1.,1.,1.,1.,1.,
1.,1.,1.,1.,1.,1.))
REPRESENTATION_ITEM('')
);
#167=(
BOUNDED_CURVE()
B_SPLINE_CURVE(5,(#29432,#29433,#29434,#29435,#29436,#29437,#29438,#29439,
#29440,#29441,#29442,#29443,#29444,#29445,#29446,#29447,#29448,#29449,#29450,
#29451,#29452,#29453,#29454,#29455,#29456,#29457,#29458,#29459,#29460,#29461,
#29462,#29463,#29464,#29465,#29466,#29467,#29468,#29469,#29470,#29471,#29472,
#29473,#29474,#29475,#29476,#29477,#29478,#29479,#29480,#29481,#29482,#29483,
#29484,#29485,#29486,#29487,#29488,#29489,#29490,#29491,#29492,#29493,#29494,
#29495,#29496,#29497,#29498,#29499,#29500,#29501),.UNSPECIFIED.,.F.,.F.)
B_SPLINE_CURVE_WITH_KNOTS((6,1,1,1,1,1,1,1,1,1,1,1,1,1,1,1,1,1,1,1,1,1,
1,1,1,1,1,1,1,1,1,1,1,1,1,1,1,1,1,1,1,1,1,1,1,1,1,1,1,1,1,1,1,1,1,1,1,1,
1,1,1,1,1,1,1,6),(0.,0.0153846153846154,0.0307692307692308,0.0461538461538462,
0.0615384615384615,0.0769230769230769,0.0923076923076923,0.107692307692308,
0.123076923076923,0.138461538461538,0.153846153846154,0.169230769230769,
0.184615384615385,0.2,0.215384615384615,0.230769230769231,0.246153846153846,
0.261538461538462,0.276923076923077,0.292307692307692,0.307692307692308,
0.323076923076923,0.338461538461538,0.353846153846154,0.369230769230769,
0.384615384615385,0.4,0.415384615384615,0.430769230769231,0.446153846153846,
0.461538461538462,0.476923076923077,0.492307692307692,0.507692307692308,
0.523076923076923,0.538461538461538,0.553846153846154,0.569230769230769,
0.584615384615384,0.6,0.615384615384615,0.63076923076923,0.646153846153846,
0.661538461538461,0.676923076923076,0.692307692307692,0.707692307692307,
0.723076923076922,0.738461538461538,0.753846153846153,0.769230769230768,
0.784615384615384,0.799999999999999,0.815384615384614,0.83076923076923,
0.846153846153845,0.86153846153846,0.876923076923076,0.892307692307691,
0.907692307692306,0.923076923076922,0.938461538461537,0.953846153846152,
0.969230769230768,0.984615384615383,1.),.UNSPECIFIED.)
CURVE()
GEOMETRIC_REPRESENTATION_ITEM()
RATIONAL_B_SPLINE_CURVE((1.,1.,1.,1.,1.,1.,1.,1.,1.,1.,1.,1.,1.,1.,1.,1.,
1.,1.,1.,1.,1.,1.,1.,1.,1.,1.,1.,1.,1.,1.,1.,1.,1.,1.,1.,1.,1.,1.,1.,1.,
1.,1.,1.,1.,1.,1.,1.,1.,1.,1.,1.,1.,1.,1.,1.,1.,1.,1.,1.,1.,1.,1.,1.,1.,
1.,1.,1.,1.,1.,1.))
REPRESENTATION_ITEM('')
);
#168=(
BOUNDED_CURVE()
B_SPLINE_CURVE(5,(#29505,#29506,#29507,#29508,#29509,#29510,#29511,#29512,
#29513,#29514,#29515,#29516,#29517,#29518,#29519,#29520,#29521,#29522,#29523,
#29524,#29525,#29526,#29527,#29528,#29529,#29530,#29531,#29532,#29533,#29534,
#29535,#29536,#29537,#29538,#29539,#29540,#29541,#29542,#29543,#29544,#29545,
#29546,#29547,#29548,#29549,#29550,#29551,#29552,#29553,#29554,#29555,#29556,
#29557,#29558,#29559,#29560,#29561,#29562,#29563,#29564,#29565,#29566,#29567,
#29568,#29569,#29570,#29571,#29572,#29573,#29574),.UNSPECIFIED.,.F.,.F.)
B_SPLINE_CURVE_WITH_KNOTS((6,1,1,1,1,1,1,1,1,1,1,1,1,1,1,1,1,1,1,1,1,1,
1,1,1,1,1,1,1,1,1,1,1,1,1,1,1,1,1,1,1,1,1,1,1,1,1,1,1,1,1,1,1,1,1,1,1,1,
1,1,1,1,1,1,1,6),(0.,0.0153846153846154,0.0307692307692308,0.0461538461538462,
0.0615384615384615,0.0769230769230769,0.0923076923076923,0.107692307692308,
0.123076923076923,0.138461538461538,0.153846153846154,0.169230769230769,
0.184615384615385,0.2,0.215384615384615,0.230769230769231,0.246153846153846,
0.261538461538462,0.276923076923077,0.292307692307692,0.307692307692308,
0.323076923076923,0.338461538461538,0.353846153846154,0.369230769230769,
0.384615384615385,0.4,0.415384615384615,0.430769230769231,0.446153846153846,
0.461538461538462,0.476923076923077,0.492307692307692,0.507692307692308,
0.523076923076923,0.538461538461538,0.553846153846154,0.569230769230769,
0.584615384615384,0.6,0.615384615384615,0.63076923076923,0.646153846153846,
0.661538461538461,0.676923076923076,0.692307692307692,0.707692307692307,
0.723076923076922,0.738461538461538,0.753846153846153,0.769230769230768,
0.784615384615384,0.799999999999999,0.815384615384614,0.83076923076923,
0.846153846153845,0.86153846153846,0.876923076923076,0.892307692307691,
0.907692307692306,0.923076923076922,0.938461538461537,0.953846153846152,
0.969230769230768,0.984615384615383,1.),.UNSPECIFIED.)
CURVE()
GEOMETRIC_REPRESENTATION_ITEM()
RATIONAL_B_SPLINE_CURVE((1.,1.,1.,1.,1.,1.,1.,1.,1.,1.,1.,1.,1.,1.,1.,1.,
1.,1.,1.,1.,1.,1.,1.,1.,1.,1.,1.,1.,1.,1.,1.,1.,1.,1.,1.,1.,1.,1.,1.,1.,
1.,1.,1.,1.,1.,1.,1.,1.,1.,1.,1.,1.,1.,1.,1.,1.,1.,1.,1.,1.,1.,1.,1.,1.,
1.,1.,1.,1.,1.,1.))
REPRESENTATION_ITEM('')
);
#169=(
BOUNDED_CURVE()
B_SPLINE_CURVE(5,(#29578,#29579,#29580,#29581,#29582,#29583,#29584,#29585,
#29586,#29587,#29588,#29589,#29590,#29591,#29592,#29593,#29594,#29595,#29596,
#29597,#29598,#29599,#29600,#29601,#29602,#29603,#29604,#29605,#29606,#29607,
#29608,#29609,#29610,#29611,#29612,#29613,#29614,#29615,#29616,#29617,#29618,
#29619,#29620,#29621,#29622,#29623,#29624,#29625,#29626,#29627,#29628,#29629,
#29630,#29631,#29632,#29633,#29634,#29635,#29636,#29637,#29638,#29639,#29640,
#29641,#29642,#29643,#29644,#29645,#29646,#29647),.UNSPECIFIED.,.F.,.F.)
B_SPLINE_CURVE_WITH_KNOTS((6,1,1,1,1,1,1,1,1,1,1,1,1,1,1,1,1,1,1,1,1,1,
1,1,1,1,1,1,1,1,1,1,1,1,1,1,1,1,1,1,1,1,1,1,1,1,1,1,1,1,1,1,1,1,1,1,1,1,
1,1,1,1,1,1,1,6),(0.,0.0153846153846154,0.0307692307692308,0.0461538461538462,
0.0615384615384615,0.0769230769230769,0.0923076923076923,0.107692307692308,
0.123076923076923,0.138461538461538,0.153846153846154,0.169230769230769,
0.184615384615385,0.2,0.215384615384615,0.230769230769231,0.246153846153846,
0.261538461538462,0.276923076923077,0.292307692307692,0.307692307692308,
0.323076923076923,0.338461538461538,0.353846153846154,0.369230769230769,
0.384615384615385,0.4,0.415384615384615,0.430769230769231,0.446153846153846,
0.461538461538462,0.476923076923077,0.492307692307692,0.507692307692308,
0.523076923076923,0.538461538461538,0.553846153846154,0.569230769230769,
0.584615384615384,0.6,0.615384615384615,0.63076923076923,0.646153846153846,
0.661538461538461,0.676923076923076,0.692307692307692,0.707692307692307,
0.723076923076922,0.738461538461538,0.753846153846153,0.769230769230768,
0.784615384615384,0.799999999999999,0.815384615384614,0.83076923076923,
0.846153846153845,0.86153846153846,0.876923076923076,0.892307692307691,
0.907692307692306,0.923076923076922,0.938461538461537,0.953846153846152,
0.969230769230768,0.984615384615383,1.),.UNSPECIFIED.)
CURVE()
GEOMETRIC_REPRESENTATION_ITEM()
RATIONAL_B_SPLINE_CURVE((1.,1.,1.,1.,1.,1.,1.,1.,1.,1.,1.,1.,1.,1.,1.,1.,
1.,1.,1.,1.,1.,1.,1.,1.,1.,1.,1.,1.,1.,1.,1.,1.,1.,1.,1.,1.,1.,1.,1.,1.,
1.,1.,1.,1.,1.,1.,1.,1.,1.,1.,1.,1.,1.,1.,1.,1.,1.,1.,1.,1.,1.,1.,1.,1.,
1.,1.,1.,1.,1.,1.))
REPRESENTATION_ITEM('')
);
#170=(
BOUNDED_CURVE()
B_SPLINE_CURVE(5,(#29650,#29651,#29652,#29653,#29654,#29655,#29656,#29657,
#29658,#29659,#29660,#29661,#29662,#29663,#29664,#29665,#29666,#29667,#29668,
#29669,#29670,#29671,#29672,#29673,#29674,#29675,#29676,#29677,#29678,#29679,
#29680,#29681,#29682,#29683,#29684,#29685,#29686,#29687,#29688,#29689,#29690,
#29691,#29692,#29693,#29694,#29695,#29696,#29697,#29698,#29699,#29700,#29701,
#29702,#29703,#29704,#29705,#29706,#29707,#29708,#29709,#29710,#29711,#29712,
#29713,#29714,#29715,#29716,#29717,#29718,#29719),.UNSPECIFIED.,.F.,.F.)
B_SPLINE_CURVE_WITH_KNOTS((6,1,1,1,1,1,1,1,1,1,1,1,1,1,1,1,1,1,1,1,1,1,
1,1,1,1,1,1,1,1,1,1,1,1,1,1,1,1,1,1,1,1,1,1,1,1,1,1,1,1,1,1,1,1,1,1,1,1,
1,1,1,1,1,1,1,6),(0.,0.0153846153846154,0.0307692307692308,0.0461538461538462,
0.0615384615384615,0.0769230769230769,0.0923076923076923,0.107692307692308,
0.123076923076923,0.138461538461538,0.153846153846154,0.169230769230769,
0.184615384615385,0.2,0.215384615384615,0.230769230769231,0.246153846153846,
0.261538461538462,0.276923076923077,0.292307692307692,0.307692307692308,
0.323076923076923,0.338461538461538,0.353846153846154,0.369230769230769,
0.384615384615385,0.4,0.415384615384615,0.430769230769231,0.446153846153846,
0.461538461538462,0.476923076923077,0.492307692307692,0.507692307692308,
0.523076923076923,0.538461538461538,0.553846153846154,0.569230769230769,
0.584615384615384,0.6,0.615384615384615,0.63076923076923,0.646153846153846,
0.661538461538461,0.676923076923076,0.692307692307692,0.707692307692307,
0.723076923076922,0.738461538461538,0.753846153846153,0.769230769230768,
0.784615384615384,0.799999999999999,0.815384615384614,0.83076923076923,
0.846153846153845,0.86153846153846,0.876923076923076,0.892307692307691,
0.907692307692306,0.923076923076922,0.938461538461537,0.953846153846152,
0.969230769230768,0.984615384615383,1.),.UNSPECIFIED.)
CURVE()
GEOMETRIC_REPRESENTATION_ITEM()
RATIONAL_B_SPLINE_CURVE((1.,1.,1.,1.,1.,1.,1.,1.,1.,1.,1.,1.,1.,1.,1.,1.,
1.,1.,1.,1.,1.,1.,1.,1.,1.,1.,1.,1.,1.,1.,1.,1.,1.,1.,1.,1.,1.,1.,1.,1.,
1.,1.,1.,1.,1.,1.,1.,1.,1.,1.,1.,1.,1.,1.,1.,1.,1.,1.,1.,1.,1.,1.,1.,1.,
1.,1.,1.,1.,1.,1.))
REPRESENTATION_ITEM('')
);
#171=(
BOUNDED_CURVE()
B_SPLINE_CURVE(5,(#29873,#29874,#29875,#29876,#29877,#29878,#29879,#29880,
#29881,#29882,#29883,#29884,#29885,#29886,#29887,#29888,#29889,#29890,#29891,
#29892,#29893,#29894,#29895,#29896,#29897,#29898,#29899,#29900,#29901,#29902,
#29903,#29904,#29905,#29906,#29907,#29908,#29909,#29910,#29911,#29912,#29913,
#29914,#29915,#29916,#29917,#29918,#29919,#29920,#29921,#29922,#29923,#29924,
#29925,#29926,#29927,#29928,#29929,#29930,#29931,#29932,#29933,#29934,#29935,
#29936,#29937,#29938,#29939,#29940,#29941,#29942),.UNSPECIFIED.,.F.,.F.)
B_SPLINE_CURVE_WITH_KNOTS((6,1,1,1,1,1,1,1,1,1,1,1,1,1,1,1,1,1,1,1,1,1,
1,1,1,1,1,1,1,1,1,1,1,1,1,1,1,1,1,1,1,1,1,1,1,1,1,1,1,1,1,1,1,1,1,1,1,1,
1,1,1,1,1,1,1,6),(-1.,-0.984615384615383,-0.969230769230768,-0.953846153846152,
-0.938461538461537,-0.923076923076922,-0.907692307692306,-0.892307692307691,
-0.876923076923076,-0.86153846153846,-0.846153846153845,-0.83076923076923,
-0.815384615384614,-0.799999999999999,-0.784615384615384,-0.769230769230768,
-0.753846153846153,-0.738461538461538,-0.723076923076922,-0.707692307692307,
-0.692307692307692,-0.676923076923076,-0.661538461538461,-0.646153846153846,
-0.63076923076923,-0.615384615384615,-0.6,-0.584615384615384,-0.569230769230769,
-0.553846153846154,-0.538461538461538,-0.523076923076923,-0.507692307692308,
-0.492307692307692,-0.476923076923077,-0.461538461538462,-0.446153846153846,
-0.430769230769231,-0.415384615384615,-0.4,-0.384615384615385,-0.369230769230769,
-0.353846153846154,-0.338461538461538,-0.323076923076923,-0.307692307692308,
-0.292307692307692,-0.276923076923077,-0.261538461538462,-0.246153846153846,
-0.230769230769231,-0.215384615384615,-0.2,-0.184615384615385,-0.169230769230769,
-0.153846153846154,-0.138461538461538,-0.123076923076923,-0.107692307692308,
-0.0923076923076923,-0.0769230769230769,-0.0615384615384615,-0.0461538461538462,
-0.0307692307692308,-0.0153846153846154,0.),.UNSPECIFIED.)
CURVE()
GEOMETRIC_REPRESENTATION_ITEM()
RATIONAL_B_SPLINE_CURVE((1.,1.,1.,1.,1.,1.,1.,1.,1.,1.,1.,1.,1.,1.,1.,1.,
1.,1.,1.,1.,1.,1.,1.,1.,1.,1.,1.,1.,1.,1.,1.,1.,1.,1.,1.,1.,1.,1.,1.,1.,
1.,1.,1.,1.,1.,1.,1.,1.,1.,1.,1.,1.,1.,1.,1.,1.,1.,1.,1.,1.,1.,1.,1.,1.,
1.,1.,1.,1.,1.,1.))
REPRESENTATION_ITEM('')
);
#172=(
BOUNDED_CURVE()
B_SPLINE_CURVE(5,(#30089,#30090,#30091,#30092,#30093,#30094,#30095,#30096,
#30097,#30098,#30099,#30100,#30101,#30102,#30103,#30104,#30105,#30106,#30107,
#30108,#30109,#30110,#30111,#30112,#30113,#30114,#30115,#30116,#30117,#30118,
#30119,#30120,#30121,#30122,#30123,#30124,#30125,#30126,#30127,#30128,#30129,
#30130,#30131,#30132,#30133,#30134,#30135,#30136,#30137,#30138,#30139,#30140,
#30141,#30142,#30143,#30144,#30145,#30146,#30147,#30148,#30149,#30150,#30151,
#30152,#30153,#30154,#30155,#30156,#30157,#30158),.UNSPECIFIED.,.F.,.F.)
B_SPLINE_CURVE_WITH_KNOTS((6,1,1,1,1,1,1,1,1,1,1,1,1,1,1,1,1,1,1,1,1,1,
1,1,1,1,1,1,1,1,1,1,1,1,1,1,1,1,1,1,1,1,1,1,1,1,1,1,1,1,1,1,1,1,1,1,1,1,
1,1,1,1,1,1,1,6),(-1.,-0.984615384615383,-0.969230769230768,-0.953846153846152,
-0.938461538461537,-0.923076923076922,-0.907692307692306,-0.892307692307691,
-0.876923076923076,-0.86153846153846,-0.846153846153845,-0.83076923076923,
-0.815384615384614,-0.799999999999999,-0.784615384615384,-0.769230769230768,
-0.753846153846153,-0.738461538461538,-0.723076923076922,-0.707692307692307,
-0.692307692307692,-0.676923076923076,-0.661538461538461,-0.646153846153846,
-0.63076923076923,-0.615384615384615,-0.6,-0.584615384615384,-0.569230769230769,
-0.553846153846154,-0.538461538461538,-0.523076923076923,-0.507692307692308,
-0.492307692307692,-0.476923076923077,-0.461538461538462,-0.446153846153846,
-0.430769230769231,-0.415384615384615,-0.4,-0.384615384615385,-0.369230769230769,
-0.353846153846154,-0.338461538461538,-0.323076923076923,-0.307692307692308,
-0.292307692307692,-0.276923076923077,-0.261538461538462,-0.246153846153846,
-0.230769230769231,-0.215384615384615,-0.2,-0.184615384615385,-0.169230769230769,
-0.153846153846154,-0.138461538461538,-0.123076923076923,-0.107692307692308,
-0.0923076923076923,-0.0769230769230769,-0.0615384615384615,-0.0461538461538462,
-0.0307692307692308,-0.0153846153846154,0.),.UNSPECIFIED.)
CURVE()
GEOMETRIC_REPRESENTATION_ITEM()
RATIONAL_B_SPLINE_CURVE((1.,1.,1.,1.,1.,1.,1.,1.,1.,1.,1.,1.,1.,1.,1.,1.,
1.,1.,1.,1.,1.,1.,1.,1.,1.,1.,1.,1.,1.,1.,1.,1.,1.,1.,1.,1.,1.,1.,1.,1.,
1.,1.,1.,1.,1.,1.,1.,1.,1.,1.,1.,1.,1.,1.,1.,1.,1.,1.,1.,1.,1.,1.,1.,1.,
1.,1.,1.,1.,1.,1.))
REPRESENTATION_ITEM('')
);
#173=(
BOUNDED_CURVE()
B_SPLINE_CURVE(5,(#30305,#30306,#30307,#30308,#30309,#30310,#30311,#30312,
#30313,#30314,#30315,#30316,#30317,#30318,#30319,#30320,#30321,#30322,#30323,
#30324,#30325,#30326,#30327,#30328,#30329,#30330,#30331,#30332,#30333,#30334,
#30335,#30336,#30337,#30338,#30339,#30340,#30341,#30342,#30343,#30344,#30345,
#30346,#30347,#30348,#30349,#30350,#30351,#30352,#30353,#30354,#30355,#30356,
#30357,#30358,#30359,#30360,#30361,#30362,#30363,#30364,#30365,#30366,#30367,
#30368,#30369,#30370,#30371,#30372,#30373,#30374),.UNSPECIFIED.,.F.,.F.)
B_SPLINE_CURVE_WITH_KNOTS((6,1,1,1,1,1,1,1,1,1,1,1,1,1,1,1,1,1,1,1,1,1,
1,1,1,1,1,1,1,1,1,1,1,1,1,1,1,1,1,1,1,1,1,1,1,1,1,1,1,1,1,1,1,1,1,1,1,1,
1,1,1,1,1,1,1,6),(-1.,-0.984615384615383,-0.969230769230768,-0.953846153846152,
-0.938461538461537,-0.923076923076922,-0.907692307692306,-0.892307692307691,
-0.876923076923076,-0.86153846153846,-0.846153846153845,-0.83076923076923,
-0.815384615384614,-0.799999999999999,-0.784615384615384,-0.769230769230768,
-0.753846153846153,-0.738461538461538,-0.723076923076922,-0.707692307692307,
-0.692307692307692,-0.676923076923076,-0.661538461538461,-0.646153846153846,
-0.63076923076923,-0.615384615384615,-0.6,-0.584615384615384,-0.569230769230769,
-0.553846153846154,-0.538461538461538,-0.523076923076923,-0.507692307692308,
-0.492307692307692,-0.476923076923077,-0.461538461538462,-0.446153846153846,
-0.430769230769231,-0.415384615384615,-0.4,-0.384615384615385,-0.369230769230769,
-0.353846153846154,-0.338461538461538,-0.323076923076923,-0.307692307692308,
-0.292307692307692,-0.276923076923077,-0.261538461538462,-0.246153846153846,
-0.230769230769231,-0.215384615384615,-0.2,-0.184615384615385,-0.169230769230769,
-0.153846153846154,-0.138461538461538,-0.123076923076923,-0.107692307692308,
-0.0923076923076923,-0.0769230769230769,-0.0615384615384615,-0.0461538461538462,
-0.0307692307692308,-0.0153846153846154,0.),.UNSPECIFIED.)
CURVE()
GEOMETRIC_REPRESENTATION_ITEM()
RATIONAL_B_SPLINE_CURVE((1.,1.,1.,1.,1.,1.,1.,1.,1.,1.,1.,1.,1.,1.,1.,1.,
1.,1.,1.,1.,1.,1.,1.,1.,1.,1.,1.,1.,1.,1.,1.,1.,1.,1.,1.,1.,1.,1.,1.,1.,
1.,1.,1.,1.,1.,1.,1.,1.,1.,1.,1.,1.,1.,1.,1.,1.,1.,1.,1.,1.,1.,1.,1.,1.,
1.,1.,1.,1.,1.,1.))
REPRESENTATION_ITEM('')
);
#174=(
BOUNDED_CURVE()
B_SPLINE_CURVE(5,(#30521,#30522,#30523,#30524,#30525,#30526,#30527,#30528,
#30529,#30530,#30531,#30532,#30533,#30534,#30535,#30536,#30537,#30538,#30539,
#30540,#30541,#30542,#30543,#30544,#30545,#30546,#30547,#30548,#30549,#30550,
#30551,#30552,#30553,#30554,#30555,#30556,#30557,#30558,#30559,#30560,#30561,
#30562,#30563,#30564,#30565,#30566,#30567,#30568,#30569,#30570,#30571,#30572,
#30573,#30574,#30575,#30576,#30577,#30578,#30579,#30580,#30581,#30582,#30583,
#30584,#30585,#30586,#30587,#30588,#30589,#30590),.UNSPECIFIED.,.F.,.F.)
B_SPLINE_CURVE_WITH_KNOTS((6,1,1,1,1,1,1,1,1,1,1,1,1,1,1,1,1,1,1,1,1,1,
1,1,1,1,1,1,1,1,1,1,1,1,1,1,1,1,1,1,1,1,1,1,1,1,1,1,1,1,1,1,1,1,1,1,1,1,
1,1,1,1,1,1,1,6),(-1.,-0.984615384615383,-0.969230769230768,-0.953846153846152,
-0.938461538461537,-0.923076923076922,-0.907692307692306,-0.892307692307691,
-0.876923076923076,-0.86153846153846,-0.846153846153845,-0.83076923076923,
-0.815384615384614,-0.799999999999999,-0.784615384615384,-0.769230769230768,
-0.753846153846153,-0.738461538461538,-0.723076923076922,-0.707692307692307,
-0.692307692307692,-0.676923076923076,-0.661538461538461,-0.646153846153846,
-0.63076923076923,-0.615384615384615,-0.6,-0.584615384615384,-0.569230769230769,
-0.553846153846154,-0.538461538461538,-0.523076923076923,-0.507692307692308,
-0.492307692307692,-0.476923076923077,-0.461538461538462,-0.446153846153846,
-0.430769230769231,-0.415384615384615,-0.4,-0.384615384615385,-0.369230769230769,
-0.353846153846154,-0.338461538461538,-0.323076923076923,-0.307692307692308,
-0.292307692307692,-0.276923076923077,-0.261538461538462,-0.246153846153846,
-0.230769230769231,-0.215384615384615,-0.2,-0.184615384615385,-0.169230769230769,
-0.153846153846154,-0.138461538461538,-0.123076923076923,-0.107692307692308,
-0.0923076923076923,-0.0769230769230769,-0.0615384615384615,-0.0461538461538462,
-0.0307692307692308,-0.0153846153846154,0.),.UNSPECIFIED.)
CURVE()
GEOMETRIC_REPRESENTATION_ITEM()
RATIONAL_B_SPLINE_CURVE((1.,1.,1.,1.,1.,1.,1.,1.,1.,1.,1.,1.,1.,1.,1.,1.,
1.,1.,1.,1.,1.,1.,1.,1.,1.,1.,1.,1.,1.,1.,1.,1.,1.,1.,1.,1.,1.,1.,1.,1.,
1.,1.,1.,1.,1.,1.,1.,1.,1.,1.,1.,1.,1.,1.,1.,1.,1.,1.,1.,1.,1.,1.,1.,1.,
1.,1.,1.,1.,1.,1.))
REPRESENTATION_ITEM('')
);
#175=(
BOUNDED_CURVE()
B_SPLINE_CURVE(5,(#30737,#30738,#30739,#30740,#30741,#30742,#30743,#30744,
#30745,#30746,#30747,#30748,#30749,#30750,#30751,#30752,#30753,#30754,#30755,
#30756,#30757,#30758,#30759,#30760,#30761,#30762,#30763,#30764,#30765,#30766,
#30767,#30768,#30769,#30770,#30771,#30772,#30773,#30774,#30775,#30776,#30777,
#30778,#30779,#30780,#30781,#30782,#30783,#30784,#30785,#30786,#30787,#30788,
#30789,#30790,#30791,#30792,#30793,#30794,#30795,#30796,#30797,#30798,#30799,
#30800,#30801,#30802,#30803,#30804,#30805,#30806),.UNSPECIFIED.,.F.,.F.)
B_SPLINE_CURVE_WITH_KNOTS((6,1,1,1,1,1,1,1,1,1,1,1,1,1,1,1,1,1,1,1,1,1,
1,1,1,1,1,1,1,1,1,1,1,1,1,1,1,1,1,1,1,1,1,1,1,1,1,1,1,1,1,1,1,1,1,1,1,1,
1,1,1,1,1,1,1,6),(-1.,-0.984615384615383,-0.969230769230768,-0.953846153846152,
-0.938461538461537,-0.923076923076922,-0.907692307692306,-0.892307692307691,
-0.876923076923076,-0.86153846153846,-0.846153846153845,-0.83076923076923,
-0.815384615384614,-0.799999999999999,-0.784615384615384,-0.769230769230768,
-0.753846153846153,-0.738461538461538,-0.723076923076922,-0.707692307692307,
-0.692307692307692,-0.676923076923076,-0.661538461538461,-0.646153846153846,
-0.63076923076923,-0.615384615384615,-0.6,-0.584615384615384,-0.569230769230769,
-0.553846153846154,-0.538461538461538,-0.523076923076923,-0.507692307692308,
-0.492307692307692,-0.476923076923077,-0.461538461538462,-0.446153846153846,
-0.430769230769231,-0.415384615384615,-0.4,-0.384615384615385,-0.369230769230769,
-0.353846153846154,-0.338461538461538,-0.323076923076923,-0.307692307692308,
-0.292307692307692,-0.276923076923077,-0.261538461538462,-0.246153846153846,
-0.230769230769231,-0.215384615384615,-0.2,-0.184615384615385,-0.169230769230769,
-0.153846153846154,-0.138461538461538,-0.123076923076923,-0.107692307692308,
-0.0923076923076923,-0.0769230769230769,-0.0615384615384615,-0.0461538461538462,
-0.0307692307692308,-0.0153846153846154,0.),.UNSPECIFIED.)
CURVE()
GEOMETRIC_REPRESENTATION_ITEM()
RATIONAL_B_SPLINE_CURVE((1.,1.,1.,1.,1.,1.,1.,1.,1.,1.,1.,1.,1.,1.,1.,1.,
1.,1.,1.,1.,1.,1.,1.,1.,1.,1.,1.,1.,1.,1.,1.,1.,1.,1.,1.,1.,1.,1.,1.,1.,
1.,1.,1.,1.,1.,1.,1.,1.,1.,1.,1.,1.,1.,1.,1.,1.,1.,1.,1.,1.,1.,1.,1.,1.,
1.,1.,1.,1.,1.,1.))
REPRESENTATION_ITEM('')
);
#176=(
BOUNDED_CURVE()
B_SPLINE_CURVE(5,(#30953,#30954,#30955,#30956,#30957,#30958,#30959,#30960,
#30961,#30962,#30963,#30964,#30965,#30966,#30967,#30968,#30969,#30970,#30971,
#30972,#30973,#30974,#30975,#30976,#30977,#30978,#30979,#30980,#30981,#30982,
#30983,#30984,#30985,#30986,#30987,#30988,#30989,#30990,#30991,#30992,#30993,
#30994,#30995,#30996,#30997,#30998,#30999,#31000,#31001,#31002,#31003,#31004,
#31005,#31006,#31007,#31008,#31009,#31010,#31011,#31012,#31013,#31014,#31015,
#31016,#31017,#31018,#31019,#31020,#31021,#31022),.UNSPECIFIED.,.F.,.F.)
B_SPLINE_CURVE_WITH_KNOTS((6,1,1,1,1,1,1,1,1,1,1,1,1,1,1,1,1,1,1,1,1,1,
1,1,1,1,1,1,1,1,1,1,1,1,1,1,1,1,1,1,1,1,1,1,1,1,1,1,1,1,1,1,1,1,1,1,1,1,
1,1,1,1,1,1,1,6),(-1.,-0.984615384615383,-0.969230769230768,-0.953846153846152,
-0.938461538461537,-0.923076923076922,-0.907692307692306,-0.892307692307691,
-0.876923076923076,-0.86153846153846,-0.846153846153845,-0.83076923076923,
-0.815384615384614,-0.799999999999999,-0.784615384615384,-0.769230769230768,
-0.753846153846153,-0.738461538461538,-0.723076923076922,-0.707692307692307,
-0.692307692307692,-0.676923076923076,-0.661538461538461,-0.646153846153846,
-0.63076923076923,-0.615384615384615,-0.6,-0.584615384615384,-0.569230769230769,
-0.553846153846154,-0.538461538461538,-0.523076923076923,-0.507692307692308,
-0.492307692307692,-0.476923076923077,-0.461538461538462,-0.446153846153846,
-0.430769230769231,-0.415384615384615,-0.4,-0.384615384615385,-0.369230769230769,
-0.353846153846154,-0.338461538461538,-0.323076923076923,-0.307692307692308,
-0.292307692307692,-0.276923076923077,-0.261538461538462,-0.246153846153846,
-0.230769230769231,-0.215384615384615,-0.2,-0.184615384615385,-0.169230769230769,
-0.153846153846154,-0.138461538461538,-0.123076923076923,-0.107692307692308,
-0.0923076923076923,-0.0769230769230769,-0.0615384615384615,-0.0461538461538462,
-0.0307692307692308,-0.0153846153846154,0.),.UNSPECIFIED.)
CURVE()
GEOMETRIC_REPRESENTATION_ITEM()
RATIONAL_B_SPLINE_CURVE((1.,1.,1.,1.,1.,1.,1.,1.,1.,1.,1.,1.,1.,1.,1.,1.,
1.,1.,1.,1.,1.,1.,1.,1.,1.,1.,1.,1.,1.,1.,1.,1.,1.,1.,1.,1.,1.,1.,1.,1.,
1.,1.,1.,1.,1.,1.,1.,1.,1.,1.,1.,1.,1.,1.,1.,1.,1.,1.,1.,1.,1.,1.,1.,1.,
1.,1.,1.,1.,1.,1.))
REPRESENTATION_ITEM('')
);
#177=(
BOUNDED_CURVE()
B_SPLINE_CURVE(5,(#31169,#31170,#31171,#31172,#31173,#31174,#31175,#31176,
#31177,#31178,#31179,#31180,#31181,#31182,#31183,#31184,#31185,#31186,#31187,
#31188,#31189,#31190,#31191,#31192,#31193,#31194,#31195,#31196,#31197,#31198,
#31199,#31200,#31201,#31202,#31203,#31204,#31205,#31206,#31207,#31208,#31209,
#31210,#31211,#31212,#31213,#31214,#31215,#31216,#31217,#31218,#31219,#31220,
#31221,#31222,#31223,#31224,#31225,#31226,#31227,#31228,#31229,#31230,#31231,
#31232,#31233,#31234,#31235,#31236,#31237,#31238),.UNSPECIFIED.,.F.,.F.)
B_SPLINE_CURVE_WITH_KNOTS((6,1,1,1,1,1,1,1,1,1,1,1,1,1,1,1,1,1,1,1,1,1,
1,1,1,1,1,1,1,1,1,1,1,1,1,1,1,1,1,1,1,1,1,1,1,1,1,1,1,1,1,1,1,1,1,1,1,1,
1,1,1,1,1,1,1,6),(-1.,-0.984615384615383,-0.969230769230768,-0.953846153846152,
-0.938461538461537,-0.923076923076922,-0.907692307692306,-0.892307692307691,
-0.876923076923076,-0.86153846153846,-0.846153846153845,-0.83076923076923,
-0.815384615384614,-0.799999999999999,-0.784615384615384,-0.769230769230768,
-0.753846153846153,-0.738461538461538,-0.723076923076922,-0.707692307692307,
-0.692307692307692,-0.676923076923076,-0.661538461538461,-0.646153846153846,
-0.63076923076923,-0.615384615384615,-0.6,-0.584615384615384,-0.569230769230769,
-0.553846153846154,-0.538461538461538,-0.523076923076923,-0.507692307692308,
-0.492307692307692,-0.476923076923077,-0.461538461538462,-0.446153846153846,
-0.430769230769231,-0.415384615384615,-0.4,-0.384615384615385,-0.369230769230769,
-0.353846153846154,-0.338461538461538,-0.323076923076923,-0.307692307692308,
-0.292307692307692,-0.276923076923077,-0.261538461538462,-0.246153846153846,
-0.230769230769231,-0.215384615384615,-0.2,-0.184615384615385,-0.169230769230769,
-0.153846153846154,-0.138461538461538,-0.123076923076923,-0.107692307692308,
-0.0923076923076923,-0.0769230769230769,-0.0615384615384615,-0.0461538461538462,
-0.0307692307692308,-0.0153846153846154,0.),.UNSPECIFIED.)
CURVE()
GEOMETRIC_REPRESENTATION_ITEM()
RATIONAL_B_SPLINE_CURVE((1.,1.,1.,1.,1.,1.,1.,1.,1.,1.,1.,1.,1.,1.,1.,1.,
1.,1.,1.,1.,1.,1.,1.,1.,1.,1.,1.,1.,1.,1.,1.,1.,1.,1.,1.,1.,1.,1.,1.,1.,
1.,1.,1.,1.,1.,1.,1.,1.,1.,1.,1.,1.,1.,1.,1.,1.,1.,1.,1.,1.,1.,1.,1.,1.,
1.,1.,1.,1.,1.,1.))
REPRESENTATION_ITEM('')
);
#178=(
BOUNDED_CURVE()
B_SPLINE_CURVE(5,(#31385,#31386,#31387,#31388,#31389,#31390,#31391,#31392,
#31393,#31394,#31395,#31396,#31397,#31398,#31399,#31400,#31401,#31402,#31403,
#31404,#31405,#31406,#31407,#31408,#31409,#31410,#31411,#31412,#31413,#31414,
#31415,#31416,#31417,#31418,#31419,#31420,#31421,#31422,#31423,#31424,#31425,
#31426,#31427,#31428,#31429,#31430,#31431,#31432,#31433,#31434,#31435,#31436,
#31437,#31438,#31439,#31440,#31441,#31442,#31443,#31444,#31445,#31446,#31447,
#31448,#31449,#31450,#31451,#31452,#31453,#31454),.UNSPECIFIED.,.F.,.F.)
B_SPLINE_CURVE_WITH_KNOTS((6,1,1,1,1,1,1,1,1,1,1,1,1,1,1,1,1,1,1,1,1,1,
1,1,1,1,1,1,1,1,1,1,1,1,1,1,1,1,1,1,1,1,1,1,1,1,1,1,1,1,1,1,1,1,1,1,1,1,
1,1,1,1,1,1,1,6),(-1.,-0.984615384615383,-0.969230769230768,-0.953846153846152,
-0.938461538461537,-0.923076923076922,-0.907692307692306,-0.892307692307691,
-0.876923076923076,-0.86153846153846,-0.846153846153845,-0.83076923076923,
-0.815384615384614,-0.799999999999999,-0.784615384615384,-0.769230769230768,
-0.753846153846153,-0.738461538461538,-0.723076923076922,-0.707692307692307,
-0.692307692307692,-0.676923076923076,-0.661538461538461,-0.646153846153846,
-0.63076923076923,-0.615384615384615,-0.6,-0.584615384615384,-0.569230769230769,
-0.553846153846154,-0.538461538461538,-0.523076923076923,-0.507692307692308,
-0.492307692307692,-0.476923076923077,-0.461538461538462,-0.446153846153846,
-0.430769230769231,-0.415384615384615,-0.4,-0.384615384615385,-0.369230769230769,
-0.353846153846154,-0.338461538461538,-0.323076923076923,-0.307692307692308,
-0.292307692307692,-0.276923076923077,-0.261538461538462,-0.246153846153846,
-0.230769230769231,-0.215384615384615,-0.2,-0.184615384615385,-0.169230769230769,
-0.153846153846154,-0.138461538461538,-0.123076923076923,-0.107692307692308,
-0.0923076923076923,-0.0769230769230769,-0.0615384615384615,-0.0461538461538462,
-0.0307692307692308,-0.0153846153846154,0.),.UNSPECIFIED.)
CURVE()
GEOMETRIC_REPRESENTATION_ITEM()
RATIONAL_B_SPLINE_CURVE((1.,1.,1.,1.,1.,1.,1.,1.,1.,1.,1.,1.,1.,1.,1.,1.,
1.,1.,1.,1.,1.,1.,1.,1.,1.,1.,1.,1.,1.,1.,1.,1.,1.,1.,1.,1.,1.,1.,1.,1.,
1.,1.,1.,1.,1.,1.,1.,1.,1.,1.,1.,1.,1.,1.,1.,1.,1.,1.,1.,1.,1.,1.,1.,1.,
1.,1.,1.,1.,1.,1.))
REPRESENTATION_ITEM('')
);
#179=(
BOUNDED_CURVE()
B_SPLINE_CURVE(5,(#31601,#31602,#31603,#31604,#31605,#31606,#31607,#31608,
#31609,#31610,#31611,#31612,#31613,#31614,#31615,#31616,#31617,#31618,#31619,
#31620,#31621,#31622,#31623,#31624,#31625,#31626,#31627,#31628,#31629,#31630,
#31631,#31632,#31633,#31634,#31635,#31636,#31637,#31638,#31639,#31640,#31641,
#31642,#31643,#31644,#31645,#31646,#31647,#31648,#31649,#31650,#31651,#31652,
#31653,#31654,#31655,#31656,#31657,#31658,#31659,#31660,#31661,#31662,#31663,
#31664,#31665,#31666,#31667,#31668,#31669,#31670),.UNSPECIFIED.,.F.,.F.)
B_SPLINE_CURVE_WITH_KNOTS((6,1,1,1,1,1,1,1,1,1,1,1,1,1,1,1,1,1,1,1,1,1,
1,1,1,1,1,1,1,1,1,1,1,1,1,1,1,1,1,1,1,1,1,1,1,1,1,1,1,1,1,1,1,1,1,1,1,1,
1,1,1,1,1,1,1,6),(-1.,-0.984615384615383,-0.969230769230768,-0.953846153846152,
-0.938461538461537,-0.923076923076922,-0.907692307692306,-0.892307692307691,
-0.876923076923076,-0.86153846153846,-0.846153846153845,-0.83076923076923,
-0.815384615384614,-0.799999999999999,-0.784615384615384,-0.769230769230768,
-0.753846153846153,-0.738461538461538,-0.723076923076922,-0.707692307692307,
-0.692307692307692,-0.676923076923076,-0.661538461538461,-0.646153846153846,
-0.63076923076923,-0.615384615384615,-0.6,-0.584615384615384,-0.569230769230769,
-0.553846153846154,-0.538461538461538,-0.523076923076923,-0.507692307692308,
-0.492307692307692,-0.476923076923077,-0.461538461538462,-0.446153846153846,
-0.430769230769231,-0.415384615384615,-0.4,-0.384615384615385,-0.369230769230769,
-0.353846153846154,-0.338461538461538,-0.323076923076923,-0.307692307692308,
-0.292307692307692,-0.276923076923077,-0.261538461538462,-0.246153846153846,
-0.230769230769231,-0.215384615384615,-0.2,-0.184615384615385,-0.169230769230769,
-0.153846153846154,-0.138461538461538,-0.123076923076923,-0.107692307692308,
-0.0923076923076923,-0.0769230769230769,-0.0615384615384615,-0.0461538461538462,
-0.0307692307692308,-0.0153846153846154,0.),.UNSPECIFIED.)
CURVE()
GEOMETRIC_REPRESENTATION_ITEM()
RATIONAL_B_SPLINE_CURVE((1.,1.,1.,1.,1.,1.,1.,1.,1.,1.,1.,1.,1.,1.,1.,1.,
1.,1.,1.,1.,1.,1.,1.,1.,1.,1.,1.,1.,1.,1.,1.,1.,1.,1.,1.,1.,1.,1.,1.,1.,
1.,1.,1.,1.,1.,1.,1.,1.,1.,1.,1.,1.,1.,1.,1.,1.,1.,1.,1.,1.,1.,1.,1.,1.,
1.,1.,1.,1.,1.,1.))
REPRESENTATION_ITEM('')
);
#180=(
BOUNDED_CURVE()
B_SPLINE_CURVE(5,(#31817,#31818,#31819,#31820,#31821,#31822,#31823,#31824,
#31825,#31826,#31827,#31828,#31829,#31830,#31831,#31832,#31833,#31834,#31835,
#31836,#31837,#31838,#31839,#31840,#31841,#31842,#31843,#31844,#31845,#31846,
#31847,#31848,#31849,#31850,#31851,#31852,#31853,#31854,#31855,#31856,#31857,
#31858,#31859,#31860,#31861,#31862,#31863,#31864,#31865,#31866,#31867,#31868,
#31869,#31870,#31871,#31872,#31873,#31874,#31875,#31876,#31877,#31878,#31879,
#31880,#31881,#31882,#31883,#31884,#31885,#31886),.UNSPECIFIED.,.F.,.F.)
B_SPLINE_CURVE_WITH_KNOTS((6,1,1,1,1,1,1,1,1,1,1,1,1,1,1,1,1,1,1,1,1,1,
1,1,1,1,1,1,1,1,1,1,1,1,1,1,1,1,1,1,1,1,1,1,1,1,1,1,1,1,1,1,1,1,1,1,1,1,
1,1,1,1,1,1,1,6),(-1.,-0.984615384615383,-0.969230769230768,-0.953846153846152,
-0.938461538461537,-0.923076923076922,-0.907692307692306,-0.892307692307691,
-0.876923076923076,-0.86153846153846,-0.846153846153845,-0.83076923076923,
-0.815384615384614,-0.799999999999999,-0.784615384615384,-0.769230769230768,
-0.753846153846153,-0.738461538461538,-0.723076923076922,-0.707692307692307,
-0.692307692307692,-0.676923076923076,-0.661538461538461,-0.646153846153846,
-0.63076923076923,-0.615384615384615,-0.6,-0.584615384615384,-0.569230769230769,
-0.553846153846154,-0.538461538461538,-0.523076923076923,-0.507692307692308,
-0.492307692307692,-0.476923076923077,-0.461538461538462,-0.446153846153846,
-0.430769230769231,-0.415384615384615,-0.4,-0.384615384615385,-0.369230769230769,
-0.353846153846154,-0.338461538461538,-0.323076923076923,-0.307692307692308,
-0.292307692307692,-0.276923076923077,-0.261538461538462,-0.246153846153846,
-0.230769230769231,-0.215384615384615,-0.2,-0.184615384615385,-0.169230769230769,
-0.153846153846154,-0.138461538461538,-0.123076923076923,-0.107692307692308,
-0.0923076923076923,-0.0769230769230769,-0.0615384615384615,-0.0461538461538462,
-0.0307692307692308,-0.0153846153846154,0.),.UNSPECIFIED.)
CURVE()
GEOMETRIC_REPRESENTATION_ITEM()
RATIONAL_B_SPLINE_CURVE((1.,1.,1.,1.,1.,1.,1.,1.,1.,1.,1.,1.,1.,1.,1.,1.,
1.,1.,1.,1.,1.,1.,1.,1.,1.,1.,1.,1.,1.,1.,1.,1.,1.,1.,1.,1.,1.,1.,1.,1.,
1.,1.,1.,1.,1.,1.,1.,1.,1.,1.,1.,1.,1.,1.,1.,1.,1.,1.,1.,1.,1.,1.,1.,1.,
1.,1.,1.,1.,1.,1.))
REPRESENTATION_ITEM('')
);
#181=(
BOUNDED_CURVE()
B_SPLINE_CURVE(5,(#32033,#32034,#32035,#32036,#32037,#32038,#32039,#32040,
#32041,#32042,#32043,#32044,#32045,#32046,#32047,#32048,#32049,#32050,#32051,
#32052,#32053,#32054,#32055,#32056,#32057,#32058,#32059,#32060,#32061,#32062,
#32063,#32064,#32065,#32066,#32067,#32068,#32069,#32070,#32071,#32072,#32073,
#32074,#32075,#32076,#32077,#32078,#32079,#32080,#32081,#32082,#32083,#32084,
#32085,#32086,#32087,#32088,#32089,#32090,#32091,#32092,#32093,#32094,#32095,
#32096,#32097,#32098,#32099,#32100,#32101,#32102),.UNSPECIFIED.,.F.,.F.)
B_SPLINE_CURVE_WITH_KNOTS((6,1,1,1,1,1,1,1,1,1,1,1,1,1,1,1,1,1,1,1,1,1,
1,1,1,1,1,1,1,1,1,1,1,1,1,1,1,1,1,1,1,1,1,1,1,1,1,1,1,1,1,1,1,1,1,1,1,1,
1,1,1,1,1,1,1,6),(-1.,-0.984615384615383,-0.969230769230768,-0.953846153846152,
-0.938461538461537,-0.923076923076922,-0.907692307692306,-0.892307692307691,
-0.876923076923076,-0.86153846153846,-0.846153846153845,-0.83076923076923,
-0.815384615384614,-0.799999999999999,-0.784615384615384,-0.769230769230768,
-0.753846153846153,-0.738461538461538,-0.723076923076922,-0.707692307692307,
-0.692307692307692,-0.676923076923076,-0.661538461538461,-0.646153846153846,
-0.63076923076923,-0.615384615384615,-0.6,-0.584615384615384,-0.569230769230769,
-0.553846153846154,-0.538461538461538,-0.523076923076923,-0.507692307692308,
-0.492307692307692,-0.476923076923077,-0.461538461538462,-0.446153846153846,
-0.430769230769231,-0.415384615384615,-0.4,-0.384615384615385,-0.369230769230769,
-0.353846153846154,-0.338461538461538,-0.323076923076923,-0.307692307692308,
-0.292307692307692,-0.276923076923077,-0.261538461538462,-0.246153846153846,
-0.230769230769231,-0.215384615384615,-0.2,-0.184615384615385,-0.169230769230769,
-0.153846153846154,-0.138461538461538,-0.123076923076923,-0.107692307692308,
-0.0923076923076923,-0.0769230769230769,-0.0615384615384615,-0.0461538461538462,
-0.0307692307692308,-0.0153846153846154,0.),.UNSPECIFIED.)
CURVE()
GEOMETRIC_REPRESENTATION_ITEM()
RATIONAL_B_SPLINE_CURVE((1.,1.,1.,1.,1.,1.,1.,1.,1.,1.,1.,1.,1.,1.,1.,1.,
1.,1.,1.,1.,1.,1.,1.,1.,1.,1.,1.,1.,1.,1.,1.,1.,1.,1.,1.,1.,1.,1.,1.,1.,
1.,1.,1.,1.,1.,1.,1.,1.,1.,1.,1.,1.,1.,1.,1.,1.,1.,1.,1.,1.,1.,1.,1.,1.,
1.,1.,1.,1.,1.,1.))
REPRESENTATION_ITEM('')
);
#182=(
BOUNDED_CURVE()
B_SPLINE_CURVE(5,(#32249,#32250,#32251,#32252,#32253,#32254,#32255,#32256,
#32257,#32258,#32259,#32260,#32261,#32262,#32263,#32264,#32265,#32266,#32267,
#32268,#32269,#32270,#32271,#32272,#32273,#32274,#32275,#32276,#32277,#32278,
#32279,#32280,#32281,#32282,#32283,#32284,#32285,#32286,#32287,#32288,#32289,
#32290,#32291,#32292,#32293,#32294,#32295,#32296,#32297,#32298,#32299,#32300,
#32301,#32302,#32303,#32304,#32305,#32306,#32307,#32308,#32309,#32310,#32311,
#32312,#32313,#32314,#32315,#32316,#32317,#32318),.UNSPECIFIED.,.F.,.F.)
B_SPLINE_CURVE_WITH_KNOTS((6,1,1,1,1,1,1,1,1,1,1,1,1,1,1,1,1,1,1,1,1,1,
1,1,1,1,1,1,1,1,1,1,1,1,1,1,1,1,1,1,1,1,1,1,1,1,1,1,1,1,1,1,1,1,1,1,1,1,
1,1,1,1,1,1,1,6),(-1.,-0.984615384615383,-0.969230769230768,-0.953846153846152,
-0.938461538461537,-0.923076923076922,-0.907692307692306,-0.892307692307691,
-0.876923076923076,-0.86153846153846,-0.846153846153845,-0.83076923076923,
-0.815384615384614,-0.799999999999999,-0.784615384615384,-0.769230769230768,
-0.753846153846153,-0.738461538461538,-0.723076923076922,-0.707692307692307,
-0.692307692307692,-0.676923076923076,-0.661538461538461,-0.646153846153846,
-0.63076923076923,-0.615384615384615,-0.6,-0.584615384615384,-0.569230769230769,
-0.553846153846154,-0.538461538461538,-0.523076923076923,-0.507692307692308,
-0.492307692307692,-0.476923076923077,-0.461538461538462,-0.446153846153846,
-0.430769230769231,-0.415384615384615,-0.4,-0.384615384615385,-0.369230769230769,
-0.353846153846154,-0.338461538461538,-0.323076923076923,-0.307692307692308,
-0.292307692307692,-0.276923076923077,-0.261538461538462,-0.246153846153846,
-0.230769230769231,-0.215384615384615,-0.2,-0.184615384615385,-0.169230769230769,
-0.153846153846154,-0.138461538461538,-0.123076923076923,-0.107692307692308,
-0.0923076923076923,-0.0769230769230769,-0.0615384615384615,-0.0461538461538462,
-0.0307692307692308,-0.0153846153846154,0.),.UNSPECIFIED.)
CURVE()
GEOMETRIC_REPRESENTATION_ITEM()
RATIONAL_B_SPLINE_CURVE((1.,1.,1.,1.,1.,1.,1.,1.,1.,1.,1.,1.,1.,1.,1.,1.,
1.,1.,1.,1.,1.,1.,1.,1.,1.,1.,1.,1.,1.,1.,1.,1.,1.,1.,1.,1.,1.,1.,1.,1.,
1.,1.,1.,1.,1.,1.,1.,1.,1.,1.,1.,1.,1.,1.,1.,1.,1.,1.,1.,1.,1.,1.,1.,1.,
1.,1.,1.,1.,1.,1.))
REPRESENTATION_ITEM('')
);
#183=(
BOUNDED_CURVE()
B_SPLINE_CURVE(5,(#32465,#32466,#32467,#32468,#32469,#32470,#32471,#32472,
#32473,#32474,#32475,#32476,#32477,#32478,#32479,#32480,#32481,#32482,#32483,
#32484,#32485,#32486,#32487,#32488,#32489,#32490,#32491,#32492,#32493,#32494,
#32495,#32496,#32497,#32498,#32499,#32500,#32501,#32502,#32503,#32504,#32505,
#32506,#32507,#32508,#32509,#32510,#32511,#32512,#32513,#32514,#32515,#32516,
#32517,#32518,#32519,#32520,#32521,#32522,#32523,#32524,#32525,#32526,#32527,
#32528,#32529,#32530,#32531,#32532,#32533,#32534),.UNSPECIFIED.,.F.,.F.)
B_SPLINE_CURVE_WITH_KNOTS((6,1,1,1,1,1,1,1,1,1,1,1,1,1,1,1,1,1,1,1,1,1,
1,1,1,1,1,1,1,1,1,1,1,1,1,1,1,1,1,1,1,1,1,1,1,1,1,1,1,1,1,1,1,1,1,1,1,1,
1,1,1,1,1,1,1,6),(-1.,-0.984615384615383,-0.969230769230768,-0.953846153846152,
-0.938461538461537,-0.923076923076922,-0.907692307692306,-0.892307692307691,
-0.876923076923076,-0.86153846153846,-0.846153846153845,-0.83076923076923,
-0.815384615384614,-0.799999999999999,-0.784615384615384,-0.769230769230768,
-0.753846153846153,-0.738461538461538,-0.723076923076922,-0.707692307692307,
-0.692307692307692,-0.676923076923076,-0.661538461538461,-0.646153846153846,
-0.63076923076923,-0.615384615384615,-0.6,-0.584615384615384,-0.569230769230769,
-0.553846153846154,-0.538461538461538,-0.523076923076923,-0.507692307692308,
-0.492307692307692,-0.476923076923077,-0.461538461538462,-0.446153846153846,
-0.430769230769231,-0.415384615384615,-0.4,-0.384615384615385,-0.369230769230769,
-0.353846153846154,-0.338461538461538,-0.323076923076923,-0.307692307692308,
-0.292307692307692,-0.276923076923077,-0.261538461538462,-0.246153846153846,
-0.230769230769231,-0.215384615384615,-0.2,-0.184615384615385,-0.169230769230769,
-0.153846153846154,-0.138461538461538,-0.123076923076923,-0.107692307692308,
-0.0923076923076923,-0.0769230769230769,-0.0615384615384615,-0.0461538461538462,
-0.0307692307692308,-0.0153846153846154,0.),.UNSPECIFIED.)
CURVE()
GEOMETRIC_REPRESENTATION_ITEM()
RATIONAL_B_SPLINE_CURVE((1.,1.,1.,1.,1.,1.,1.,1.,1.,1.,1.,1.,1.,1.,1.,1.,
1.,1.,1.,1.,1.,1.,1.,1.,1.,1.,1.,1.,1.,1.,1.,1.,1.,1.,1.,1.,1.,1.,1.,1.,
1.,1.,1.,1.,1.,1.,1.,1.,1.,1.,1.,1.,1.,1.,1.,1.,1.,1.,1.,1.,1.,1.,1.,1.,
1.,1.,1.,1.,1.,1.))
REPRESENTATION_ITEM('')
);
#184=(
BOUNDED_CURVE()
B_SPLINE_CURVE(5,(#32681,#32682,#32683,#32684,#32685,#32686,#32687,#32688,
#32689,#32690,#32691,#32692,#32693,#32694,#32695,#32696,#32697,#32698,#32699,
#32700,#32701,#32702,#32703,#32704,#32705,#32706,#32707,#32708,#32709,#32710,
#32711,#32712,#32713,#32714,#32715,#32716,#32717,#32718,#32719,#32720,#32721,
#32722,#32723,#32724,#32725,#32726,#32727,#32728,#32729,#32730,#32731,#32732,
#32733,#32734,#32735,#32736,#32737,#32738,#32739,#32740,#32741,#32742,#32743,
#32744,#32745,#32746,#32747,#32748,#32749,#32750),.UNSPECIFIED.,.F.,.F.)
B_SPLINE_CURVE_WITH_KNOTS((6,1,1,1,1,1,1,1,1,1,1,1,1,1,1,1,1,1,1,1,1,1,
1,1,1,1,1,1,1,1,1,1,1,1,1,1,1,1,1,1,1,1,1,1,1,1,1,1,1,1,1,1,1,1,1,1,1,1,
1,1,1,1,1,1,1,6),(-1.,-0.984615384615383,-0.969230769230768,-0.953846153846152,
-0.938461538461537,-0.923076923076922,-0.907692307692306,-0.892307692307691,
-0.876923076923076,-0.86153846153846,-0.846153846153845,-0.83076923076923,
-0.815384615384614,-0.799999999999999,-0.784615384615384,-0.769230769230768,
-0.753846153846153,-0.738461538461538,-0.723076923076922,-0.707692307692307,
-0.692307692307692,-0.676923076923076,-0.661538461538461,-0.646153846153846,
-0.63076923076923,-0.615384615384615,-0.6,-0.584615384615384,-0.569230769230769,
-0.553846153846154,-0.538461538461538,-0.523076923076923,-0.507692307692308,
-0.492307692307692,-0.476923076923077,-0.461538461538462,-0.446153846153846,
-0.430769230769231,-0.415384615384615,-0.4,-0.384615384615385,-0.369230769230769,
-0.353846153846154,-0.338461538461538,-0.323076923076923,-0.307692307692308,
-0.292307692307692,-0.276923076923077,-0.261538461538462,-0.246153846153846,
-0.230769230769231,-0.215384615384615,-0.2,-0.184615384615385,-0.169230769230769,
-0.153846153846154,-0.138461538461538,-0.123076923076923,-0.107692307692308,
-0.0923076923076923,-0.0769230769230769,-0.0615384615384615,-0.0461538461538462,
-0.0307692307692308,-0.0153846153846154,0.),.UNSPECIFIED.)
CURVE()
GEOMETRIC_REPRESENTATION_ITEM()
RATIONAL_B_SPLINE_CURVE((1.,1.,1.,1.,1.,1.,1.,1.,1.,1.,1.,1.,1.,1.,1.,1.,
1.,1.,1.,1.,1.,1.,1.,1.,1.,1.,1.,1.,1.,1.,1.,1.,1.,1.,1.,1.,1.,1.,1.,1.,
1.,1.,1.,1.,1.,1.,1.,1.,1.,1.,1.,1.,1.,1.,1.,1.,1.,1.,1.,1.,1.,1.,1.,1.,
1.,1.,1.,1.,1.,1.))
REPRESENTATION_ITEM('')
);
#185=(
BOUNDED_CURVE()
B_SPLINE_CURVE(5,(#32897,#32898,#32899,#32900,#32901,#32902,#32903,#32904,
#32905,#32906,#32907,#32908,#32909,#32910,#32911,#32912,#32913,#32914,#32915,
#32916,#32917,#32918,#32919,#32920,#32921,#32922,#32923,#32924,#32925,#32926,
#32927,#32928,#32929,#32930,#32931,#32932,#32933,#32934,#32935,#32936,#32937,
#32938,#32939,#32940,#32941,#32942,#32943,#32944,#32945,#32946,#32947,#32948,
#32949,#32950,#32951,#32952,#32953,#32954,#32955,#32956,#32957,#32958,#32959,
#32960,#32961,#32962,#32963,#32964,#32965,#32966),.UNSPECIFIED.,.F.,.F.)
B_SPLINE_CURVE_WITH_KNOTS((6,1,1,1,1,1,1,1,1,1,1,1,1,1,1,1,1,1,1,1,1,1,
1,1,1,1,1,1,1,1,1,1,1,1,1,1,1,1,1,1,1,1,1,1,1,1,1,1,1,1,1,1,1,1,1,1,1,1,
1,1,1,1,1,1,1,6),(-1.,-0.984615384615383,-0.969230769230768,-0.953846153846152,
-0.938461538461537,-0.923076923076922,-0.907692307692306,-0.892307692307691,
-0.876923076923076,-0.86153846153846,-0.846153846153845,-0.83076923076923,
-0.815384615384614,-0.799999999999999,-0.784615384615384,-0.769230769230768,
-0.753846153846153,-0.738461538461538,-0.723076923076922,-0.707692307692307,
-0.692307692307692,-0.676923076923076,-0.661538461538461,-0.646153846153846,
-0.63076923076923,-0.615384615384615,-0.6,-0.584615384615384,-0.569230769230769,
-0.553846153846154,-0.538461538461538,-0.523076923076923,-0.507692307692308,
-0.492307692307692,-0.476923076923077,-0.461538461538462,-0.446153846153846,
-0.430769230769231,-0.415384615384615,-0.4,-0.384615384615385,-0.369230769230769,
-0.353846153846154,-0.338461538461538,-0.323076923076923,-0.307692307692308,
-0.292307692307692,-0.276923076923077,-0.261538461538462,-0.246153846153846,
-0.230769230769231,-0.215384615384615,-0.2,-0.184615384615385,-0.169230769230769,
-0.153846153846154,-0.138461538461538,-0.123076923076923,-0.107692307692308,
-0.0923076923076923,-0.0769230769230769,-0.0615384615384615,-0.0461538461538462,
-0.0307692307692308,-0.0153846153846154,0.),.UNSPECIFIED.)
CURVE()
GEOMETRIC_REPRESENTATION_ITEM()
RATIONAL_B_SPLINE_CURVE((1.,1.,1.,1.,1.,1.,1.,1.,1.,1.,1.,1.,1.,1.,1.,1.,
1.,1.,1.,1.,1.,1.,1.,1.,1.,1.,1.,1.,1.,1.,1.,1.,1.,1.,1.,1.,1.,1.,1.,1.,
1.,1.,1.,1.,1.,1.,1.,1.,1.,1.,1.,1.,1.,1.,1.,1.,1.,1.,1.,1.,1.,1.,1.,1.,
1.,1.,1.,1.,1.,1.))
REPRESENTATION_ITEM('')
);
#186=(
BOUNDED_CURVE()
B_SPLINE_CURVE(5,(#33113,#33114,#33115,#33116,#33117,#33118,#33119,#33120,
#33121,#33122,#33123,#33124,#33125,#33126,#33127,#33128,#33129,#33130,#33131,
#33132,#33133,#33134,#33135,#33136,#33137,#33138,#33139,#33140,#33141,#33142,
#33143,#33144,#33145,#33146,#33147,#33148,#33149,#33150,#33151,#33152,#33153,
#33154,#33155,#33156,#33157,#33158,#33159,#33160,#33161,#33162,#33163,#33164,
#33165,#33166,#33167,#33168,#33169,#33170,#33171,#33172,#33173,#33174,#33175,
#33176,#33177,#33178,#33179,#33180,#33181,#33182),.UNSPECIFIED.,.F.,.F.)
B_SPLINE_CURVE_WITH_KNOTS((6,1,1,1,1,1,1,1,1,1,1,1,1,1,1,1,1,1,1,1,1,1,
1,1,1,1,1,1,1,1,1,1,1,1,1,1,1,1,1,1,1,1,1,1,1,1,1,1,1,1,1,1,1,1,1,1,1,1,
1,1,1,1,1,1,1,6),(-1.,-0.984615384615383,-0.969230769230768,-0.953846153846152,
-0.938461538461537,-0.923076923076922,-0.907692307692306,-0.892307692307691,
-0.876923076923076,-0.86153846153846,-0.846153846153845,-0.83076923076923,
-0.815384615384614,-0.799999999999999,-0.784615384615384,-0.769230769230768,
-0.753846153846153,-0.738461538461538,-0.723076923076922,-0.707692307692307,
-0.692307692307692,-0.676923076923076,-0.661538461538461,-0.646153846153846,
-0.63076923076923,-0.615384615384615,-0.6,-0.584615384615384,-0.569230769230769,
-0.553846153846154,-0.538461538461538,-0.523076923076923,-0.507692307692308,
-0.492307692307692,-0.476923076923077,-0.461538461538462,-0.446153846153846,
-0.430769230769231,-0.415384615384615,-0.4,-0.384615384615385,-0.369230769230769,
-0.353846153846154,-0.338461538461538,-0.323076923076923,-0.307692307692308,
-0.292307692307692,-0.276923076923077,-0.261538461538462,-0.246153846153846,
-0.230769230769231,-0.215384615384615,-0.2,-0.184615384615385,-0.169230769230769,
-0.153846153846154,-0.138461538461538,-0.123076923076923,-0.107692307692308,
-0.0923076923076923,-0.0769230769230769,-0.0615384615384615,-0.0461538461538462,
-0.0307692307692308,-0.0153846153846154,0.),.UNSPECIFIED.)
CURVE()
GEOMETRIC_REPRESENTATION_ITEM()
RATIONAL_B_SPLINE_CURVE((1.,1.,1.,1.,1.,1.,1.,1.,1.,1.,1.,1.,1.,1.,1.,1.,
1.,1.,1.,1.,1.,1.,1.,1.,1.,1.,1.,1.,1.,1.,1.,1.,1.,1.,1.,1.,1.,1.,1.,1.,
1.,1.,1.,1.,1.,1.,1.,1.,1.,1.,1.,1.,1.,1.,1.,1.,1.,1.,1.,1.,1.,1.,1.,1.,
1.,1.,1.,1.,1.,1.))
REPRESENTATION_ITEM('')
);
#187=(
BOUNDED_CURVE()
B_SPLINE_CURVE(5,(#33329,#33330,#33331,#33332,#33333,#33334,#33335,#33336,
#33337,#33338,#33339,#33340,#33341,#33342,#33343,#33344,#33345,#33346,#33347,
#33348,#33349,#33350,#33351,#33352,#33353,#33354,#33355,#33356,#33357,#33358,
#33359,#33360,#33361,#33362,#33363,#33364,#33365,#33366,#33367,#33368,#33369,
#33370,#33371,#33372,#33373,#33374,#33375,#33376,#33377,#33378,#33379,#33380,
#33381,#33382,#33383,#33384,#33385,#33386,#33387,#33388,#33389,#33390,#33391,
#33392,#33393,#33394,#33395,#33396,#33397,#33398),.UNSPECIFIED.,.F.,.F.)
B_SPLINE_CURVE_WITH_KNOTS((6,1,1,1,1,1,1,1,1,1,1,1,1,1,1,1,1,1,1,1,1,1,
1,1,1,1,1,1,1,1,1,1,1,1,1,1,1,1,1,1,1,1,1,1,1,1,1,1,1,1,1,1,1,1,1,1,1,1,
1,1,1,1,1,1,1,6),(-1.,-0.984615384615383,-0.969230769230768,-0.953846153846152,
-0.938461538461537,-0.923076923076922,-0.907692307692306,-0.892307692307691,
-0.876923076923076,-0.86153846153846,-0.846153846153845,-0.83076923076923,
-0.815384615384614,-0.799999999999999,-0.784615384615384,-0.769230769230768,
-0.753846153846153,-0.738461538461538,-0.723076923076922,-0.707692307692307,
-0.692307692307692,-0.676923076923076,-0.661538461538461,-0.646153846153846,
-0.63076923076923,-0.615384615384615,-0.6,-0.584615384615384,-0.569230769230769,
-0.553846153846154,-0.538461538461538,-0.523076923076923,-0.507692307692308,
-0.492307692307692,-0.476923076923077,-0.461538461538462,-0.446153846153846,
-0.430769230769231,-0.415384615384615,-0.4,-0.384615384615385,-0.369230769230769,
-0.353846153846154,-0.338461538461538,-0.323076923076923,-0.307692307692308,
-0.292307692307692,-0.276923076923077,-0.261538461538462,-0.246153846153846,
-0.230769230769231,-0.215384615384615,-0.2,-0.184615384615385,-0.169230769230769,
-0.153846153846154,-0.138461538461538,-0.123076923076923,-0.107692307692308,
-0.0923076923076923,-0.0769230769230769,-0.0615384615384615,-0.0461538461538462,
-0.0307692307692308,-0.0153846153846154,0.),.UNSPECIFIED.)
CURVE()
GEOMETRIC_REPRESENTATION_ITEM()
RATIONAL_B_SPLINE_CURVE((1.,1.,1.,1.,1.,1.,1.,1.,1.,1.,1.,1.,1.,1.,1.,1.,
1.,1.,1.,1.,1.,1.,1.,1.,1.,1.,1.,1.,1.,1.,1.,1.,1.,1.,1.,1.,1.,1.,1.,1.,
1.,1.,1.,1.,1.,1.,1.,1.,1.,1.,1.,1.,1.,1.,1.,1.,1.,1.,1.,1.,1.,1.,1.,1.,
1.,1.,1.,1.,1.,1.))
REPRESENTATION_ITEM('')
);
#188=(
BOUNDED_CURVE()
B_SPLINE_CURVE(5,(#33545,#33546,#33547,#33548,#33549,#33550,#33551,#33552,
#33553,#33554,#33555,#33556,#33557,#33558,#33559,#33560,#33561,#33562,#33563,
#33564,#33565,#33566,#33567,#33568,#33569,#33570,#33571,#33572,#33573,#33574,
#33575,#33576,#33577,#33578,#33579,#33580,#33581,#33582,#33583,#33584,#33585,
#33586,#33587,#33588,#33589,#33590,#33591,#33592,#33593,#33594,#33595,#33596,
#33597,#33598,#33599,#33600,#33601,#33602,#33603,#33604,#33605,#33606,#33607,
#33608,#33609,#33610,#33611,#33612,#33613,#33614),.UNSPECIFIED.,.F.,.F.)
B_SPLINE_CURVE_WITH_KNOTS((6,1,1,1,1,1,1,1,1,1,1,1,1,1,1,1,1,1,1,1,1,1,
1,1,1,1,1,1,1,1,1,1,1,1,1,1,1,1,1,1,1,1,1,1,1,1,1,1,1,1,1,1,1,1,1,1,1,1,
1,1,1,1,1,1,1,6),(-1.,-0.984615384615383,-0.969230769230768,-0.953846153846152,
-0.938461538461537,-0.923076923076922,-0.907692307692306,-0.892307692307691,
-0.876923076923076,-0.86153846153846,-0.846153846153845,-0.83076923076923,
-0.815384615384614,-0.799999999999999,-0.784615384615384,-0.769230769230768,
-0.753846153846153,-0.738461538461538,-0.723076923076922,-0.707692307692307,
-0.692307692307692,-0.676923076923076,-0.661538461538461,-0.646153846153846,
-0.63076923076923,-0.615384615384615,-0.6,-0.584615384615384,-0.569230769230769,
-0.553846153846154,-0.538461538461538,-0.523076923076923,-0.507692307692308,
-0.492307692307692,-0.476923076923077,-0.461538461538462,-0.446153846153846,
-0.430769230769231,-0.415384615384615,-0.4,-0.384615384615385,-0.369230769230769,
-0.353846153846154,-0.338461538461538,-0.323076923076923,-0.307692307692308,
-0.292307692307692,-0.276923076923077,-0.261538461538462,-0.246153846153846,
-0.230769230769231,-0.215384615384615,-0.2,-0.184615384615385,-0.169230769230769,
-0.153846153846154,-0.138461538461538,-0.123076923076923,-0.107692307692308,
-0.0923076923076923,-0.0769230769230769,-0.0615384615384615,-0.0461538461538462,
-0.0307692307692308,-0.0153846153846154,0.),.UNSPECIFIED.)
CURVE()
GEOMETRIC_REPRESENTATION_ITEM()
RATIONAL_B_SPLINE_CURVE((1.,1.,1.,1.,1.,1.,1.,1.,1.,1.,1.,1.,1.,1.,1.,1.,
1.,1.,1.,1.,1.,1.,1.,1.,1.,1.,1.,1.,1.,1.,1.,1.,1.,1.,1.,1.,1.,1.,1.,1.,
1.,1.,1.,1.,1.,1.,1.,1.,1.,1.,1.,1.,1.,1.,1.,1.,1.,1.,1.,1.,1.,1.,1.,1.,
1.,1.,1.,1.,1.,1.))
REPRESENTATION_ITEM('')
);
#189=(
BOUNDED_CURVE()
B_SPLINE_CURVE(5,(#33761,#33762,#33763,#33764,#33765,#33766,#33767,#33768,
#33769,#33770,#33771,#33772,#33773,#33774,#33775,#33776,#33777,#33778,#33779,
#33780,#33781,#33782,#33783,#33784,#33785,#33786,#33787,#33788,#33789,#33790,
#33791,#33792,#33793,#33794,#33795,#33796,#33797,#33798,#33799,#33800,#33801,
#33802,#33803,#33804,#33805,#33806,#33807,#33808,#33809,#33810,#33811,#33812,
#33813,#33814,#33815,#33816,#33817,#33818,#33819,#33820,#33821,#33822,#33823,
#33824,#33825,#33826,#33827,#33828,#33829,#33830),.UNSPECIFIED.,.F.,.F.)
B_SPLINE_CURVE_WITH_KNOTS((6,1,1,1,1,1,1,1,1,1,1,1,1,1,1,1,1,1,1,1,1,1,
1,1,1,1,1,1,1,1,1,1,1,1,1,1,1,1,1,1,1,1,1,1,1,1,1,1,1,1,1,1,1,1,1,1,1,1,
1,1,1,1,1,1,1,6),(-1.,-0.984615384615383,-0.969230769230768,-0.953846153846152,
-0.938461538461537,-0.923076923076922,-0.907692307692306,-0.892307692307691,
-0.876923076923076,-0.86153846153846,-0.846153846153845,-0.83076923076923,
-0.815384615384614,-0.799999999999999,-0.784615384615384,-0.769230769230768,
-0.753846153846153,-0.738461538461538,-0.723076923076922,-0.707692307692307,
-0.692307692307692,-0.676923076923076,-0.661538461538461,-0.646153846153846,
-0.63076923076923,-0.615384615384615,-0.6,-0.584615384615384,-0.569230769230769,
-0.553846153846154,-0.538461538461538,-0.523076923076923,-0.507692307692308,
-0.492307692307692,-0.476923076923077,-0.461538461538462,-0.446153846153846,
-0.430769230769231,-0.415384615384615,-0.4,-0.384615384615385,-0.369230769230769,
-0.353846153846154,-0.338461538461538,-0.323076923076923,-0.307692307692308,
-0.292307692307692,-0.276923076923077,-0.261538461538462,-0.246153846153846,
-0.230769230769231,-0.215384615384615,-0.2,-0.184615384615385,-0.169230769230769,
-0.153846153846154,-0.138461538461538,-0.123076923076923,-0.107692307692308,
-0.0923076923076923,-0.0769230769230769,-0.0615384615384615,-0.0461538461538462,
-0.0307692307692308,-0.0153846153846154,0.),.UNSPECIFIED.)
CURVE()
GEOMETRIC_REPRESENTATION_ITEM()
RATIONAL_B_SPLINE_CURVE((1.,1.,1.,1.,1.,1.,1.,1.,1.,1.,1.,1.,1.,1.,1.,1.,
1.,1.,1.,1.,1.,1.,1.,1.,1.,1.,1.,1.,1.,1.,1.,1.,1.,1.,1.,1.,1.,1.,1.,1.,
1.,1.,1.,1.,1.,1.,1.,1.,1.,1.,1.,1.,1.,1.,1.,1.,1.,1.,1.,1.,1.,1.,1.,1.,
1.,1.,1.,1.,1.,1.))
REPRESENTATION_ITEM('')
);
#190=(
BOUNDED_CURVE()
B_SPLINE_CURVE(5,(#33977,#33978,#33979,#33980,#33981,#33982,#33983,#33984,
#33985,#33986,#33987,#33988,#33989,#33990,#33991,#33992,#33993,#33994,#33995,
#33996,#33997,#33998,#33999,#34000,#34001,#34002,#34003,#34004,#34005,#34006,
#34007,#34008,#34009,#34010,#34011,#34012,#34013,#34014,#34015,#34016,#34017,
#34018,#34019,#34020,#34021,#34022,#34023,#34024,#34025,#34026,#34027,#34028,
#34029,#34030,#34031,#34032,#34033,#34034,#34035,#34036,#34037,#34038,#34039,
#34040,#34041,#34042,#34043,#34044,#34045,#34046),.UNSPECIFIED.,.F.,.F.)
B_SPLINE_CURVE_WITH_KNOTS((6,1,1,1,1,1,1,1,1,1,1,1,1,1,1,1,1,1,1,1,1,1,
1,1,1,1,1,1,1,1,1,1,1,1,1,1,1,1,1,1,1,1,1,1,1,1,1,1,1,1,1,1,1,1,1,1,1,1,
1,1,1,1,1,1,1,6),(-1.,-0.984615384615383,-0.969230769230768,-0.953846153846152,
-0.938461538461537,-0.923076923076922,-0.907692307692306,-0.892307692307691,
-0.876923076923076,-0.86153846153846,-0.846153846153845,-0.83076923076923,
-0.815384615384614,-0.799999999999999,-0.784615384615384,-0.769230769230768,
-0.753846153846153,-0.738461538461538,-0.723076923076922,-0.707692307692307,
-0.692307692307692,-0.676923076923076,-0.661538461538461,-0.646153846153846,
-0.63076923076923,-0.615384615384615,-0.6,-0.584615384615384,-0.569230769230769,
-0.553846153846154,-0.538461538461538,-0.523076923076923,-0.507692307692308,
-0.492307692307692,-0.476923076923077,-0.461538461538462,-0.446153846153846,
-0.430769230769231,-0.415384615384615,-0.4,-0.384615384615385,-0.369230769230769,
-0.353846153846154,-0.338461538461538,-0.323076923076923,-0.307692307692308,
-0.292307692307692,-0.276923076923077,-0.261538461538462,-0.246153846153846,
-0.230769230769231,-0.215384615384615,-0.2,-0.184615384615385,-0.169230769230769,
-0.153846153846154,-0.138461538461538,-0.123076923076923,-0.107692307692308,
-0.0923076923076923,-0.0769230769230769,-0.0615384615384615,-0.0461538461538462,
-0.0307692307692308,-0.0153846153846154,0.),.UNSPECIFIED.)
CURVE()
GEOMETRIC_REPRESENTATION_ITEM()
RATIONAL_B_SPLINE_CURVE((1.,1.,1.,1.,1.,1.,1.,1.,1.,1.,1.,1.,1.,1.,1.,1.,
1.,1.,1.,1.,1.,1.,1.,1.,1.,1.,1.,1.,1.,1.,1.,1.,1.,1.,1.,1.,1.,1.,1.,1.,
1.,1.,1.,1.,1.,1.,1.,1.,1.,1.,1.,1.,1.,1.,1.,1.,1.,1.,1.,1.,1.,1.,1.,1.,
1.,1.,1.,1.,1.,1.))
REPRESENTATION_ITEM('')
);
#191=(
BOUNDED_CURVE()
B_SPLINE_CURVE(5,(#34193,#34194,#34195,#34196,#34197,#34198,#34199,#34200,
#34201,#34202,#34203,#34204,#34205,#34206,#34207,#34208,#34209,#34210,#34211,
#34212,#34213,#34214,#34215,#34216,#34217,#34218,#34219,#34220,#34221,#34222,
#34223,#34224,#34225,#34226,#34227,#34228,#34229,#34230,#34231,#34232,#34233,
#34234,#34235,#34236,#34237,#34238,#34239,#34240,#34241,#34242,#34243,#34244,
#34245,#34246,#34247,#34248,#34249,#34250,#34251,#34252,#34253,#34254,#34255,
#34256,#34257,#34258,#34259,#34260,#34261,#34262),.UNSPECIFIED.,.F.,.F.)
B_SPLINE_CURVE_WITH_KNOTS((6,1,1,1,1,1,1,1,1,1,1,1,1,1,1,1,1,1,1,1,1,1,
1,1,1,1,1,1,1,1,1,1,1,1,1,1,1,1,1,1,1,1,1,1,1,1,1,1,1,1,1,1,1,1,1,1,1,1,
1,1,1,1,1,1,1,6),(-1.,-0.984615384615383,-0.969230769230768,-0.953846153846152,
-0.938461538461537,-0.923076923076922,-0.907692307692306,-0.892307692307691,
-0.876923076923076,-0.86153846153846,-0.846153846153845,-0.83076923076923,
-0.815384615384614,-0.799999999999999,-0.784615384615384,-0.769230769230768,
-0.753846153846153,-0.738461538461538,-0.723076923076922,-0.707692307692307,
-0.692307692307692,-0.676923076923076,-0.661538461538461,-0.646153846153846,
-0.63076923076923,-0.615384615384615,-0.6,-0.584615384615384,-0.569230769230769,
-0.553846153846154,-0.538461538461538,-0.523076923076923,-0.507692307692308,
-0.492307692307692,-0.476923076923077,-0.461538461538462,-0.446153846153846,
-0.430769230769231,-0.415384615384615,-0.4,-0.384615384615385,-0.369230769230769,
-0.353846153846154,-0.338461538461538,-0.323076923076923,-0.307692307692308,
-0.292307692307692,-0.276923076923077,-0.261538461538462,-0.246153846153846,
-0.230769230769231,-0.215384615384615,-0.2,-0.184615384615385,-0.169230769230769,
-0.153846153846154,-0.138461538461538,-0.123076923076923,-0.107692307692308,
-0.0923076923076923,-0.0769230769230769,-0.0615384615384615,-0.0461538461538462,
-0.0307692307692308,-0.0153846153846154,0.),.UNSPECIFIED.)
CURVE()
GEOMETRIC_REPRESENTATION_ITEM()
RATIONAL_B_SPLINE_CURVE((1.,1.,1.,1.,1.,1.,1.,1.,1.,1.,1.,1.,1.,1.,1.,1.,
1.,1.,1.,1.,1.,1.,1.,1.,1.,1.,1.,1.,1.,1.,1.,1.,1.,1.,1.,1.,1.,1.,1.,1.,
1.,1.,1.,1.,1.,1.,1.,1.,1.,1.,1.,1.,1.,1.,1.,1.,1.,1.,1.,1.,1.,1.,1.,1.,
1.,1.,1.,1.,1.,1.))
REPRESENTATION_ITEM('')
);
#192=(
BOUNDED_CURVE()
B_SPLINE_CURVE(5,(#34409,#34410,#34411,#34412,#34413,#34414,#34415,#34416,
#34417,#34418,#34419,#34420,#34421,#34422,#34423,#34424,#34425,#34426,#34427,
#34428,#34429,#34430,#34431,#34432,#34433,#34434,#34435,#34436,#34437,#34438,
#34439,#34440,#34441,#34442,#34443,#34444,#34445,#34446,#34447,#34448,#34449,
#34450,#34451,#34452,#34453,#34454,#34455,#34456,#34457,#34458,#34459,#34460,
#34461,#34462,#34463,#34464,#34465,#34466,#34467,#34468,#34469,#34470,#34471,
#34472,#34473,#34474,#34475,#34476,#34477,#34478),.UNSPECIFIED.,.F.,.F.)
B_SPLINE_CURVE_WITH_KNOTS((6,1,1,1,1,1,1,1,1,1,1,1,1,1,1,1,1,1,1,1,1,1,
1,1,1,1,1,1,1,1,1,1,1,1,1,1,1,1,1,1,1,1,1,1,1,1,1,1,1,1,1,1,1,1,1,1,1,1,
1,1,1,1,1,1,1,6),(-1.,-0.984615384615383,-0.969230769230768,-0.953846153846152,
-0.938461538461537,-0.923076923076922,-0.907692307692306,-0.892307692307691,
-0.876923076923076,-0.86153846153846,-0.846153846153845,-0.83076923076923,
-0.815384615384614,-0.799999999999999,-0.784615384615384,-0.769230769230768,
-0.753846153846153,-0.738461538461538,-0.723076923076922,-0.707692307692307,
-0.692307692307692,-0.676923076923076,-0.661538461538461,-0.646153846153846,
-0.63076923076923,-0.615384615384615,-0.6,-0.584615384615384,-0.569230769230769,
-0.553846153846154,-0.538461538461538,-0.523076923076923,-0.507692307692308,
-0.492307692307692,-0.476923076923077,-0.461538461538462,-0.446153846153846,
-0.430769230769231,-0.415384615384615,-0.4,-0.384615384615385,-0.369230769230769,
-0.353846153846154,-0.338461538461538,-0.323076923076923,-0.307692307692308,
-0.292307692307692,-0.276923076923077,-0.261538461538462,-0.246153846153846,
-0.230769230769231,-0.215384615384615,-0.2,-0.184615384615385,-0.169230769230769,
-0.153846153846154,-0.138461538461538,-0.123076923076923,-0.107692307692308,
-0.0923076923076923,-0.0769230769230769,-0.0615384615384615,-0.0461538461538462,
-0.0307692307692308,-0.0153846153846154,0.),.UNSPECIFIED.)
CURVE()
GEOMETRIC_REPRESENTATION_ITEM()
RATIONAL_B_SPLINE_CURVE((1.,1.,1.,1.,1.,1.,1.,1.,1.,1.,1.,1.,1.,1.,1.,1.,
1.,1.,1.,1.,1.,1.,1.,1.,1.,1.,1.,1.,1.,1.,1.,1.,1.,1.,1.,1.,1.,1.,1.,1.,
1.,1.,1.,1.,1.,1.,1.,1.,1.,1.,1.,1.,1.,1.,1.,1.,1.,1.,1.,1.,1.,1.,1.,1.,
1.,1.,1.,1.,1.,1.))
REPRESENTATION_ITEM('')
);
#193=(
BOUNDED_CURVE()
B_SPLINE_CURVE(5,(#34625,#34626,#34627,#34628,#34629,#34630,#34631,#34632,
#34633,#34634,#34635,#34636,#34637,#34638,#34639,#34640,#34641,#34642,#34643,
#34644,#34645,#34646,#34647,#34648,#34649,#34650,#34651,#34652,#34653,#34654,
#34655,#34656,#34657,#34658,#34659,#34660,#34661,#34662,#34663,#34664,#34665,
#34666,#34667,#34668,#34669,#34670,#34671,#34672,#34673,#34674,#34675,#34676,
#34677,#34678,#34679,#34680,#34681,#34682,#34683,#34684,#34685,#34686,#34687,
#34688,#34689,#34690,#34691,#34692,#34693,#34694),.UNSPECIFIED.,.F.,.F.)
B_SPLINE_CURVE_WITH_KNOTS((6,1,1,1,1,1,1,1,1,1,1,1,1,1,1,1,1,1,1,1,1,1,
1,1,1,1,1,1,1,1,1,1,1,1,1,1,1,1,1,1,1,1,1,1,1,1,1,1,1,1,1,1,1,1,1,1,1,1,
1,1,1,1,1,1,1,6),(-1.,-0.984615384615383,-0.969230769230768,-0.953846153846152,
-0.938461538461537,-0.923076923076922,-0.907692307692306,-0.892307692307691,
-0.876923076923076,-0.86153846153846,-0.846153846153845,-0.83076923076923,
-0.815384615384614,-0.799999999999999,-0.784615384615384,-0.769230769230768,
-0.753846153846153,-0.738461538461538,-0.723076923076922,-0.707692307692307,
-0.692307692307692,-0.676923076923076,-0.661538461538461,-0.646153846153846,
-0.63076923076923,-0.615384615384615,-0.6,-0.584615384615384,-0.569230769230769,
-0.553846153846154,-0.538461538461538,-0.523076923076923,-0.507692307692308,
-0.492307692307692,-0.476923076923077,-0.461538461538462,-0.446153846153846,
-0.430769230769231,-0.415384615384615,-0.4,-0.384615384615385,-0.369230769230769,
-0.353846153846154,-0.338461538461538,-0.323076923076923,-0.307692307692308,
-0.292307692307692,-0.276923076923077,-0.261538461538462,-0.246153846153846,
-0.230769230769231,-0.215384615384615,-0.2,-0.184615384615385,-0.169230769230769,
-0.153846153846154,-0.138461538461538,-0.123076923076923,-0.107692307692308,
-0.0923076923076923,-0.0769230769230769,-0.0615384615384615,-0.0461538461538462,
-0.0307692307692308,-0.0153846153846154,0.),.UNSPECIFIED.)
CURVE()
GEOMETRIC_REPRESENTATION_ITEM()
RATIONAL_B_SPLINE_CURVE((1.,1.,1.,1.,1.,1.,1.,1.,1.,1.,1.,1.,1.,1.,1.,1.,
1.,1.,1.,1.,1.,1.,1.,1.,1.,1.,1.,1.,1.,1.,1.,1.,1.,1.,1.,1.,1.,1.,1.,1.,
1.,1.,1.,1.,1.,1.,1.,1.,1.,1.,1.,1.,1.,1.,1.,1.,1.,1.,1.,1.,1.,1.,1.,1.,
1.,1.,1.,1.,1.,1.))
REPRESENTATION_ITEM('')
);
#194=(
BOUNDED_CURVE()
B_SPLINE_CURVE(5,(#34841,#34842,#34843,#34844,#34845,#34846,#34847,#34848,
#34849,#34850,#34851,#34852,#34853,#34854,#34855,#34856,#34857,#34858,#34859,
#34860,#34861,#34862,#34863,#34864,#34865,#34866,#34867,#34868,#34869,#34870,
#34871,#34872,#34873,#34874,#34875,#34876,#34877,#34878,#34879,#34880,#34881,
#34882,#34883,#34884,#34885,#34886,#34887,#34888,#34889,#34890,#34891,#34892,
#34893,#34894,#34895,#34896,#34897,#34898,#34899,#34900,#34901,#34902,#34903,
#34904,#34905,#34906,#34907,#34908,#34909,#34910),.UNSPECIFIED.,.F.,.F.)
B_SPLINE_CURVE_WITH_KNOTS((6,1,1,1,1,1,1,1,1,1,1,1,1,1,1,1,1,1,1,1,1,1,
1,1,1,1,1,1,1,1,1,1,1,1,1,1,1,1,1,1,1,1,1,1,1,1,1,1,1,1,1,1,1,1,1,1,1,1,
1,1,1,1,1,1,1,6),(-1.,-0.984615384615383,-0.969230769230768,-0.953846153846152,
-0.938461538461537,-0.923076923076922,-0.907692307692306,-0.892307692307691,
-0.876923076923076,-0.86153846153846,-0.846153846153845,-0.83076923076923,
-0.815384615384614,-0.799999999999999,-0.784615384615384,-0.769230769230768,
-0.753846153846153,-0.738461538461538,-0.723076923076922,-0.707692307692307,
-0.692307692307692,-0.676923076923076,-0.661538461538461,-0.646153846153846,
-0.63076923076923,-0.615384615384615,-0.6,-0.584615384615384,-0.569230769230769,
-0.553846153846154,-0.538461538461538,-0.523076923076923,-0.507692307692308,
-0.492307692307692,-0.476923076923077,-0.461538461538462,-0.446153846153846,
-0.430769230769231,-0.415384615384615,-0.4,-0.384615384615385,-0.369230769230769,
-0.353846153846154,-0.338461538461538,-0.323076923076923,-0.307692307692308,
-0.292307692307692,-0.276923076923077,-0.261538461538462,-0.246153846153846,
-0.230769230769231,-0.215384615384615,-0.2,-0.184615384615385,-0.169230769230769,
-0.153846153846154,-0.138461538461538,-0.123076923076923,-0.107692307692308,
-0.0923076923076923,-0.0769230769230769,-0.0615384615384615,-0.0461538461538462,
-0.0307692307692308,-0.0153846153846154,0.),.UNSPECIFIED.)
CURVE()
GEOMETRIC_REPRESENTATION_ITEM()
RATIONAL_B_SPLINE_CURVE((1.,1.,1.,1.,1.,1.,1.,1.,1.,1.,1.,1.,1.,1.,1.,1.,
1.,1.,1.,1.,1.,1.,1.,1.,1.,1.,1.,1.,1.,1.,1.,1.,1.,1.,1.,1.,1.,1.,1.,1.,
1.,1.,1.,1.,1.,1.,1.,1.,1.,1.,1.,1.,1.,1.,1.,1.,1.,1.,1.,1.,1.,1.,1.,1.,
1.,1.,1.,1.,1.,1.))
REPRESENTATION_ITEM('')
);
#195=(
BOUNDED_CURVE()
B_SPLINE_CURVE(5,(#35057,#35058,#35059,#35060,#35061,#35062,#35063,#35064,
#35065,#35066,#35067,#35068,#35069,#35070,#35071,#35072,#35073,#35074,#35075,
#35076,#35077,#35078,#35079,#35080,#35081,#35082,#35083,#35084,#35085,#35086,
#35087,#35088,#35089,#35090,#35091,#35092,#35093,#35094,#35095,#35096,#35097,
#35098,#35099,#35100,#35101,#35102,#35103,#35104,#35105,#35106,#35107,#35108,
#35109,#35110,#35111,#35112,#35113,#35114,#35115,#35116,#35117,#35118,#35119,
#35120,#35121,#35122,#35123,#35124,#35125,#35126),.UNSPECIFIED.,.F.,.F.)
B_SPLINE_CURVE_WITH_KNOTS((6,1,1,1,1,1,1,1,1,1,1,1,1,1,1,1,1,1,1,1,1,1,
1,1,1,1,1,1,1,1,1,1,1,1,1,1,1,1,1,1,1,1,1,1,1,1,1,1,1,1,1,1,1,1,1,1,1,1,
1,1,1,1,1,1,1,6),(-1.,-0.984615384615383,-0.969230769230768,-0.953846153846152,
-0.938461538461537,-0.923076923076922,-0.907692307692306,-0.892307692307691,
-0.876923076923076,-0.86153846153846,-0.846153846153845,-0.83076923076923,
-0.815384615384614,-0.799999999999999,-0.784615384615384,-0.769230769230768,
-0.753846153846153,-0.738461538461538,-0.723076923076922,-0.707692307692307,
-0.692307692307692,-0.676923076923076,-0.661538461538461,-0.646153846153846,
-0.63076923076923,-0.615384615384615,-0.6,-0.584615384615384,-0.569230769230769,
-0.553846153846154,-0.538461538461538,-0.523076923076923,-0.507692307692308,
-0.492307692307692,-0.476923076923077,-0.461538461538462,-0.446153846153846,
-0.430769230769231,-0.415384615384615,-0.4,-0.384615384615385,-0.369230769230769,
-0.353846153846154,-0.338461538461538,-0.323076923076923,-0.307692307692308,
-0.292307692307692,-0.276923076923077,-0.261538461538462,-0.246153846153846,
-0.230769230769231,-0.215384615384615,-0.2,-0.184615384615385,-0.169230769230769,
-0.153846153846154,-0.138461538461538,-0.123076923076923,-0.107692307692308,
-0.0923076923076923,-0.0769230769230769,-0.0615384615384615,-0.0461538461538462,
-0.0307692307692308,-0.0153846153846154,0.),.UNSPECIFIED.)
CURVE()
GEOMETRIC_REPRESENTATION_ITEM()
RATIONAL_B_SPLINE_CURVE((1.,1.,1.,1.,1.,1.,1.,1.,1.,1.,1.,1.,1.,1.,1.,1.,
1.,1.,1.,1.,1.,1.,1.,1.,1.,1.,1.,1.,1.,1.,1.,1.,1.,1.,1.,1.,1.,1.,1.,1.,
1.,1.,1.,1.,1.,1.,1.,1.,1.,1.,1.,1.,1.,1.,1.,1.,1.,1.,1.,1.,1.,1.,1.,1.,
1.,1.,1.,1.,1.,1.))
REPRESENTATION_ITEM('')
);
#196=(
BOUNDED_CURVE()
B_SPLINE_CURVE(5,(#35273,#35274,#35275,#35276,#35277,#35278,#35279,#35280,
#35281,#35282,#35283,#35284,#35285,#35286,#35287,#35288,#35289,#35290,#35291,
#35292,#35293,#35294,#35295,#35296,#35297,#35298,#35299,#35300,#35301,#35302,
#35303,#35304,#35305,#35306,#35307,#35308,#35309,#35310,#35311,#35312,#35313,
#35314,#35315,#35316,#35317,#35318,#35319,#35320,#35321,#35322,#35323,#35324,
#35325,#35326,#35327,#35328,#35329,#35330,#35331,#35332,#35333,#35334,#35335,
#35336,#35337,#35338,#35339,#35340,#35341,#35342),.UNSPECIFIED.,.F.,.F.)
B_SPLINE_CURVE_WITH_KNOTS((6,1,1,1,1,1,1,1,1,1,1,1,1,1,1,1,1,1,1,1,1,1,
1,1,1,1,1,1,1,1,1,1,1,1,1,1,1,1,1,1,1,1,1,1,1,1,1,1,1,1,1,1,1,1,1,1,1,1,
1,1,1,1,1,1,1,6),(-1.,-0.984615384615383,-0.969230769230768,-0.953846153846152,
-0.938461538461537,-0.923076923076922,-0.907692307692306,-0.892307692307691,
-0.876923076923076,-0.86153846153846,-0.846153846153845,-0.83076923076923,
-0.815384615384614,-0.799999999999999,-0.784615384615384,-0.769230769230768,
-0.753846153846153,-0.738461538461538,-0.723076923076922,-0.707692307692307,
-0.692307692307692,-0.676923076923076,-0.661538461538461,-0.646153846153846,
-0.63076923076923,-0.615384615384615,-0.6,-0.584615384615384,-0.569230769230769,
-0.553846153846154,-0.538461538461538,-0.523076923076923,-0.507692307692308,
-0.492307692307692,-0.476923076923077,-0.461538461538462,-0.446153846153846,
-0.430769230769231,-0.415384615384615,-0.4,-0.384615384615385,-0.369230769230769,
-0.353846153846154,-0.338461538461538,-0.323076923076923,-0.307692307692308,
-0.292307692307692,-0.276923076923077,-0.261538461538462,-0.246153846153846,
-0.230769230769231,-0.215384615384615,-0.2,-0.184615384615385,-0.169230769230769,
-0.153846153846154,-0.138461538461538,-0.123076923076923,-0.107692307692308,
-0.0923076923076923,-0.0769230769230769,-0.0615384615384615,-0.0461538461538462,
-0.0307692307692308,-0.0153846153846154,0.),.UNSPECIFIED.)
CURVE()
GEOMETRIC_REPRESENTATION_ITEM()
RATIONAL_B_SPLINE_CURVE((1.,1.,1.,1.,1.,1.,1.,1.,1.,1.,1.,1.,1.,1.,1.,1.,
1.,1.,1.,1.,1.,1.,1.,1.,1.,1.,1.,1.,1.,1.,1.,1.,1.,1.,1.,1.,1.,1.,1.,1.,
1.,1.,1.,1.,1.,1.,1.,1.,1.,1.,1.,1.,1.,1.,1.,1.,1.,1.,1.,1.,1.,1.,1.,1.,
1.,1.,1.,1.,1.,1.))
REPRESENTATION_ITEM('')
);
#197=(
BOUNDED_CURVE()
B_SPLINE_CURVE(5,(#35489,#35490,#35491,#35492,#35493,#35494,#35495,#35496,
#35497,#35498,#35499,#35500,#35501,#35502,#35503,#35504,#35505,#35506,#35507,
#35508,#35509,#35510,#35511,#35512,#35513,#35514,#35515,#35516,#35517,#35518,
#35519,#35520,#35521,#35522,#35523,#35524,#35525,#35526,#35527,#35528,#35529,
#35530,#35531,#35532,#35533,#35534,#35535,#35536,#35537,#35538,#35539,#35540,
#35541,#35542,#35543,#35544,#35545,#35546,#35547,#35548,#35549,#35550,#35551,
#35552,#35553,#35554,#35555,#35556,#35557,#35558),.UNSPECIFIED.,.F.,.F.)
B_SPLINE_CURVE_WITH_KNOTS((6,1,1,1,1,1,1,1,1,1,1,1,1,1,1,1,1,1,1,1,1,1,
1,1,1,1,1,1,1,1,1,1,1,1,1,1,1,1,1,1,1,1,1,1,1,1,1,1,1,1,1,1,1,1,1,1,1,1,
1,1,1,1,1,1,1,6),(-1.,-0.984615384615383,-0.969230769230768,-0.953846153846152,
-0.938461538461537,-0.923076923076922,-0.907692307692306,-0.892307692307691,
-0.876923076923076,-0.86153846153846,-0.846153846153845,-0.83076923076923,
-0.815384615384614,-0.799999999999999,-0.784615384615384,-0.769230769230768,
-0.753846153846153,-0.738461538461538,-0.723076923076922,-0.707692307692307,
-0.692307692307692,-0.676923076923076,-0.661538461538461,-0.646153846153846,
-0.63076923076923,-0.615384615384615,-0.6,-0.584615384615384,-0.569230769230769,
-0.553846153846154,-0.538461538461538,-0.523076923076923,-0.507692307692308,
-0.492307692307692,-0.476923076923077,-0.461538461538462,-0.446153846153846,
-0.430769230769231,-0.415384615384615,-0.4,-0.384615384615385,-0.369230769230769,
-0.353846153846154,-0.338461538461538,-0.323076923076923,-0.307692307692308,
-0.292307692307692,-0.276923076923077,-0.261538461538462,-0.246153846153846,
-0.230769230769231,-0.215384615384615,-0.2,-0.184615384615385,-0.169230769230769,
-0.153846153846154,-0.138461538461538,-0.123076923076923,-0.107692307692308,
-0.0923076923076923,-0.0769230769230769,-0.0615384615384615,-0.0461538461538462,
-0.0307692307692308,-0.0153846153846154,0.),.UNSPECIFIED.)
CURVE()
GEOMETRIC_REPRESENTATION_ITEM()
RATIONAL_B_SPLINE_CURVE((1.,1.,1.,1.,1.,1.,1.,1.,1.,1.,1.,1.,1.,1.,1.,1.,
1.,1.,1.,1.,1.,1.,1.,1.,1.,1.,1.,1.,1.,1.,1.,1.,1.,1.,1.,1.,1.,1.,1.,1.,
1.,1.,1.,1.,1.,1.,1.,1.,1.,1.,1.,1.,1.,1.,1.,1.,1.,1.,1.,1.,1.,1.,1.,1.,
1.,1.,1.,1.,1.,1.))
REPRESENTATION_ITEM('')
);
#198=(
BOUNDED_CURVE()
B_SPLINE_CURVE(5,(#35705,#35706,#35707,#35708,#35709,#35710,#35711,#35712,
#35713,#35714,#35715,#35716,#35717,#35718,#35719,#35720,#35721,#35722,#35723,
#35724,#35725,#35726,#35727,#35728,#35729,#35730,#35731,#35732,#35733,#35734,
#35735,#35736,#35737,#35738,#35739,#35740,#35741,#35742,#35743,#35744,#35745,
#35746,#35747,#35748,#35749,#35750,#35751,#35752,#35753,#35754,#35755,#35756,
#35757,#35758,#35759,#35760,#35761,#35762,#35763,#35764,#35765,#35766,#35767,
#35768,#35769,#35770,#35771,#35772,#35773,#35774),.UNSPECIFIED.,.F.,.F.)
B_SPLINE_CURVE_WITH_KNOTS((6,1,1,1,1,1,1,1,1,1,1,1,1,1,1,1,1,1,1,1,1,1,
1,1,1,1,1,1,1,1,1,1,1,1,1,1,1,1,1,1,1,1,1,1,1,1,1,1,1,1,1,1,1,1,1,1,1,1,
1,1,1,1,1,1,1,6),(-1.,-0.984615384615383,-0.969230769230768,-0.953846153846152,
-0.938461538461537,-0.923076923076922,-0.907692307692306,-0.892307692307691,
-0.876923076923076,-0.86153846153846,-0.846153846153845,-0.83076923076923,
-0.815384615384614,-0.799999999999999,-0.784615384615384,-0.769230769230768,
-0.753846153846153,-0.738461538461538,-0.723076923076922,-0.707692307692307,
-0.692307692307692,-0.676923076923076,-0.661538461538461,-0.646153846153846,
-0.63076923076923,-0.615384615384615,-0.6,-0.584615384615384,-0.569230769230769,
-0.553846153846154,-0.538461538461538,-0.523076923076923,-0.507692307692308,
-0.492307692307692,-0.476923076923077,-0.461538461538462,-0.446153846153846,
-0.430769230769231,-0.415384615384615,-0.4,-0.384615384615385,-0.369230769230769,
-0.353846153846154,-0.338461538461538,-0.323076923076923,-0.307692307692308,
-0.292307692307692,-0.276923076923077,-0.261538461538462,-0.246153846153846,
-0.230769230769231,-0.215384615384615,-0.2,-0.184615384615385,-0.169230769230769,
-0.153846153846154,-0.138461538461538,-0.123076923076923,-0.107692307692308,
-0.0923076923076923,-0.0769230769230769,-0.0615384615384615,-0.0461538461538462,
-0.0307692307692308,-0.0153846153846154,0.),.UNSPECIFIED.)
CURVE()
GEOMETRIC_REPRESENTATION_ITEM()
RATIONAL_B_SPLINE_CURVE((1.,1.,1.,1.,1.,1.,1.,1.,1.,1.,1.,1.,1.,1.,1.,1.,
1.,1.,1.,1.,1.,1.,1.,1.,1.,1.,1.,1.,1.,1.,1.,1.,1.,1.,1.,1.,1.,1.,1.,1.,
1.,1.,1.,1.,1.,1.,1.,1.,1.,1.,1.,1.,1.,1.,1.,1.,1.,1.,1.,1.,1.,1.,1.,1.,
1.,1.,1.,1.,1.,1.))
REPRESENTATION_ITEM('')
);
#199=(
BOUNDED_CURVE()
B_SPLINE_CURVE(5,(#35921,#35922,#35923,#35924,#35925,#35926,#35927,#35928,
#35929,#35930,#35931,#35932,#35933,#35934,#35935,#35936,#35937,#35938,#35939,
#35940,#35941,#35942,#35943,#35944,#35945,#35946,#35947,#35948,#35949,#35950,
#35951,#35952,#35953,#35954,#35955,#35956,#35957,#35958,#35959,#35960,#35961,
#35962,#35963,#35964,#35965,#35966,#35967,#35968,#35969,#35970,#35971,#35972,
#35973,#35974,#35975,#35976,#35977,#35978,#35979,#35980,#35981,#35982,#35983,
#35984,#35985,#35986,#35987,#35988,#35989,#35990),.UNSPECIFIED.,.F.,.F.)
B_SPLINE_CURVE_WITH_KNOTS((6,1,1,1,1,1,1,1,1,1,1,1,1,1,1,1,1,1,1,1,1,1,
1,1,1,1,1,1,1,1,1,1,1,1,1,1,1,1,1,1,1,1,1,1,1,1,1,1,1,1,1,1,1,1,1,1,1,1,
1,1,1,1,1,1,1,6),(-1.,-0.984615384615383,-0.969230769230768,-0.953846153846152,
-0.938461538461537,-0.923076923076922,-0.907692307692306,-0.892307692307691,
-0.876923076923076,-0.86153846153846,-0.846153846153845,-0.83076923076923,
-0.815384615384614,-0.799999999999999,-0.784615384615384,-0.769230769230768,
-0.753846153846153,-0.738461538461538,-0.723076923076922,-0.707692307692307,
-0.692307692307692,-0.676923076923076,-0.661538461538461,-0.646153846153846,
-0.63076923076923,-0.615384615384615,-0.6,-0.584615384615384,-0.569230769230769,
-0.553846153846154,-0.538461538461538,-0.523076923076923,-0.507692307692308,
-0.492307692307692,-0.476923076923077,-0.461538461538462,-0.446153846153846,
-0.430769230769231,-0.415384615384615,-0.4,-0.384615384615385,-0.369230769230769,
-0.353846153846154,-0.338461538461538,-0.323076923076923,-0.307692307692308,
-0.292307692307692,-0.276923076923077,-0.261538461538462,-0.246153846153846,
-0.230769230769231,-0.215384615384615,-0.2,-0.184615384615385,-0.169230769230769,
-0.153846153846154,-0.138461538461538,-0.123076923076923,-0.107692307692308,
-0.0923076923076923,-0.0769230769230769,-0.0615384615384615,-0.0461538461538462,
-0.0307692307692308,-0.0153846153846154,0.),.UNSPECIFIED.)
CURVE()
GEOMETRIC_REPRESENTATION_ITEM()
RATIONAL_B_SPLINE_CURVE((1.,1.,1.,1.,1.,1.,1.,1.,1.,1.,1.,1.,1.,1.,1.,1.,
1.,1.,1.,1.,1.,1.,1.,1.,1.,1.,1.,1.,1.,1.,1.,1.,1.,1.,1.,1.,1.,1.,1.,1.,
1.,1.,1.,1.,1.,1.,1.,1.,1.,1.,1.,1.,1.,1.,1.,1.,1.,1.,1.,1.,1.,1.,1.,1.,
1.,1.,1.,1.,1.,1.))
REPRESENTATION_ITEM('')
);
#200=(
BOUNDED_CURVE()
B_SPLINE_CURVE(5,(#36137,#36138,#36139,#36140,#36141,#36142,#36143,#36144,
#36145,#36146,#36147,#36148,#36149,#36150,#36151,#36152,#36153,#36154,#36155,
#36156,#36157,#36158,#36159,#36160,#36161,#36162,#36163,#36164,#36165,#36166,
#36167,#36168,#36169,#36170,#36171,#36172,#36173,#36174,#36175,#36176,#36177,
#36178,#36179,#36180,#36181,#36182,#36183,#36184,#36185,#36186,#36187,#36188,
#36189,#36190,#36191,#36192,#36193,#36194,#36195,#36196,#36197,#36198,#36199,
#36200,#36201,#36202,#36203,#36204,#36205,#36206),.UNSPECIFIED.,.F.,.F.)
B_SPLINE_CURVE_WITH_KNOTS((6,1,1,1,1,1,1,1,1,1,1,1,1,1,1,1,1,1,1,1,1,1,
1,1,1,1,1,1,1,1,1,1,1,1,1,1,1,1,1,1,1,1,1,1,1,1,1,1,1,1,1,1,1,1,1,1,1,1,
1,1,1,1,1,1,1,6),(-1.,-0.984615384615383,-0.969230769230768,-0.953846153846152,
-0.938461538461537,-0.923076923076922,-0.907692307692306,-0.892307692307691,
-0.876923076923076,-0.86153846153846,-0.846153846153845,-0.83076923076923,
-0.815384615384614,-0.799999999999999,-0.784615384615384,-0.769230769230768,
-0.753846153846153,-0.738461538461538,-0.723076923076922,-0.707692307692307,
-0.692307692307692,-0.676923076923076,-0.661538461538461,-0.646153846153846,
-0.63076923076923,-0.615384615384615,-0.6,-0.584615384615384,-0.569230769230769,
-0.553846153846154,-0.538461538461538,-0.523076923076923,-0.507692307692308,
-0.492307692307692,-0.476923076923077,-0.461538461538462,-0.446153846153846,
-0.430769230769231,-0.415384615384615,-0.4,-0.384615384615385,-0.369230769230769,
-0.353846153846154,-0.338461538461538,-0.323076923076923,-0.307692307692308,
-0.292307692307692,-0.276923076923077,-0.261538461538462,-0.246153846153846,
-0.230769230769231,-0.215384615384615,-0.2,-0.184615384615385,-0.169230769230769,
-0.153846153846154,-0.138461538461538,-0.123076923076923,-0.107692307692308,
-0.0923076923076923,-0.0769230769230769,-0.0615384615384615,-0.0461538461538462,
-0.0307692307692308,-0.0153846153846154,0.),.UNSPECIFIED.)
CURVE()
GEOMETRIC_REPRESENTATION_ITEM()
RATIONAL_B_SPLINE_CURVE((1.,1.,1.,1.,1.,1.,1.,1.,1.,1.,1.,1.,1.,1.,1.,1.,
1.,1.,1.,1.,1.,1.,1.,1.,1.,1.,1.,1.,1.,1.,1.,1.,1.,1.,1.,1.,1.,1.,1.,1.,
1.,1.,1.,1.,1.,1.,1.,1.,1.,1.,1.,1.,1.,1.,1.,1.,1.,1.,1.,1.,1.,1.,1.,1.,
1.,1.,1.,1.,1.,1.))
REPRESENTATION_ITEM('')
);
#201=(
BOUNDED_CURVE()
B_SPLINE_CURVE(5,(#36353,#36354,#36355,#36356,#36357,#36358,#36359,#36360,
#36361,#36362,#36363,#36364,#36365,#36366,#36367,#36368,#36369,#36370,#36371,
#36372,#36373,#36374,#36375,#36376,#36377,#36378,#36379,#36380,#36381,#36382,
#36383,#36384,#36385,#36386,#36387,#36388,#36389,#36390,#36391,#36392,#36393,
#36394,#36395,#36396,#36397,#36398,#36399,#36400,#36401,#36402,#36403,#36404,
#36405,#36406,#36407,#36408,#36409,#36410,#36411,#36412,#36413,#36414,#36415,
#36416,#36417,#36418,#36419,#36420,#36421,#36422),.UNSPECIFIED.,.F.,.F.)
B_SPLINE_CURVE_WITH_KNOTS((6,1,1,1,1,1,1,1,1,1,1,1,1,1,1,1,1,1,1,1,1,1,
1,1,1,1,1,1,1,1,1,1,1,1,1,1,1,1,1,1,1,1,1,1,1,1,1,1,1,1,1,1,1,1,1,1,1,1,
1,1,1,1,1,1,1,6),(-1.,-0.984615384615383,-0.969230769230768,-0.953846153846152,
-0.938461538461537,-0.923076923076922,-0.907692307692306,-0.892307692307691,
-0.876923076923076,-0.86153846153846,-0.846153846153845,-0.83076923076923,
-0.815384615384614,-0.799999999999999,-0.784615384615384,-0.769230769230768,
-0.753846153846153,-0.738461538461538,-0.723076923076922,-0.707692307692307,
-0.692307692307692,-0.676923076923076,-0.661538461538461,-0.646153846153846,
-0.63076923076923,-0.615384615384615,-0.6,-0.584615384615384,-0.569230769230769,
-0.553846153846154,-0.538461538461538,-0.523076923076923,-0.507692307692308,
-0.492307692307692,-0.476923076923077,-0.461538461538462,-0.446153846153846,
-0.430769230769231,-0.415384615384615,-0.4,-0.384615384615385,-0.369230769230769,
-0.353846153846154,-0.338461538461538,-0.323076923076923,-0.307692307692308,
-0.292307692307692,-0.276923076923077,-0.261538461538462,-0.246153846153846,
-0.230769230769231,-0.215384615384615,-0.2,-0.184615384615385,-0.169230769230769,
-0.153846153846154,-0.138461538461538,-0.123076923076923,-0.107692307692308,
-0.0923076923076923,-0.0769230769230769,-0.0615384615384615,-0.0461538461538462,
-0.0307692307692308,-0.0153846153846154,0.),.UNSPECIFIED.)
CURVE()
GEOMETRIC_REPRESENTATION_ITEM()
RATIONAL_B_SPLINE_CURVE((1.,1.,1.,1.,1.,1.,1.,1.,1.,1.,1.,1.,1.,1.,1.,1.,
1.,1.,1.,1.,1.,1.,1.,1.,1.,1.,1.,1.,1.,1.,1.,1.,1.,1.,1.,1.,1.,1.,1.,1.,
1.,1.,1.,1.,1.,1.,1.,1.,1.,1.,1.,1.,1.,1.,1.,1.,1.,1.,1.,1.,1.,1.,1.,1.,
1.,1.,1.,1.,1.,1.))
REPRESENTATION_ITEM('')
);
#202=(
BOUNDED_CURVE()
B_SPLINE_CURVE(5,(#36569,#36570,#36571,#36572,#36573,#36574,#36575,#36576,
#36577,#36578,#36579,#36580,#36581,#36582,#36583,#36584,#36585,#36586,#36587,
#36588,#36589,#36590,#36591,#36592,#36593,#36594,#36595,#36596,#36597,#36598,
#36599,#36600,#36601,#36602,#36603,#36604,#36605,#36606,#36607,#36608,#36609,
#36610,#36611,#36612,#36613,#36614,#36615,#36616,#36617,#36618,#36619,#36620,
#36621,#36622,#36623,#36624,#36625,#36626,#36627,#36628,#36629,#36630,#36631,
#36632,#36633,#36634,#36635,#36636,#36637,#36638),.UNSPECIFIED.,.F.,.F.)
B_SPLINE_CURVE_WITH_KNOTS((6,1,1,1,1,1,1,1,1,1,1,1,1,1,1,1,1,1,1,1,1,1,
1,1,1,1,1,1,1,1,1,1,1,1,1,1,1,1,1,1,1,1,1,1,1,1,1,1,1,1,1,1,1,1,1,1,1,1,
1,1,1,1,1,1,1,6),(-1.,-0.984615384615383,-0.969230769230768,-0.953846153846152,
-0.938461538461537,-0.923076923076922,-0.907692307692306,-0.892307692307691,
-0.876923076923076,-0.86153846153846,-0.846153846153845,-0.83076923076923,
-0.815384615384614,-0.799999999999999,-0.784615384615384,-0.769230769230768,
-0.753846153846153,-0.738461538461538,-0.723076923076922,-0.707692307692307,
-0.692307692307692,-0.676923076923076,-0.661538461538461,-0.646153846153846,
-0.63076923076923,-0.615384615384615,-0.6,-0.584615384615384,-0.569230769230769,
-0.553846153846154,-0.538461538461538,-0.523076923076923,-0.507692307692308,
-0.492307692307692,-0.476923076923077,-0.461538461538462,-0.446153846153846,
-0.430769230769231,-0.415384615384615,-0.4,-0.384615384615385,-0.369230769230769,
-0.353846153846154,-0.338461538461538,-0.323076923076923,-0.307692307692308,
-0.292307692307692,-0.276923076923077,-0.261538461538462,-0.246153846153846,
-0.230769230769231,-0.215384615384615,-0.2,-0.184615384615385,-0.169230769230769,
-0.153846153846154,-0.138461538461538,-0.123076923076923,-0.107692307692308,
-0.0923076923076923,-0.0769230769230769,-0.0615384615384615,-0.0461538461538462,
-0.0307692307692308,-0.0153846153846154,0.),.UNSPECIFIED.)
CURVE()
GEOMETRIC_REPRESENTATION_ITEM()
RATIONAL_B_SPLINE_CURVE((1.,1.,1.,1.,1.,1.,1.,1.,1.,1.,1.,1.,1.,1.,1.,1.,
1.,1.,1.,1.,1.,1.,1.,1.,1.,1.,1.,1.,1.,1.,1.,1.,1.,1.,1.,1.,1.,1.,1.,1.,
1.,1.,1.,1.,1.,1.,1.,1.,1.,1.,1.,1.,1.,1.,1.,1.,1.,1.,1.,1.,1.,1.,1.,1.,
1.,1.,1.,1.,1.,1.))
REPRESENTATION_ITEM('')
);
#203=(
BOUNDED_CURVE()
B_SPLINE_CURVE(5,(#36785,#36786,#36787,#36788,#36789,#36790,#36791,#36792,
#36793,#36794,#36795,#36796,#36797,#36798,#36799,#36800,#36801,#36802,#36803,
#36804,#36805,#36806,#36807,#36808,#36809,#36810,#36811,#36812,#36813,#36814,
#36815,#36816,#36817,#36818,#36819,#36820,#36821,#36822,#36823,#36824,#36825,
#36826,#36827,#36828,#36829,#36830,#36831,#36832,#36833,#36834,#36835,#36836,
#36837,#36838,#36839,#36840,#36841,#36842,#36843,#36844,#36845,#36846,#36847,
#36848,#36849,#36850,#36851,#36852,#36853,#36854),.UNSPECIFIED.,.F.,.F.)
B_SPLINE_CURVE_WITH_KNOTS((6,1,1,1,1,1,1,1,1,1,1,1,1,1,1,1,1,1,1,1,1,1,
1,1,1,1,1,1,1,1,1,1,1,1,1,1,1,1,1,1,1,1,1,1,1,1,1,1,1,1,1,1,1,1,1,1,1,1,
1,1,1,1,1,1,1,6),(-1.,-0.984615384615383,-0.969230769230768,-0.953846153846152,
-0.938461538461537,-0.923076923076922,-0.907692307692306,-0.892307692307691,
-0.876923076923076,-0.86153846153846,-0.846153846153845,-0.83076923076923,
-0.815384615384614,-0.799999999999999,-0.784615384615384,-0.769230769230768,
-0.753846153846153,-0.738461538461538,-0.723076923076922,-0.707692307692307,
-0.692307692307692,-0.676923076923076,-0.661538461538461,-0.646153846153846,
-0.63076923076923,-0.615384615384615,-0.6,-0.584615384615384,-0.569230769230769,
-0.553846153846154,-0.538461538461538,-0.523076923076923,-0.507692307692308,
-0.492307692307692,-0.476923076923077,-0.461538461538462,-0.446153846153846,
-0.430769230769231,-0.415384615384615,-0.4,-0.384615384615385,-0.369230769230769,
-0.353846153846154,-0.338461538461538,-0.323076923076923,-0.307692307692308,
-0.292307692307692,-0.276923076923077,-0.261538461538462,-0.246153846153846,
-0.230769230769231,-0.215384615384615,-0.2,-0.184615384615385,-0.169230769230769,
-0.153846153846154,-0.138461538461538,-0.123076923076923,-0.107692307692308,
-0.0923076923076923,-0.0769230769230769,-0.0615384615384615,-0.0461538461538462,
-0.0307692307692308,-0.0153846153846154,0.),.UNSPECIFIED.)
CURVE()
GEOMETRIC_REPRESENTATION_ITEM()
RATIONAL_B_SPLINE_CURVE((1.,1.,1.,1.,1.,1.,1.,1.,1.,1.,1.,1.,1.,1.,1.,1.,
1.,1.,1.,1.,1.,1.,1.,1.,1.,1.,1.,1.,1.,1.,1.,1.,1.,1.,1.,1.,1.,1.,1.,1.,
1.,1.,1.,1.,1.,1.,1.,1.,1.,1.,1.,1.,1.,1.,1.,1.,1.,1.,1.,1.,1.,1.,1.,1.,
1.,1.,1.,1.,1.,1.))
REPRESENTATION_ITEM('')
);
#204=(
BOUNDED_CURVE()
B_SPLINE_CURVE(5,(#37001,#37002,#37003,#37004,#37005,#37006,#37007,#37008,
#37009,#37010,#37011,#37012,#37013,#37014,#37015,#37016,#37017,#37018,#37019,
#37020,#37021,#37022,#37023,#37024,#37025,#37026,#37027,#37028,#37029,#37030,
#37031,#37032,#37033,#37034,#37035,#37036,#37037,#37038,#37039,#37040,#37041,
#37042,#37043,#37044,#37045,#37046,#37047,#37048,#37049,#37050,#37051,#37052,
#37053,#37054,#37055,#37056,#37057,#37058,#37059,#37060,#37061,#37062,#37063,
#37064,#37065,#37066,#37067,#37068,#37069,#37070),.UNSPECIFIED.,.F.,.F.)
B_SPLINE_CURVE_WITH_KNOTS((6,1,1,1,1,1,1,1,1,1,1,1,1,1,1,1,1,1,1,1,1,1,
1,1,1,1,1,1,1,1,1,1,1,1,1,1,1,1,1,1,1,1,1,1,1,1,1,1,1,1,1,1,1,1,1,1,1,1,
1,1,1,1,1,1,1,6),(-1.,-0.984615384615383,-0.969230769230768,-0.953846153846152,
-0.938461538461537,-0.923076923076922,-0.907692307692306,-0.892307692307691,
-0.876923076923076,-0.86153846153846,-0.846153846153845,-0.83076923076923,
-0.815384615384614,-0.799999999999999,-0.784615384615384,-0.769230769230768,
-0.753846153846153,-0.738461538461538,-0.723076923076922,-0.707692307692307,
-0.692307692307692,-0.676923076923076,-0.661538461538461,-0.646153846153846,
-0.63076923076923,-0.615384615384615,-0.6,-0.584615384615384,-0.569230769230769,
-0.553846153846154,-0.538461538461538,-0.523076923076923,-0.507692307692308,
-0.492307692307692,-0.476923076923077,-0.461538461538462,-0.446153846153846,
-0.430769230769231,-0.415384615384615,-0.4,-0.384615384615385,-0.369230769230769,
-0.353846153846154,-0.338461538461538,-0.323076923076923,-0.307692307692308,
-0.292307692307692,-0.276923076923077,-0.261538461538462,-0.246153846153846,
-0.230769230769231,-0.215384615384615,-0.2,-0.184615384615385,-0.169230769230769,
-0.153846153846154,-0.138461538461538,-0.123076923076923,-0.107692307692308,
-0.0923076923076923,-0.0769230769230769,-0.0615384615384615,-0.0461538461538462,
-0.0307692307692308,-0.0153846153846154,0.),.UNSPECIFIED.)
CURVE()
GEOMETRIC_REPRESENTATION_ITEM()
RATIONAL_B_SPLINE_CURVE((1.,1.,1.,1.,1.,1.,1.,1.,1.,1.,1.,1.,1.,1.,1.,1.,
1.,1.,1.,1.,1.,1.,1.,1.,1.,1.,1.,1.,1.,1.,1.,1.,1.,1.,1.,1.,1.,1.,1.,1.,
1.,1.,1.,1.,1.,1.,1.,1.,1.,1.,1.,1.,1.,1.,1.,1.,1.,1.,1.,1.,1.,1.,1.,1.,
1.,1.,1.,1.,1.,1.))
REPRESENTATION_ITEM('')
);
#205=(
BOUNDED_CURVE()
B_SPLINE_CURVE(5,(#37217,#37218,#37219,#37220,#37221,#37222,#37223,#37224,
#37225,#37226,#37227,#37228,#37229,#37230,#37231,#37232,#37233,#37234,#37235,
#37236,#37237,#37238,#37239,#37240,#37241,#37242,#37243,#37244,#37245,#37246,
#37247,#37248,#37249,#37250,#37251,#37252,#37253,#37254,#37255,#37256,#37257,
#37258,#37259,#37260,#37261,#37262,#37263,#37264,#37265,#37266,#37267,#37268,
#37269,#37270,#37271,#37272,#37273,#37274,#37275,#37276,#37277,#37278,#37279,
#37280,#37281,#37282,#37283,#37284,#37285,#37286),.UNSPECIFIED.,.F.,.F.)
B_SPLINE_CURVE_WITH_KNOTS((6,1,1,1,1,1,1,1,1,1,1,1,1,1,1,1,1,1,1,1,1,1,
1,1,1,1,1,1,1,1,1,1,1,1,1,1,1,1,1,1,1,1,1,1,1,1,1,1,1,1,1,1,1,1,1,1,1,1,
1,1,1,1,1,1,1,6),(-1.,-0.984615384615383,-0.969230769230768,-0.953846153846152,
-0.938461538461537,-0.923076923076922,-0.907692307692306,-0.892307692307691,
-0.876923076923076,-0.86153846153846,-0.846153846153845,-0.83076923076923,
-0.815384615384614,-0.799999999999999,-0.784615384615384,-0.769230769230768,
-0.753846153846153,-0.738461538461538,-0.723076923076922,-0.707692307692307,
-0.692307692307692,-0.676923076923076,-0.661538461538461,-0.646153846153846,
-0.63076923076923,-0.615384615384615,-0.6,-0.584615384615384,-0.569230769230769,
-0.553846153846154,-0.538461538461538,-0.523076923076923,-0.507692307692308,
-0.492307692307692,-0.476923076923077,-0.461538461538462,-0.446153846153846,
-0.430769230769231,-0.415384615384615,-0.4,-0.384615384615385,-0.369230769230769,
-0.353846153846154,-0.338461538461538,-0.323076923076923,-0.307692307692308,
-0.292307692307692,-0.276923076923077,-0.261538461538462,-0.246153846153846,
-0.230769230769231,-0.215384615384615,-0.2,-0.184615384615385,-0.169230769230769,
-0.153846153846154,-0.138461538461538,-0.123076923076923,-0.107692307692308,
-0.0923076923076923,-0.0769230769230769,-0.0615384615384615,-0.0461538461538462,
-0.0307692307692308,-0.0153846153846154,0.),.UNSPECIFIED.)
CURVE()
GEOMETRIC_REPRESENTATION_ITEM()
RATIONAL_B_SPLINE_CURVE((1.,1.,1.,1.,1.,1.,1.,1.,1.,1.,1.,1.,1.,1.,1.,1.,
1.,1.,1.,1.,1.,1.,1.,1.,1.,1.,1.,1.,1.,1.,1.,1.,1.,1.,1.,1.,1.,1.,1.,1.,
1.,1.,1.,1.,1.,1.,1.,1.,1.,1.,1.,1.,1.,1.,1.,1.,1.,1.,1.,1.,1.,1.,1.,1.,
1.,1.,1.,1.,1.,1.))
REPRESENTATION_ITEM('')
);
#206=(
BOUNDED_CURVE()
B_SPLINE_CURVE(5,(#37433,#37434,#37435,#37436,#37437,#37438,#37439,#37440,
#37441,#37442,#37443,#37444,#37445,#37446,#37447,#37448,#37449,#37450,#37451,
#37452,#37453,#37454,#37455,#37456,#37457,#37458,#37459,#37460,#37461,#37462,
#37463,#37464,#37465,#37466,#37467,#37468,#37469,#37470,#37471,#37472,#37473,
#37474,#37475,#37476,#37477,#37478,#37479,#37480,#37481,#37482,#37483,#37484,
#37485,#37486,#37487,#37488,#37489,#37490,#37491,#37492,#37493,#37494,#37495,
#37496,#37497,#37498,#37499,#37500,#37501,#37502),.UNSPECIFIED.,.F.,.F.)
B_SPLINE_CURVE_WITH_KNOTS((6,1,1,1,1,1,1,1,1,1,1,1,1,1,1,1,1,1,1,1,1,1,
1,1,1,1,1,1,1,1,1,1,1,1,1,1,1,1,1,1,1,1,1,1,1,1,1,1,1,1,1,1,1,1,1,1,1,1,
1,1,1,1,1,1,1,6),(-1.,-0.984615384615383,-0.969230769230768,-0.953846153846152,
-0.938461538461537,-0.923076923076922,-0.907692307692306,-0.892307692307691,
-0.876923076923076,-0.86153846153846,-0.846153846153845,-0.83076923076923,
-0.815384615384614,-0.799999999999999,-0.784615384615384,-0.769230769230768,
-0.753846153846153,-0.738461538461538,-0.723076923076922,-0.707692307692307,
-0.692307692307692,-0.676923076923076,-0.661538461538461,-0.646153846153846,
-0.63076923076923,-0.615384615384615,-0.6,-0.584615384615384,-0.569230769230769,
-0.553846153846154,-0.538461538461538,-0.523076923076923,-0.507692307692308,
-0.492307692307692,-0.476923076923077,-0.461538461538462,-0.446153846153846,
-0.430769230769231,-0.415384615384615,-0.4,-0.384615384615385,-0.369230769230769,
-0.353846153846154,-0.338461538461538,-0.323076923076923,-0.307692307692308,
-0.292307692307692,-0.276923076923077,-0.261538461538462,-0.246153846153846,
-0.230769230769231,-0.215384615384615,-0.2,-0.184615384615385,-0.169230769230769,
-0.153846153846154,-0.138461538461538,-0.123076923076923,-0.107692307692308,
-0.0923076923076923,-0.0769230769230769,-0.0615384615384615,-0.0461538461538462,
-0.0307692307692308,-0.0153846153846154,0.),.UNSPECIFIED.)
CURVE()
GEOMETRIC_REPRESENTATION_ITEM()
RATIONAL_B_SPLINE_CURVE((1.,1.,1.,1.,1.,1.,1.,1.,1.,1.,1.,1.,1.,1.,1.,1.,
1.,1.,1.,1.,1.,1.,1.,1.,1.,1.,1.,1.,1.,1.,1.,1.,1.,1.,1.,1.,1.,1.,1.,1.,
1.,1.,1.,1.,1.,1.,1.,1.,1.,1.,1.,1.,1.,1.,1.,1.,1.,1.,1.,1.,1.,1.,1.,1.,
1.,1.,1.,1.,1.,1.))
REPRESENTATION_ITEM('')
);
#207=(
BOUNDED_CURVE()
B_SPLINE_CURVE(5,(#37649,#37650,#37651,#37652,#37653,#37654,#37655,#37656,
#37657,#37658,#37659,#37660,#37661,#37662,#37663,#37664,#37665,#37666,#37667,
#37668,#37669,#37670,#37671,#37672,#37673,#37674,#37675,#37676,#37677,#37678,
#37679,#37680,#37681,#37682,#37683,#37684,#37685,#37686,#37687,#37688,#37689,
#37690,#37691,#37692,#37693,#37694,#37695,#37696,#37697,#37698,#37699,#37700,
#37701,#37702,#37703,#37704,#37705,#37706,#37707,#37708,#37709,#37710,#37711,
#37712,#37713,#37714,#37715,#37716,#37717,#37718),.UNSPECIFIED.,.F.,.F.)
B_SPLINE_CURVE_WITH_KNOTS((6,1,1,1,1,1,1,1,1,1,1,1,1,1,1,1,1,1,1,1,1,1,
1,1,1,1,1,1,1,1,1,1,1,1,1,1,1,1,1,1,1,1,1,1,1,1,1,1,1,1,1,1,1,1,1,1,1,1,
1,1,1,1,1,1,1,6),(-1.,-0.984615384615383,-0.969230769230768,-0.953846153846152,
-0.938461538461537,-0.923076923076922,-0.907692307692306,-0.892307692307691,
-0.876923076923076,-0.86153846153846,-0.846153846153845,-0.83076923076923,
-0.815384615384614,-0.799999999999999,-0.784615384615384,-0.769230769230768,
-0.753846153846153,-0.738461538461538,-0.723076923076922,-0.707692307692307,
-0.692307692307692,-0.676923076923076,-0.661538461538461,-0.646153846153846,
-0.63076923076923,-0.615384615384615,-0.6,-0.584615384615384,-0.569230769230769,
-0.553846153846154,-0.538461538461538,-0.523076923076923,-0.507692307692308,
-0.492307692307692,-0.476923076923077,-0.461538461538462,-0.446153846153846,
-0.430769230769231,-0.415384615384615,-0.4,-0.384615384615385,-0.369230769230769,
-0.353846153846154,-0.338461538461538,-0.323076923076923,-0.307692307692308,
-0.292307692307692,-0.276923076923077,-0.261538461538462,-0.246153846153846,
-0.230769230769231,-0.215384615384615,-0.2,-0.184615384615385,-0.169230769230769,
-0.153846153846154,-0.138461538461538,-0.123076923076923,-0.107692307692308,
-0.0923076923076923,-0.0769230769230769,-0.0615384615384615,-0.0461538461538462,
-0.0307692307692308,-0.0153846153846154,0.),.UNSPECIFIED.)
CURVE()
GEOMETRIC_REPRESENTATION_ITEM()
RATIONAL_B_SPLINE_CURVE((1.,1.,1.,1.,1.,1.,1.,1.,1.,1.,1.,1.,1.,1.,1.,1.,
1.,1.,1.,1.,1.,1.,1.,1.,1.,1.,1.,1.,1.,1.,1.,1.,1.,1.,1.,1.,1.,1.,1.,1.,
1.,1.,1.,1.,1.,1.,1.,1.,1.,1.,1.,1.,1.,1.,1.,1.,1.,1.,1.,1.,1.,1.,1.,1.,
1.,1.,1.,1.,1.,1.))
REPRESENTATION_ITEM('')
);
#208=(
BOUNDED_CURVE()
B_SPLINE_CURVE(5,(#37865,#37866,#37867,#37868,#37869,#37870,#37871,#37872,
#37873,#37874,#37875,#37876,#37877,#37878,#37879,#37880,#37881,#37882,#37883,
#37884,#37885,#37886,#37887,#37888,#37889,#37890,#37891,#37892,#37893,#37894,
#37895,#37896,#37897,#37898,#37899,#37900,#37901,#37902,#37903,#37904,#37905,
#37906,#37907,#37908,#37909,#37910,#37911,#37912,#37913,#37914,#37915,#37916,
#37917,#37918,#37919,#37920,#37921,#37922,#37923,#37924,#37925,#37926,#37927,
#37928,#37929,#37930,#37931,#37932,#37933,#37934),.UNSPECIFIED.,.F.,.F.)
B_SPLINE_CURVE_WITH_KNOTS((6,1,1,1,1,1,1,1,1,1,1,1,1,1,1,1,1,1,1,1,1,1,
1,1,1,1,1,1,1,1,1,1,1,1,1,1,1,1,1,1,1,1,1,1,1,1,1,1,1,1,1,1,1,1,1,1,1,1,
1,1,1,1,1,1,1,6),(-1.,-0.984615384615383,-0.969230769230768,-0.953846153846152,
-0.938461538461537,-0.923076923076922,-0.907692307692306,-0.892307692307691,
-0.876923076923076,-0.86153846153846,-0.846153846153845,-0.83076923076923,
-0.815384615384614,-0.799999999999999,-0.784615384615384,-0.769230769230768,
-0.753846153846153,-0.738461538461538,-0.723076923076922,-0.707692307692307,
-0.692307692307692,-0.676923076923076,-0.661538461538461,-0.646153846153846,
-0.63076923076923,-0.615384615384615,-0.6,-0.584615384615384,-0.569230769230769,
-0.553846153846154,-0.538461538461538,-0.523076923076923,-0.507692307692308,
-0.492307692307692,-0.476923076923077,-0.461538461538462,-0.446153846153846,
-0.430769230769231,-0.415384615384615,-0.4,-0.384615384615385,-0.369230769230769,
-0.353846153846154,-0.338461538461538,-0.323076923076923,-0.307692307692308,
-0.292307692307692,-0.276923076923077,-0.261538461538462,-0.246153846153846,
-0.230769230769231,-0.215384615384615,-0.2,-0.184615384615385,-0.169230769230769,
-0.153846153846154,-0.138461538461538,-0.123076923076923,-0.107692307692308,
-0.0923076923076923,-0.0769230769230769,-0.0615384615384615,-0.0461538461538462,
-0.0307692307692308,-0.0153846153846154,0.),.UNSPECIFIED.)
CURVE()
GEOMETRIC_REPRESENTATION_ITEM()
RATIONAL_B_SPLINE_CURVE((1.,1.,1.,1.,1.,1.,1.,1.,1.,1.,1.,1.,1.,1.,1.,1.,
1.,1.,1.,1.,1.,1.,1.,1.,1.,1.,1.,1.,1.,1.,1.,1.,1.,1.,1.,1.,1.,1.,1.,1.,
1.,1.,1.,1.,1.,1.,1.,1.,1.,1.,1.,1.,1.,1.,1.,1.,1.,1.,1.,1.,1.,1.,1.,1.,
1.,1.,1.,1.,1.,1.))
REPRESENTATION_ITEM('')
);
#209=(
BOUNDED_CURVE()
B_SPLINE_CURVE(5,(#38081,#38082,#38083,#38084,#38085,#38086,#38087,#38088,
#38089,#38090,#38091,#38092,#38093,#38094,#38095,#38096,#38097,#38098,#38099,
#38100,#38101,#38102,#38103,#38104,#38105,#38106,#38107,#38108,#38109,#38110,
#38111,#38112,#38113,#38114,#38115,#38116,#38117,#38118,#38119,#38120,#38121,
#38122,#38123,#38124,#38125,#38126,#38127,#38128,#38129,#38130,#38131,#38132,
#38133,#38134,#38135,#38136,#38137,#38138,#38139,#38140,#38141,#38142,#38143,
#38144,#38145,#38146,#38147,#38148,#38149,#38150),.UNSPECIFIED.,.F.,.F.)
B_SPLINE_CURVE_WITH_KNOTS((6,1,1,1,1,1,1,1,1,1,1,1,1,1,1,1,1,1,1,1,1,1,
1,1,1,1,1,1,1,1,1,1,1,1,1,1,1,1,1,1,1,1,1,1,1,1,1,1,1,1,1,1,1,1,1,1,1,1,
1,1,1,1,1,1,1,6),(-1.,-0.984615384615383,-0.969230769230768,-0.953846153846152,
-0.938461538461537,-0.923076923076922,-0.907692307692306,-0.892307692307691,
-0.876923076923076,-0.86153846153846,-0.846153846153845,-0.83076923076923,
-0.815384615384614,-0.799999999999999,-0.784615384615384,-0.769230769230768,
-0.753846153846153,-0.738461538461538,-0.723076923076922,-0.707692307692307,
-0.692307692307692,-0.676923076923076,-0.661538461538461,-0.646153846153846,
-0.63076923076923,-0.615384615384615,-0.6,-0.584615384615384,-0.569230769230769,
-0.553846153846154,-0.538461538461538,-0.523076923076923,-0.507692307692308,
-0.492307692307692,-0.476923076923077,-0.461538461538462,-0.446153846153846,
-0.430769230769231,-0.415384615384615,-0.4,-0.384615384615385,-0.369230769230769,
-0.353846153846154,-0.338461538461538,-0.323076923076923,-0.307692307692308,
-0.292307692307692,-0.276923076923077,-0.261538461538462,-0.246153846153846,
-0.230769230769231,-0.215384615384615,-0.2,-0.184615384615385,-0.169230769230769,
-0.153846153846154,-0.138461538461538,-0.123076923076923,-0.107692307692308,
-0.0923076923076923,-0.0769230769230769,-0.0615384615384615,-0.0461538461538462,
-0.0307692307692308,-0.0153846153846154,0.),.UNSPECIFIED.)
CURVE()
GEOMETRIC_REPRESENTATION_ITEM()
RATIONAL_B_SPLINE_CURVE((1.,1.,1.,1.,1.,1.,1.,1.,1.,1.,1.,1.,1.,1.,1.,1.,
1.,1.,1.,1.,1.,1.,1.,1.,1.,1.,1.,1.,1.,1.,1.,1.,1.,1.,1.,1.,1.,1.,1.,1.,
1.,1.,1.,1.,1.,1.,1.,1.,1.,1.,1.,1.,1.,1.,1.,1.,1.,1.,1.,1.,1.,1.,1.,1.,
1.,1.,1.,1.,1.,1.))
REPRESENTATION_ITEM('')
);
#210=(
BOUNDED_CURVE()
B_SPLINE_CURVE(5,(#38297,#38298,#38299,#38300,#38301,#38302,#38303,#38304,
#38305,#38306,#38307,#38308,#38309,#38310,#38311,#38312,#38313,#38314,#38315,
#38316,#38317,#38318,#38319,#38320,#38321,#38322,#38323,#38324,#38325,#38326,
#38327,#38328,#38329,#38330,#38331,#38332,#38333,#38334,#38335,#38336,#38337,
#38338,#38339,#38340,#38341,#38342,#38343,#38344,#38345,#38346,#38347,#38348,
#38349,#38350,#38351,#38352,#38353,#38354,#38355,#38356,#38357,#38358,#38359,
#38360,#38361,#38362,#38363,#38364,#38365,#38366),.UNSPECIFIED.,.F.,.F.)
B_SPLINE_CURVE_WITH_KNOTS((6,1,1,1,1,1,1,1,1,1,1,1,1,1,1,1,1,1,1,1,1,1,
1,1,1,1,1,1,1,1,1,1,1,1,1,1,1,1,1,1,1,1,1,1,1,1,1,1,1,1,1,1,1,1,1,1,1,1,
1,1,1,1,1,1,1,6),(-1.,-0.984615384615383,-0.969230769230768,-0.953846153846152,
-0.938461538461537,-0.923076923076922,-0.907692307692306,-0.892307692307691,
-0.876923076923076,-0.86153846153846,-0.846153846153845,-0.83076923076923,
-0.815384615384614,-0.799999999999999,-0.784615384615384,-0.769230769230768,
-0.753846153846153,-0.738461538461538,-0.723076923076922,-0.707692307692307,
-0.692307692307692,-0.676923076923076,-0.661538461538461,-0.646153846153846,
-0.63076923076923,-0.615384615384615,-0.6,-0.584615384615384,-0.569230769230769,
-0.553846153846154,-0.538461538461538,-0.523076923076923,-0.507692307692308,
-0.492307692307692,-0.476923076923077,-0.461538461538462,-0.446153846153846,
-0.430769230769231,-0.415384615384615,-0.4,-0.384615384615385,-0.369230769230769,
-0.353846153846154,-0.338461538461538,-0.323076923076923,-0.307692307692308,
-0.292307692307692,-0.276923076923077,-0.261538461538462,-0.246153846153846,
-0.230769230769231,-0.215384615384615,-0.2,-0.184615384615385,-0.169230769230769,
-0.153846153846154,-0.138461538461538,-0.123076923076923,-0.107692307692308,
-0.0923076923076923,-0.0769230769230769,-0.0615384615384615,-0.0461538461538462,
-0.0307692307692308,-0.0153846153846154,0.),.UNSPECIFIED.)
CURVE()
GEOMETRIC_REPRESENTATION_ITEM()
RATIONAL_B_SPLINE_CURVE((1.,1.,1.,1.,1.,1.,1.,1.,1.,1.,1.,1.,1.,1.,1.,1.,
1.,1.,1.,1.,1.,1.,1.,1.,1.,1.,1.,1.,1.,1.,1.,1.,1.,1.,1.,1.,1.,1.,1.,1.,
1.,1.,1.,1.,1.,1.,1.,1.,1.,1.,1.,1.,1.,1.,1.,1.,1.,1.,1.,1.,1.,1.,1.,1.,
1.,1.,1.,1.,1.,1.))
REPRESENTATION_ITEM('')
);
#1110=SHAPE_REPRESENTATION_RELATIONSHIP('SRR','None',#63087,#1174);
#1174=ADVANCED_BREP_SHAPE_REPRESENTATION('',(#1328),#62741);
#1253=STYLED_ITEM('',(#63476),#1328);
#1328=MANIFOLD_SOLID_BREP('Body1',#16437);
#1600=FACE_BOUND('',#3896,.T.);
#1601=FACE_BOUND('',#3900,.T.);
#1602=FACE_BOUND('',#3981,.T.);
#1977=PLANE('',#18272);
#1978=PLANE('',#18273);
#1979=PLANE('',#18274);
#1980=PLANE('',#18275);
#1981=PLANE('',#18302);
#1982=PLANE('',#18303);
#1983=PLANE('',#18306);
#1984=PLANE('',#18309);
#1985=PLANE('',#18312);
#1986=PLANE('',#18315);
#1987=PLANE('',#18318);
#1988=PLANE('',#18321);
#1989=PLANE('',#18324);
#1990=PLANE('',#18327);
#1991=PLANE('',#18330);
#1992=PLANE('',#18333);
#1993=PLANE('',#18336);
#1994=PLANE('',#18339);
#1995=PLANE('',#18342);
#1996=PLANE('',#18345);
#1997=PLANE('',#18348);
#1998=PLANE('',#18351);
#1999=PLANE('',#18354);
#2000=PLANE('',#18357);
#2001=PLANE('',#18360);
#2002=PLANE('',#18361);
#2698=FACE_OUTER_BOUND('',#3892,.T.);
#2699=FACE_OUTER_BOUND('',#3893,.T.);
#2700=FACE_OUTER_BOUND('',#3894,.T.);
#2701=FACE_OUTER_BOUND('',#3895,.T.);
#2702=FACE_OUTER_BOUND('',#3897,.T.);
#2703=FACE_OUTER_BOUND('',#3898,.T.);
#2704=FACE_OUTER_BOUND('',#3899,.T.);
#2705=FACE_OUTER_BOUND('',#3901,.T.);
#2706=FACE_OUTER_BOUND('',#3902,.T.);
#2707=FACE_OUTER_BOUND('',#3903,.T.);
#2708=FACE_OUTER_BOUND('',#3904,.T.);
#2709=FACE_OUTER_BOUND('',#3905,.T.);
#2710=FACE_OUTER_BOUND('',#3906,.T.);
#2711=FACE_OUTER_BOUND('',#3907,.T.);
#2712=FACE_OUTER_BOUND('',#3908,.T.);
#2713=FACE_OUTER_BOUND('',#3909,.T.);
#2714=FACE_OUTER_BOUND('',#3910,.T.);
#2715=FACE_OUTER_BOUND('',#3911,.T.);
#2716=FACE_OUTER_BOUND('',#3912,.T.);
#2717=FACE_OUTER_BOUND('',#3913,.T.);
#2718=FACE_OUTER_BOUND('',#3914,.T.);
#2719=FACE_OUTER_BOUND('',#3915,.T.);
#2720=FACE_OUTER_BOUND('',#3916,.T.);
#2721=FACE_OUTER_BOUND('',#3917,.T.);
#2722=FACE_OUTER_BOUND('',#3918,.T.);
#2723=FACE_OUTER_BOUND('',#3919,.T.);
#2724=FACE_OUTER_BOUND('',#3920,.T.);
#2725=FACE_OUTER_BOUND('',#3921,.T.);
#2726=FACE_OUTER_BOUND('',#3922,.T.);
#2727=FACE_OUTER_BOUND('',#3923,.T.);
#2728=FACE_OUTER_BOUND('',#3924,.T.);
#2729=FACE_OUTER_BOUND('',#3925,.T.);
#2730=FACE_OUTER_BOUND('',#3926,.T.);
#2731=FACE_OUTER_BOUND('',#3927,.T.);
#2732=FACE_OUTER_BOUND('',#3928,.T.);
#2733=FACE_OUTER_BOUND('',#3929,.T.);
#2734=FACE_OUTER_BOUND('',#3930,.T.);
#2735=FACE_OUTER_BOUND('',#3931,.T.);
#2736=FACE_OUTER_BOUND('',#3932,.T.);
#2737=FACE_OUTER_BOUND('',#3933,.T.);
#2738=FACE_OUTER_BOUND('',#3934,.T.);
#2739=FACE_OUTER_BOUND('',#3935,.T.);
#2740=FACE_OUTER_BOUND('',#3936,.T.);
#2741=FACE_OUTER_BOUND('',#3937,.T.);
#2742=FACE_OUTER_BOUND('',#3938,.T.);
#2743=FACE_OUTER_BOUND('',#3939,.T.);
#2744=FACE_OUTER_BOUND('',#3940,.T.);
#2745=FACE_OUTER_BOUND('',#3941,.T.);
#2746=FACE_OUTER_BOUND('',#3942,.T.);
#2747=FACE_OUTER_BOUND('',#3943,.T.);
#2748=FACE_OUTER_BOUND('',#3944,.T.);
#2749=FACE_OUTER_BOUND('',#3945,.T.);
#2750=FACE_OUTER_BOUND('',#3946,.T.);
#2751=FACE_OUTER_BOUND('',#3947,.T.);
#2752=FACE_OUTER_BOUND('',#3948,.T.);
#2753=FACE_OUTER_BOUND('',#3949,.T.);
#2754=FACE_OUTER_BOUND('',#3950,.T.);
#2755=FACE_OUTER_BOUND('',#3951,.T.);
#2756=FACE_OUTER_BOUND('',#3952,.T.);
#2757=FACE_OUTER_BOUND('',#3953,.T.);
#2758=FACE_OUTER_BOUND('',#3954,.T.);
#2759=FACE_OUTER_BOUND('',#3955,.T.);
#2760=FACE_OUTER_BOUND('',#3956,.T.);
#2761=FACE_OUTER_BOUND('',#3957,.T.);
#2762=FACE_OUTER_BOUND('',#3958,.T.);
#2763=FACE_OUTER_BOUND('',#3959,.T.);
#2764=FACE_OUTER_BOUND('',#3960,.T.);
#2765=FACE_OUTER_BOUND('',#3961,.T.);
#2766=FACE_OUTER_BOUND('',#3962,.T.);
#2767=FACE_OUTER_BOUND('',#3963,.T.);
#2768=FACE_OUTER_BOUND('',#3964,.T.);
#2769=FACE_OUTER_BOUND('',#3965,.T.);
#2770=FACE_OUTER_BOUND('',#3966,.T.);
#2771=FACE_OUTER_BOUND('',#3967,.T.);
#2772=FACE_OUTER_BOUND('',#3968,.T.);
#2773=FACE_OUTER_BOUND('',#3969,.T.);
#2774=FACE_OUTER_BOUND('',#3970,.T.);
#2775=FACE_OUTER_BOUND('',#3971,.T.);
#2776=FACE_OUTER_BOUND('',#3972,.T.);
#2777=FACE_OUTER_BOUND('',#3973,.T.);
#2778=FACE_OUTER_BOUND('',#3974,.T.);
#2779=FACE_OUTER_BOUND('',#3975,.T.);
#2780=FACE_OUTER_BOUND('',#3976,.T.);
#2781=FACE_OUTER_BOUND('',#3977,.T.);
#2782=FACE_OUTER_BOUND('',#3978,.T.);
#2783=FACE_OUTER_BOUND('',#3979,.T.);
#2784=FACE_OUTER_BOUND('',#3980,.T.);
#2785=FACE_OUTER_BOUND('',#3982,.T.);
#3892=EDGE_LOOP('',(#13255,#13256,#13257,#13258));
#3893=EDGE_LOOP('',(#13259,#13260,#13261,#13262));
#3894=EDGE_LOOP('',(#13263,#13264,#13265,#13266));
#3895=EDGE_LOOP('',(#13267,#13268,#13269,#13270,#13271,#13272,#13273,#13274,
#13275,#13276,#13277,#13278,#13279,#13280,#13281,#13282,#13283,#13284,#13285,
#13286,#13287,#13288,#13289,#13290,#13291,#13292,#13293,#13294,#13295,#13296,
#13297,#13298,#13299,#13300,#13301,#13302,#13303,#13304,#13305,#13306,#13307,
#13308,#13309,#13310,#13311,#13312,#13313,#13314,#13315,#13316,#13317,#13318,
#13319,#13320,#13321,#13322,#13323,#13324,#13325,#13326,#13327,#13328,#13329,
#13330,#13331,#13332,#13333,#13334,#13335,#13336,#13337,#13338,#13339,#13340,
#13341,#13342,#13343,#13344,#13345,#13346));
#3896=EDGE_LOOP('',(#13347,#13348,#13349,#13350));
#3897=EDGE_LOOP('',(#13351,#13352,#13353,#13354));
#3898=EDGE_LOOP('',(#13355,#13356,#13357,#13358));
#3899=EDGE_LOOP('',(#13359));
#3900=EDGE_LOOP('',(#13360,#13361,#13362,#13363));
#3901=EDGE_LOOP('',(#13364,#13365,#13366,#13367));
#3902=EDGE_LOOP('',(#13368,#13369,#13370,#13371));
#3903=EDGE_LOOP('',(#13372,#13373,#13374,#13375));
#3904=EDGE_LOOP('',(#13376,#13377,#13378,#13379));
#3905=EDGE_LOOP('',(#13380,#13381,#13382,#13383));
#3906=EDGE_LOOP('',(#13384,#13385,#13386,#13387));
#3907=EDGE_LOOP('',(#13388,#13389,#13390,#13391));
#3908=EDGE_LOOP('',(#13392,#13393,#13394,#13395));
#3909=EDGE_LOOP('',(#13396,#13397,#13398,#13399));
#3910=EDGE_LOOP('',(#13400,#13401,#13402,#13403));
#3911=EDGE_LOOP('',(#13404,#13405,#13406,#13407));
#3912=EDGE_LOOP('',(#13408,#13409,#13410,#13411));
#3913=EDGE_LOOP('',(#13412,#13413,#13414,#13415));
#3914=EDGE_LOOP('',(#13416,#13417,#13418,#13419));
#3915=EDGE_LOOP('',(#13420,#13421,#13422,#13423));
#3916=EDGE_LOOP('',(#13424,#13425,#13426,#13427));
#3917=EDGE_LOOP('',(#13428,#13429,#13430,#13431));
#3918=EDGE_LOOP('',(#13432,#13433,#13434,#13435));
#3919=EDGE_LOOP('',(#13436,#13437,#13438,#13439));
#3920=EDGE_LOOP('',(#13440,#13441,#13442,#13443));
#3921=EDGE_LOOP('',(#13444,#13445,#13446,#13447));
#3922=EDGE_LOOP('',(#13448,#13449,#13450,#13451));
#3923=EDGE_LOOP('',(#13452,#13453,#13454,#13455));
#3924=EDGE_LOOP('',(#13456,#13457,#13458,#13459));
#3925=EDGE_LOOP('',(#13460,#13461,#13462,#13463));
#3926=EDGE_LOOP('',(#13464,#13465,#13466,#13467));
#3927=EDGE_LOOP('',(#13468,#13469,#13470,#13471));
#3928=EDGE_LOOP('',(#13472,#13473,#13474,#13475));
#3929=EDGE_LOOP('',(#13476,#13477,#13478,#13479));
#3930=EDGE_LOOP('',(#13480,#13481,#13482,#13483));
#3931=EDGE_LOOP('',(#13484,#13485,#13486,#13487));
#3932=EDGE_LOOP('',(#13488,#13489,#13490,#13491));
#3933=EDGE_LOOP('',(#13492,#13493,#13494,#13495));
#3934=EDGE_LOOP('',(#13496,#13497,#13498,#13499));
#3935=EDGE_LOOP('',(#13500,#13501,#13502,#13503));
#3936=EDGE_LOOP('',(#13504,#13505,#13506,#13507));
#3937=EDGE_LOOP('',(#13508,#13509,#13510,#13511));
#3938=EDGE_LOOP('',(#13512,#13513,#13514,#13515));
#3939=EDGE_LOOP('',(#13516,#13517,#13518,#13519));
#3940=EDGE_LOOP('',(#13520,#13521,#13522,#13523));
#3941=EDGE_LOOP('',(#13524,#13525,#13526,#13527));
#3942=EDGE_LOOP('',(#13528,#13529,#13530,#13531));
#3943=EDGE_LOOP('',(#13532,#13533,#13534,#13535));
#3944=EDGE_LOOP('',(#13536,#13537,#13538,#13539));
#3945=EDGE_LOOP('',(#13540,#13541,#13542,#13543));
#3946=EDGE_LOOP('',(#13544,#13545,#13546,#13547));
#3947=EDGE_LOOP('',(#13548,#13549,#13550,#13551));
#3948=EDGE_LOOP('',(#13552,#13553,#13554,#13555));
#3949=EDGE_LOOP('',(#13556,#13557,#13558,#13559));
#3950=EDGE_LOOP('',(#13560,#13561,#13562,#13563));
#3951=EDGE_LOOP('',(#13564,#13565,#13566,#13567));
#3952=EDGE_LOOP('',(#13568,#13569,#13570,#13571));
#3953=EDGE_LOOP('',(#13572,#13573,#13574,#13575));
#3954=EDGE_LOOP('',(#13576,#13577,#13578,#13579));
#3955=EDGE_LOOP('',(#13580,#13581,#13582,#13583));
#3956=EDGE_LOOP('',(#13584,#13585,#13586,#13587));
#3957=EDGE_LOOP('',(#13588,#13589,#13590,#13591));
#3958=EDGE_LOOP('',(#13592,#13593,#13594,#13595));
#3959=EDGE_LOOP('',(#13596,#13597,#13598,#13599));
#3960=EDGE_LOOP('',(#13600,#13601,#13602,#13603));
#3961=EDGE_LOOP('',(#13604,#13605,#13606,#13607));
#3962=EDGE_LOOP('',(#13608,#13609,#13610,#13611));
#3963=EDGE_LOOP('',(#13612,#13613,#13614,#13615));
#3964=EDGE_LOOP('',(#13616,#13617,#13618,#13619));
#3965=EDGE_LOOP('',(#13620,#13621,#13622,#13623));
#3966=EDGE_LOOP('',(#13624,#13625,#13626,#13627));
#3967=EDGE_LOOP('',(#13628,#13629,#13630,#13631));
#3968=EDGE_LOOP('',(#13632,#13633,#13634,#13635));
#3969=EDGE_LOOP('',(#13636,#13637,#13638,#13639));
#3970=EDGE_LOOP('',(#13640,#13641,#13642,#13643));
#3971=EDGE_LOOP('',(#13644,#13645,#13646,#13647));
#3972=EDGE_LOOP('',(#13648,#13649,#13650,#13651));
#3973=EDGE_LOOP('',(#13652,#13653,#13654,#13655));
#3974=EDGE_LOOP('',(#13656,#13657,#13658,#13659));
#3975=EDGE_LOOP('',(#13660,#13661,#13662,#13663));
#3976=EDGE_LOOP('',(#13664,#13665,#13666,#13667));
#3977=EDGE_LOOP('',(#13668,#13669,#13670,#13671));
#3978=EDGE_LOOP('',(#13672,#13673,#13674,#13675));
#3979=EDGE_LOOP('',(#13676,#13677,#13678,#13679));
#3980=EDGE_LOOP('',(#13680,#13681,#13682,#13683,#13684,#13685,#13686,#13687,
#13688,#13689,#13690,#13691,#13692,#13693,#13694,#13695,#13696,#13697,#13698,
#13699,#13700,#13701,#13702,#13703,#13704,#13705,#13706,#13707,#13708,#13709,
#13710,#13711,#13712,#13713,#13714,#13715,#13716,#13717,#13718,#13719,#13720,
#13721,#13722,#13723,#13724,#13725,#13726,#13727,#13728,#13729,#13730,#13731,
#13732,#13733,#13734,#13735,#13736,#13737,#13738,#13739,#13740,#13741,#13742,
#13743,#13744,#13745,#13746,#13747,#13748,#13749,#13750,#13751,#13752,#13753,
#13754,#13755,#13756,#13757,#13758,#13759));
#3981=EDGE_LOOP('',(#13760));
#3982=EDGE_LOOP('',(#13761,#13762,#13763,#13764));
#4980=LINE('',#26781,#6112);
#4981=LINE('',#26783,#6113);
#4982=LINE('',#26785,#6114);
#4983=LINE('',#26786,#6115);
#4984=LINE('',#26789,#6116);
#4985=LINE('',#26791,#6117);
#4986=LINE('',#26792,#6118);
#4987=LINE('',#26795,#6119);
#4988=LINE('',#26797,#6120);
#4989=LINE('',#26798,#6121);
#4990=LINE('',#26875,#6122);
#4991=LINE('',#27021,#6123);
#4992=LINE('',#27167,#6124);
#4993=LINE('',#27313,#6125);
#4994=LINE('',#27459,#6126);
#4995=LINE('',#27605,#6127);
#4996=LINE('',#27751,#6128);
#4997=LINE('',#27897,#6129);
#4998=LINE('',#28043,#6130);
#4999=LINE('',#28189,#6131);
#5000=LINE('',#28335,#6132);
#5001=LINE('',#28481,#6133);
#5002=LINE('',#28627,#6134);
#5003=LINE('',#28773,#6135);
#5004=LINE('',#28919,#6136);
#5005=LINE('',#29065,#6137);
#5006=LINE('',#29211,#6138);
#5007=LINE('',#29357,#6139);
#5008=LINE('',#29503,#6140);
#5009=LINE('',#29649,#6141);
#5010=LINE('',#29727,#6142);
#5011=LINE('',#29871,#6143);
#5012=LINE('',#29943,#6144);
#5013=LINE('',#29946,#6145);
#5014=LINE('',#29947,#6146);
#5015=LINE('',#30159,#6147);
#5016=LINE('',#30163,#6148);
#5017=LINE('',#30375,#6149);
#5018=LINE('',#30378,#6150);
#5019=LINE('',#30379,#6151);
#5020=LINE('',#30591,#6152);
#5021=LINE('',#30595,#6153);
#5022=LINE('',#30807,#6154);
#5023=LINE('',#30810,#6155);
#5024=LINE('',#30811,#6156);
#5025=LINE('',#31023,#6157);
#5026=LINE('',#31027,#6158);
#5027=LINE('',#31239,#6159);
#5028=LINE('',#31242,#6160);
#5029=LINE('',#31243,#6161);
#5030=LINE('',#31455,#6162);
#5031=LINE('',#31459,#6163);
#5032=LINE('',#31671,#6164);
#5033=LINE('',#31674,#6165);
#5034=LINE('',#31675,#6166);
#5035=LINE('',#31887,#6167);
#5036=LINE('',#31891,#6168);
#5037=LINE('',#32103,#6169);
#5038=LINE('',#32106,#6170);
#5039=LINE('',#32107,#6171);
#5040=LINE('',#32319,#6172);
#5041=LINE('',#32323,#6173);
#5042=LINE('',#32535,#6174);
#5043=LINE('',#32538,#6175);
#5044=LINE('',#32539,#6176);
#5045=LINE('',#32751,#6177);
#5046=LINE('',#32755,#6178);
#5047=LINE('',#32967,#6179);
#5048=LINE('',#32970,#6180);
#5049=LINE('',#32971,#6181);
#5050=LINE('',#33183,#6182);
#5051=LINE('',#33187,#6183);
#5052=LINE('',#33399,#6184);
#5053=LINE('',#33402,#6185);
#5054=LINE('',#33403,#6186);
#5055=LINE('',#33615,#6187);
#5056=LINE('',#33619,#6188);
#5057=LINE('',#33831,#6189);
#5058=LINE('',#33834,#6190);
#5059=LINE('',#33835,#6191);
#5060=LINE('',#34047,#6192);
#5061=LINE('',#34051,#6193);
#5062=LINE('',#34263,#6194);
#5063=LINE('',#34266,#6195);
#5064=LINE('',#34267,#6196);
#5065=LINE('',#34479,#6197);
#5066=LINE('',#34483,#6198);
#5067=LINE('',#34695,#6199);
#5068=LINE('',#34698,#6200);
#5069=LINE('',#34699,#6201);
#5070=LINE('',#34911,#6202);
#5071=LINE('',#34915,#6203);
#5072=LINE('',#35127,#6204);
#5073=LINE('',#35130,#6205);
#5074=LINE('',#35131,#6206);
#5075=LINE('',#35343,#6207);
#5076=LINE('',#35347,#6208);
#5077=LINE('',#35559,#6209);
#5078=LINE('',#35562,#6210);
#5079=LINE('',#35563,#6211);
#5080=LINE('',#35775,#6212);
#5081=LINE('',#35779,#6213);
#5082=LINE('',#35991,#6214);
#5083=LINE('',#35994,#6215);
#5084=LINE('',#35995,#6216);
#5085=LINE('',#36207,#6217);
#5086=LINE('',#36211,#6218);
#5087=LINE('',#36423,#6219);
#5088=LINE('',#36426,#6220);
#5089=LINE('',#36427,#6221);
#5090=LINE('',#36639,#6222);
#5091=LINE('',#36643,#6223);
#5092=LINE('',#36855,#6224);
#5093=LINE('',#36858,#6225);
#5094=LINE('',#36859,#6226);
#5095=LINE('',#37071,#6227);
#5096=LINE('',#37075,#6228);
#5097=LINE('',#37287,#6229);
#5098=LINE('',#37290,#6230);
#5099=LINE('',#37291,#6231);
#5100=LINE('',#37503,#6232);
#5101=LINE('',#37507,#6233);
#5102=LINE('',#37719,#6234);
#5103=LINE('',#37722,#6235);
#5104=LINE('',#37723,#6236);
#5105=LINE('',#37935,#6237);
#5106=LINE('',#37939,#6238);
#5107=LINE('',#38151,#6239);
#5108=LINE('',#38154,#6240);
#5109=LINE('',#38155,#6241);
#5110=LINE('',#38367,#6242);
#6112=VECTOR('',#21755,1.);
#6113=VECTOR('',#21756,1.);
#6114=VECTOR('',#21757,1.);
#6115=VECTOR('',#21758,1.);
#6116=VECTOR('',#21761,1.);
#6117=VECTOR('',#21762,1.);
#6118=VECTOR('',#21763,1.);
#6119=VECTOR('',#21766,1.);
#6120=VECTOR('',#21767,1.);
#6121=VECTOR('',#21768,1.);
#6122=VECTOR('',#21773,1.);
#6123=VECTOR('',#21776,1.);
#6124=VECTOR('',#21779,1.);
#6125=VECTOR('',#21782,1.);
#6126=VECTOR('',#21785,1.);
#6127=VECTOR('',#21788,1.);
#6128=VECTOR('',#21791,1.);
#6129=VECTOR('',#21794,1.);
#6130=VECTOR('',#21797,1.);
#6131=VECTOR('',#21800,1.);
#6132=VECTOR('',#21803,1.);
#6133=VECTOR('',#21806,1.);
#6134=VECTOR('',#21809,1.);
#6135=VECTOR('',#21812,1.);
#6136=VECTOR('',#21815,1.);
#6137=VECTOR('',#21818,1.);
#6138=VECTOR('',#21821,1.);
#6139=VECTOR('',#21824,1.);
#6140=VECTOR('',#21827,1.);
#6141=VECTOR('',#21830,1.);
#6142=VECTOR('',#21841,1.4);
#6143=VECTOR('',#21846,1.);
#6144=VECTOR('',#21847,1.);
#6145=VECTOR('',#21850,1.);
#6146=VECTOR('',#21851,1.);
#6147=VECTOR('',#21852,1.);
#6148=VECTOR('',#21857,1.);
#6149=VECTOR('',#21858,1.);
#6150=VECTOR('',#21861,1.);
#6151=VECTOR('',#21862,1.);
#6152=VECTOR('',#21863,1.);
#6153=VECTOR('',#21868,1.);
#6154=VECTOR('',#21869,1.);
#6155=VECTOR('',#21872,1.);
#6156=VECTOR('',#21873,1.);
#6157=VECTOR('',#21874,1.);
#6158=VECTOR('',#21879,1.);
#6159=VECTOR('',#21880,1.);
#6160=VECTOR('',#21883,1.);
#6161=VECTOR('',#21884,1.);
#6162=VECTOR('',#21885,1.);
#6163=VECTOR('',#21890,1.);
#6164=VECTOR('',#21891,1.);
#6165=VECTOR('',#21894,1.);
#6166=VECTOR('',#21895,1.);
#6167=VECTOR('',#21896,1.);
#6168=VECTOR('',#21901,1.);
#6169=VECTOR('',#21902,1.);
#6170=VECTOR('',#21905,1.);
#6171=VECTOR('',#21906,1.);
#6172=VECTOR('',#21907,1.);
#6173=VECTOR('',#21912,1.);
#6174=VECTOR('',#21913,1.);
#6175=VECTOR('',#21916,1.);
#6176=VECTOR('',#21917,1.);
#6177=VECTOR('',#21918,1.);
#6178=VECTOR('',#21923,1.);
#6179=VECTOR('',#21924,1.);
#6180=VECTOR('',#21927,1.);
#6181=VECTOR('',#21928,1.);
#6182=VECTOR('',#21929,1.);
#6183=VECTOR('',#21934,1.);
#6184=VECTOR('',#21935,1.);
#6185=VECTOR('',#21938,1.);
#6186=VECTOR('',#21939,1.);
#6187=VECTOR('',#21940,1.);
#6188=VECTOR('',#21945,1.);
#6189=VECTOR('',#21946,1.);
#6190=VECTOR('',#21949,1.);
#6191=VECTOR('',#21950,1.);
#6192=VECTOR('',#21951,1.);
#6193=VECTOR('',#21956,1.);
#6194=VECTOR('',#21957,1.);
#6195=VECTOR('',#21960,1.);
#6196=VECTOR('',#21961,1.);
#6197=VECTOR('',#21962,1.);
#6198=VECTOR('',#21967,1.);
#6199=VECTOR('',#21968,1.);
#6200=VECTOR('',#21971,1.);
#6201=VECTOR('',#21972,1.);
#6202=VECTOR('',#21973,1.);
#6203=VECTOR('',#21978,1.);
#6204=VECTOR('',#21979,1.);
#6205=VECTOR('',#21982,1.);
#6206=VECTOR('',#21983,1.);
#6207=VECTOR('',#21984,1.);
#6208=VECTOR('',#21989,1.);
#6209=VECTOR('',#21990,1.);
#6210=VECTOR('',#21993,1.);
#6211=VECTOR('',#21994,1.);
#6212=VECTOR('',#21995,1.);
#6213=VECTOR('',#22000,1.);
#6214=VECTOR('',#22001,1.);
#6215=VECTOR('',#22004,1.);
#6216=VECTOR('',#22005,1.);
#6217=VECTOR('',#22006,1.);
#6218=VECTOR('',#22011,1.);
#6219=VECTOR('',#22012,1.);
#6220=VECTOR('',#22015,1.);
#6221=VECTOR('',#22016,1.);
#6222=VECTOR('',#22017,1.);
#6223=VECTOR('',#22022,1.);
#6224=VECTOR('',#22023,1.);
#6225=VECTOR('',#22026,1.);
#6226=VECTOR('',#22027,1.);
#6227=VECTOR('',#22028,1.);
#6228=VECTOR('',#22033,1.);
#6229=VECTOR('',#22034,1.);
#6230=VECTOR('',#22037,1.);
#6231=VECTOR('',#22038,1.);
#6232=VECTOR('',#22039,1.);
#6233=VECTOR('',#22044,1.);
#6234=VECTOR('',#22045,1.);
#6235=VECTOR('',#22048,1.);
#6236=VECTOR('',#22049,1.);
#6237=VECTOR('',#22050,1.);
#6238=VECTOR('',#22055,1.);
#6239=VECTOR('',#22056,1.);
#6240=VECTOR('',#22059,1.);
#6241=VECTOR('',#22060,1.);
#6242=VECTOR('',#22061,1.);
#7022=CIRCLE('',#18276,1.75);
#7023=CIRCLE('',#18277,1.75);
#7024=CIRCLE('',#18278,1.75);
#7025=CIRCLE('',#18279,1.75);
#7026=CIRCLE('',#18280,1.75);
#7027=CIRCLE('',#18281,1.75);
#7028=CIRCLE('',#18282,1.75);
#7029=CIRCLE('',#18283,1.75);
#7030=CIRCLE('',#18284,1.75);
#7031=CIRCLE('',#18285,1.75);
#7032=CIRCLE('',#18286,1.75);
#7033=CIRCLE('',#18287,1.75);
#7034=CIRCLE('',#18288,1.75);
#7035=CIRCLE('',#18289,1.75);
#7036=CIRCLE('',#18290,1.75);
#7037=CIRCLE('',#18291,1.75);
#7038=CIRCLE('',#18292,1.75);
#7039=CIRCLE('',#18293,1.75);
#7040=CIRCLE('',#18294,1.75);
#7041=CIRCLE('',#18295,1.75);
#7042=CIRCLE('',#18296,0.6);
#7043=CIRCLE('',#18298,0.6);
#7044=CIRCLE('',#18300,1.4);
#7045=CIRCLE('',#18301,1.4);
#7046=CIRCLE('',#18305,1.75);
#7047=CIRCLE('',#18308,1.75);
#7048=CIRCLE('',#18311,1.75);
#7049=CIRCLE('',#18314,1.75);
#7050=CIRCLE('',#18317,1.75);
#7051=CIRCLE('',#18320,1.75);
#7052=CIRCLE('',#18323,1.75);
#7053=CIRCLE('',#18326,1.75);
#7054=CIRCLE('',#18329,1.75);
#7055=CIRCLE('',#18332,1.75);
#7056=CIRCLE('',#18335,1.75);
#7057=CIRCLE('',#18338,1.75);
#7058=CIRCLE('',#18341,1.75);
#7059=CIRCLE('',#18344,1.75);
#7060=CIRCLE('',#18347,1.75);
#7061=CIRCLE('',#18350,1.75);
#7062=CIRCLE('',#18353,1.75);
#7063=CIRCLE('',#18356,1.75);
#7064=CIRCLE('',#18359,1.75);
#7065=CIRCLE('',#18362,1.75);
#8033=VERTEX_POINT('',#26779);
#8034=VERTEX_POINT('',#26780);
#8035=VERTEX_POINT('',#26782);
#8036=VERTEX_POINT('',#26784);
#8037=VERTEX_POINT('',#26788);
#8038=VERTEX_POINT('',#26790);
#8039=VERTEX_POINT('',#26794);
#8040=VERTEX_POINT('',#26796);
#8041=VERTEX_POINT('',#26800);
#8042=VERTEX_POINT('',#26801);
#8043=VERTEX_POINT('',#26803);
#8044=VERTEX_POINT('',#26874);
#8045=VERTEX_POINT('',#26876);
#8046=VERTEX_POINT('',#26947);
#8047=VERTEX_POINT('',#26949);
#8048=VERTEX_POINT('',#27020);
#8049=VERTEX_POINT('',#27022);
#8050=VERTEX_POINT('',#27093);
#8051=VERTEX_POINT('',#27095);
#8052=VERTEX_POINT('',#27166);
#8053=VERTEX_POINT('',#27168);
#8054=VERTEX_POINT('',#27239);
#8055=VERTEX_POINT('',#27241);
#8056=VERTEX_POINT('',#27312);
#8057=VERTEX_POINT('',#27314);
#8058=VERTEX_POINT('',#27385);
#8059=VERTEX_POINT('',#27387);
#8060=VERTEX_POINT('',#27458);
#8061=VERTEX_POINT('',#27460);
#8062=VERTEX_POINT('',#27531);
#8063=VERTEX_POINT('',#27533);
#8064=VERTEX_POINT('',#27604);
#8065=VERTEX_POINT('',#27606);
#8066=VERTEX_POINT('',#27677);
#8067=VERTEX_POINT('',#27679);
#8068=VERTEX_POINT('',#27750);
#8069=VERTEX_POINT('',#27752);
#8070=VERTEX_POINT('',#27823);
#8071=VERTEX_POINT('',#27825);
#8072=VERTEX_POINT('',#27896);
#8073=VERTEX_POINT('',#27898);
#8074=VERTEX_POINT('',#27969);
#8075=VERTEX_POINT('',#27971);
#8076=VERTEX_POINT('',#28042);
#8077=VERTEX_POINT('',#28044);
#8078=VERTEX_POINT('',#28115);
#8079=VERTEX_POINT('',#28117);
#8080=VERTEX_POINT('',#28188);
#8081=VERTEX_POINT('',#28190);
#8082=VERTEX_POINT('',#28261);
#8083=VERTEX_POINT('',#28263);
#8084=VERTEX_POINT('',#28334);
#8085=VERTEX_POINT('',#28336);
#8086=VERTEX_POINT('',#28407);
#8087=VERTEX_POINT('',#28409);
#8088=VERTEX_POINT('',#28480);
#8089=VERTEX_POINT('',#28482);
#8090=VERTEX_POINT('',#28553);
#8091=VERTEX_POINT('',#28555);
#8092=VERTEX_POINT('',#28626);
#8093=VERTEX_POINT('',#28628);
#8094=VERTEX_POINT('',#28699);
#8095=VERTEX_POINT('',#28701);
#8096=VERTEX_POINT('',#28772);
#8097=VERTEX_POINT('',#28774);
#8098=VERTEX_POINT('',#28845);
#8099=VERTEX_POINT('',#28847);
#8100=VERTEX_POINT('',#28918);
#8101=VERTEX_POINT('',#28920);
#8102=VERTEX_POINT('',#28991);
#8103=VERTEX_POINT('',#28993);
#8104=VERTEX_POINT('',#29064);
#8105=VERTEX_POINT('',#29066);
#8106=VERTEX_POINT('',#29137);
#8107=VERTEX_POINT('',#29139);
#8108=VERTEX_POINT('',#29210);
#8109=VERTEX_POINT('',#29212);
#8110=VERTEX_POINT('',#29283);
#8111=VERTEX_POINT('',#29285);
#8112=VERTEX_POINT('',#29356);
#8113=VERTEX_POINT('',#29358);
#8114=VERTEX_POINT('',#29429);
#8115=VERTEX_POINT('',#29431);
#8116=VERTEX_POINT('',#29502);
#8117=VERTEX_POINT('',#29504);
#8118=VERTEX_POINT('',#29575);
#8119=VERTEX_POINT('',#29577);
#8120=VERTEX_POINT('',#29648);
#8121=VERTEX_POINT('',#29724);
#8122=VERTEX_POINT('',#29726);
#8123=VERTEX_POINT('',#29870);
#8124=VERTEX_POINT('',#29872);
#8125=VERTEX_POINT('',#29945);
#8126=VERTEX_POINT('',#30088);
#8127=VERTEX_POINT('',#30161);
#8128=VERTEX_POINT('',#30304);
#8129=VERTEX_POINT('',#30377);
#8130=VERTEX_POINT('',#30520);
#8131=VERTEX_POINT('',#30593);
#8132=VERTEX_POINT('',#30736);
#8133=VERTEX_POINT('',#30809);
#8134=VERTEX_POINT('',#30952);
#8135=VERTEX_POINT('',#31025);
#8136=VERTEX_POINT('',#31168);
#8137=VERTEX_POINT('',#31241);
#8138=VERTEX_POINT('',#31384);
#8139=VERTEX_POINT('',#31457);
#8140=VERTEX_POINT('',#31600);
#8141=VERTEX_POINT('',#31673);
#8142=VERTEX_POINT('',#31816);
#8143=VERTEX_POINT('',#31889);
#8144=VERTEX_POINT('',#32032);
#8145=VERTEX_POINT('',#32105);
#8146=VERTEX_POINT('',#32248);
#8147=VERTEX_POINT('',#32321);
#8148=VERTEX_POINT('',#32464);
#8149=VERTEX_POINT('',#32537);
#8150=VERTEX_POINT('',#32680);
#8151=VERTEX_POINT('',#32753);
#8152=VERTEX_POINT('',#32896);
#8153=VERTEX_POINT('',#32969);
#8154=VERTEX_POINT('',#33112);
#8155=VERTEX_POINT('',#33185);
#8156=VERTEX_POINT('',#33328);
#8157=VERTEX_POINT('',#33401);
#8158=VERTEX_POINT('',#33544);
#8159=VERTEX_POINT('',#33617);
#8160=VERTEX_POINT('',#33760);
#8161=VERTEX_POINT('',#33833);
#8162=VERTEX_POINT('',#33976);
#8163=VERTEX_POINT('',#34049);
#8164=VERTEX_POINT('',#34192);
#8165=VERTEX_POINT('',#34265);
#8166=VERTEX_POINT('',#34408);
#8167=VERTEX_POINT('',#34481);
#8168=VERTEX_POINT('',#34624);
#8169=VERTEX_POINT('',#34697);
#8170=VERTEX_POINT('',#34840);
#8171=VERTEX_POINT('',#34913);
#8172=VERTEX_POINT('',#35056);
#8173=VERTEX_POINT('',#35129);
#8174=VERTEX_POINT('',#35272);
#8175=VERTEX_POINT('',#35345);
#8176=VERTEX_POINT('',#35488);
#8177=VERTEX_POINT('',#35561);
#8178=VERTEX_POINT('',#35704);
#8179=VERTEX_POINT('',#35777);
#8180=VERTEX_POINT('',#35920);
#8181=VERTEX_POINT('',#35993);
#8182=VERTEX_POINT('',#36136);
#8183=VERTEX_POINT('',#36209);
#8184=VERTEX_POINT('',#36352);
#8185=VERTEX_POINT('',#36425);
#8186=VERTEX_POINT('',#36568);
#8187=VERTEX_POINT('',#36641);
#8188=VERTEX_POINT('',#36784);
#8189=VERTEX_POINT('',#36857);
#8190=VERTEX_POINT('',#37000);
#8191=VERTEX_POINT('',#37073);
#8192=VERTEX_POINT('',#37216);
#8193=VERTEX_POINT('',#37289);
#8194=VERTEX_POINT('',#37432);
#8195=VERTEX_POINT('',#37505);
#8196=VERTEX_POINT('',#37648);
#8197=VERTEX_POINT('',#37721);
#8198=VERTEX_POINT('',#37864);
#8199=VERTEX_POINT('',#37937);
#8200=VERTEX_POINT('',#38080);
#8201=VERTEX_POINT('',#38153);
#8202=VERTEX_POINT('',#38296);
#9879=EDGE_CURVE('',#8033,#8034,#4980,.T.);
#9880=EDGE_CURVE('',#8035,#8033,#4981,.T.);
#9881=EDGE_CURVE('',#8036,#8035,#4982,.T.);
#9882=EDGE_CURVE('',#8034,#8036,#4983,.T.);
#9883=EDGE_CURVE('',#8037,#8033,#4984,.T.);
#9884=EDGE_CURVE('',#8037,#8038,#4985,.T.);
#9885=EDGE_CURVE('',#8035,#8038,#4986,.T.);
#9886=EDGE_CURVE('',#8039,#8037,#4987,.T.);
#9887=EDGE_CURVE('',#8040,#8039,#4988,.T.);
#9888=EDGE_CURVE('',#8038,#8040,#4989,.T.);
#9889=EDGE_CURVE('',#8041,#8042,#7022,.T.);
#9890=EDGE_CURVE('',#8042,#8043,#131,.T.);
#9891=EDGE_CURVE('',#8043,#8044,#4990,.T.);
#9892=EDGE_CURVE('',#8044,#8045,#132,.T.);
#9893=EDGE_CURVE('',#8045,#8046,#7023,.T.);
#9894=EDGE_CURVE('',#8046,#8047,#133,.T.);
#9895=EDGE_CURVE('',#8047,#8048,#4991,.T.);
#9896=EDGE_CURVE('',#8048,#8049,#134,.T.);
#9897=EDGE_CURVE('',#8049,#8050,#7024,.T.);
#9898=EDGE_CURVE('',#8050,#8051,#135,.T.);
#9899=EDGE_CURVE('',#8051,#8052,#4992,.T.);
#9900=EDGE_CURVE('',#8052,#8053,#136,.T.);
#9901=EDGE_CURVE('',#8053,#8054,#7025,.T.);
#9902=EDGE_CURVE('',#8054,#8055,#137,.T.);
#9903=EDGE_CURVE('',#8055,#8056,#4993,.T.);
#9904=EDGE_CURVE('',#8056,#8057,#138,.T.);
#9905=EDGE_CURVE('',#8057,#8058,#7026,.T.);
#9906=EDGE_CURVE('',#8058,#8059,#139,.T.);
#9907=EDGE_CURVE('',#8059,#8060,#4994,.T.);
#9908=EDGE_CURVE('',#8060,#8061,#140,.T.);
#9909=EDGE_CURVE('',#8061,#8062,#7027,.T.);
#9910=EDGE_CURVE('',#8062,#8063,#141,.T.);
#9911=EDGE_CURVE('',#8063,#8064,#4995,.T.);
#9912=EDGE_CURVE('',#8064,#8065,#142,.T.);
#9913=EDGE_CURVE('',#8065,#8066,#7028,.T.);
#9914=EDGE_CURVE('',#8066,#8067,#143,.T.);
#9915=EDGE_CURVE('',#8067,#8068,#4996,.T.);
#9916=EDGE_CURVE('',#8068,#8069,#144,.T.);
#9917=EDGE_CURVE('',#8069,#8070,#7029,.T.);
#9918=EDGE_CURVE('',#8070,#8071,#145,.T.);
#9919=EDGE_CURVE('',#8071,#8072,#4997,.T.);
#9920=EDGE_CURVE('',#8072,#8073,#146,.T.);
#9921=EDGE_CURVE('',#8073,#8074,#7030,.T.);
#9922=EDGE_CURVE('',#8074,#8075,#147,.T.);
#9923=EDGE_CURVE('',#8075,#8076,#4998,.T.);
#9924=EDGE_CURVE('',#8076,#8077,#148,.T.);
#9925=EDGE_CURVE('',#8077,#8078,#7031,.T.);
#9926=EDGE_CURVE('',#8078,#8079,#149,.T.);
#9927=EDGE_CURVE('',#8079,#8080,#4999,.T.);
#9928=EDGE_CURVE('',#8080,#8081,#150,.T.);
#9929=EDGE_CURVE('',#8081,#8082,#7032,.T.);
#9930=EDGE_CURVE('',#8082,#8083,#151,.T.);
#9931=EDGE_CURVE('',#8083,#8084,#5000,.T.);
#9932=EDGE_CURVE('',#8084,#8085,#152,.T.);
#9933=EDGE_CURVE('',#8085,#8086,#7033,.T.);
#9934=EDGE_CURVE('',#8086,#8087,#153,.T.);
#9935=EDGE_CURVE('',#8087,#8088,#5001,.T.);
#9936=EDGE_CURVE('',#8088,#8089,#154,.T.);
#9937=EDGE_CURVE('',#8089,#8090,#7034,.T.);
#9938=EDGE_CURVE('',#8090,#8091,#155,.T.);
#9939=EDGE_CURVE('',#8091,#8092,#5002,.T.);
#9940=EDGE_CURVE('',#8092,#8093,#156,.T.);
#9941=EDGE_CURVE('',#8093,#8094,#7035,.T.);
#9942=EDGE_CURVE('',#8094,#8095,#157,.T.);
#9943=EDGE_CURVE('',#8095,#8096,#5003,.T.);
#9944=EDGE_CURVE('',#8096,#8097,#158,.T.);
#9945=EDGE_CURVE('',#8097,#8098,#7036,.T.);
#9946=EDGE_CURVE('',#8098,#8099,#159,.T.);
#9947=EDGE_CURVE('',#8099,#8100,#5004,.T.);
#9948=EDGE_CURVE('',#8100,#8101,#160,.T.);
#9949=EDGE_CURVE('',#8101,#8102,#7037,.T.);
#9950=EDGE_CURVE('',#8102,#8103,#161,.T.);
#9951=EDGE_CURVE('',#8103,#8104,#5005,.T.);
#9952=EDGE_CURVE('',#8104,#8105,#162,.T.);
#9953=EDGE_CURVE('',#8105,#8106,#7038,.T.);
#9954=EDGE_CURVE('',#8106,#8107,#163,.T.);
#9955=EDGE_CURVE('',#8107,#8108,#5006,.T.);
#9956=EDGE_CURVE('',#8108,#8109,#164,.T.);
#9957=EDGE_CURVE('',#8109,#8110,#7039,.T.);
#9958=EDGE_CURVE('',#8110,#8111,#165,.T.);
#9959=EDGE_CURVE('',#8111,#8112,#5007,.T.);
#9960=EDGE_CURVE('',#8112,#8113,#166,.T.);
#9961=EDGE_CURVE('',#8113,#8114,#7040,.T.);
#9962=EDGE_CURVE('',#8114,#8115,#167,.T.);
#9963=EDGE_CURVE('',#8115,#8116,#5008,.T.);
#9964=EDGE_CURVE('',#8116,#8117,#168,.T.);
#9965=EDGE_CURVE('',#8117,#8118,#7041,.T.);
#9966=EDGE_CURVE('',#8118,#8119,#169,.T.);
#9967=EDGE_CURVE('',#8119,#8120,#5009,.T.);
#9968=EDGE_CURVE('',#8120,#8041,#170,.T.);
#9969=EDGE_CURVE('',#8040,#8036,#7042,.T.);
#9970=EDGE_CURVE('',#8034,#8039,#7043,.T.);
#9971=EDGE_CURVE('',#8121,#8121,#7044,.T.);
#9972=EDGE_CURVE('',#8121,#8122,#5010,.T.);
#9973=EDGE_CURVE('',#8122,#8122,#7045,.T.);
#9974=EDGE_CURVE('',#8123,#8118,#5011,.T.);
#9975=EDGE_CURVE('',#8124,#8123,#171,.T.);
#9976=EDGE_CURVE('',#8119,#8124,#5012,.T.);
#9977=EDGE_CURVE('',#8125,#8124,#5013,.T.);
#9978=EDGE_CURVE('',#8120,#8125,#5014,.T.);
#9979=EDGE_CURVE('',#8126,#8125,#172,.T.);
#9980=EDGE_CURVE('',#8041,#8126,#5015,.T.);
#9981=EDGE_CURVE('',#8127,#8126,#7046,.T.);
#9982=EDGE_CURVE('',#8127,#8042,#5016,.T.);
#9983=EDGE_CURVE('',#8128,#8127,#173,.T.);
#9984=EDGE_CURVE('',#8043,#8128,#5017,.T.);
#9985=EDGE_CURVE('',#8129,#8128,#5018,.T.);
#9986=EDGE_CURVE('',#8044,#8129,#5019,.T.);
#9987=EDGE_CURVE('',#8130,#8129,#174,.T.);
#9988=EDGE_CURVE('',#8045,#8130,#5020,.T.);
#9989=EDGE_CURVE('',#8131,#8130,#7047,.T.);
#9990=EDGE_CURVE('',#8131,#8046,#5021,.T.);
#9991=EDGE_CURVE('',#8132,#8131,#175,.T.);
#9992=EDGE_CURVE('',#8047,#8132,#5022,.T.);
#9993=EDGE_CURVE('',#8133,#8132,#5023,.T.);
#9994=EDGE_CURVE('',#8048,#8133,#5024,.T.);
#9995=EDGE_CURVE('',#8134,#8133,#176,.T.);
#9996=EDGE_CURVE('',#8049,#8134,#5025,.T.);
#9997=EDGE_CURVE('',#8135,#8134,#7048,.T.);
#9998=EDGE_CURVE('',#8135,#8050,#5026,.T.);
#9999=EDGE_CURVE('',#8136,#8135,#177,.T.);
#10000=EDGE_CURVE('',#8051,#8136,#5027,.T.);
#10001=EDGE_CURVE('',#8137,#8136,#5028,.T.);
#10002=EDGE_CURVE('',#8052,#8137,#5029,.T.);
#10003=EDGE_CURVE('',#8138,#8137,#178,.T.);
#10004=EDGE_CURVE('',#8053,#8138,#5030,.T.);
#10005=EDGE_CURVE('',#8139,#8138,#7049,.T.);
#10006=EDGE_CURVE('',#8139,#8054,#5031,.T.);
#10007=EDGE_CURVE('',#8140,#8139,#179,.T.);
#10008=EDGE_CURVE('',#8055,#8140,#5032,.T.);
#10009=EDGE_CURVE('',#8141,#8140,#5033,.T.);
#10010=EDGE_CURVE('',#8056,#8141,#5034,.T.);
#10011=EDGE_CURVE('',#8142,#8141,#180,.T.);
#10012=EDGE_CURVE('',#8057,#8142,#5035,.T.);
#10013=EDGE_CURVE('',#8143,#8142,#7050,.T.);
#10014=EDGE_CURVE('',#8143,#8058,#5036,.T.);
#10015=EDGE_CURVE('',#8144,#8143,#181,.T.);
#10016=EDGE_CURVE('',#8059,#8144,#5037,.T.);
#10017=EDGE_CURVE('',#8145,#8144,#5038,.T.);
#10018=EDGE_CURVE('',#8060,#8145,#5039,.T.);
#10019=EDGE_CURVE('',#8146,#8145,#182,.T.);
#10020=EDGE_CURVE('',#8061,#8146,#5040,.T.);
#10021=EDGE_CURVE('',#8147,#8146,#7051,.T.);
#10022=EDGE_CURVE('',#8147,#8062,#5041,.T.);
#10023=EDGE_CURVE('',#8148,#8147,#183,.T.);
#10024=EDGE_CURVE('',#8063,#8148,#5042,.T.);
#10025=EDGE_CURVE('',#8149,#8148,#5043,.T.);
#10026=EDGE_CURVE('',#8064,#8149,#5044,.T.);
#10027=EDGE_CURVE('',#8150,#8149,#184,.T.);
#10028=EDGE_CURVE('',#8065,#8150,#5045,.T.);
#10029=EDGE_CURVE('',#8151,#8150,#7052,.T.);
#10030=EDGE_CURVE('',#8151,#8066,#5046,.T.);
#10031=EDGE_CURVE('',#8152,#8151,#185,.T.);
#10032=EDGE_CURVE('',#8067,#8152,#5047,.T.);
#10033=EDGE_CURVE('',#8153,#8152,#5048,.T.);
#10034=EDGE_CURVE('',#8068,#8153,#5049,.T.);
#10035=EDGE_CURVE('',#8154,#8153,#186,.T.);
#10036=EDGE_CURVE('',#8069,#8154,#5050,.T.);
#10037=EDGE_CURVE('',#8155,#8154,#7053,.T.);
#10038=EDGE_CURVE('',#8155,#8070,#5051,.T.);
#10039=EDGE_CURVE('',#8156,#8155,#187,.T.);
#10040=EDGE_CURVE('',#8071,#8156,#5052,.T.);
#10041=EDGE_CURVE('',#8157,#8156,#5053,.T.);
#10042=EDGE_CURVE('',#8072,#8157,#5054,.T.);
#10043=EDGE_CURVE('',#8158,#8157,#188,.T.);
#10044=EDGE_CURVE('',#8073,#8158,#5055,.T.);
#10045=EDGE_CURVE('',#8159,#8158,#7054,.T.);
#10046=EDGE_CURVE('',#8159,#8074,#5056,.T.);
#10047=EDGE_CURVE('',#8160,#8159,#189,.T.);
#10048=EDGE_CURVE('',#8075,#8160,#5057,.T.);
#10049=EDGE_CURVE('',#8161,#8160,#5058,.T.);
#10050=EDGE_CURVE('',#8076,#8161,#5059,.T.);
#10051=EDGE_CURVE('',#8162,#8161,#190,.T.);
#10052=EDGE_CURVE('',#8077,#8162,#5060,.T.);
#10053=EDGE_CURVE('',#8163,#8162,#7055,.T.);
#10054=EDGE_CURVE('',#8163,#8078,#5061,.T.);
#10055=EDGE_CURVE('',#8164,#8163,#191,.T.);
#10056=EDGE_CURVE('',#8079,#8164,#5062,.T.);
#10057=EDGE_CURVE('',#8165,#8164,#5063,.T.);
#10058=EDGE_CURVE('',#8080,#8165,#5064,.T.);
#10059=EDGE_CURVE('',#8166,#8165,#192,.T.);
#10060=EDGE_CURVE('',#8081,#8166,#5065,.T.);
#10061=EDGE_CURVE('',#8167,#8166,#7056,.T.);
#10062=EDGE_CURVE('',#8167,#8082,#5066,.T.);
#10063=EDGE_CURVE('',#8168,#8167,#193,.T.);
#10064=EDGE_CURVE('',#8083,#8168,#5067,.T.);
#10065=EDGE_CURVE('',#8169,#8168,#5068,.T.);
#10066=EDGE_CURVE('',#8084,#8169,#5069,.T.);
#10067=EDGE_CURVE('',#8170,#8169,#194,.T.);
#10068=EDGE_CURVE('',#8085,#8170,#5070,.T.);
#10069=EDGE_CURVE('',#8171,#8170,#7057,.T.);
#10070=EDGE_CURVE('',#8171,#8086,#5071,.T.);
#10071=EDGE_CURVE('',#8172,#8171,#195,.T.);
#10072=EDGE_CURVE('',#8087,#8172,#5072,.T.);
#10073=EDGE_CURVE('',#8173,#8172,#5073,.T.);
#10074=EDGE_CURVE('',#8088,#8173,#5074,.T.);
#10075=EDGE_CURVE('',#8174,#8173,#196,.T.);
#10076=EDGE_CURVE('',#8089,#8174,#5075,.T.);
#10077=EDGE_CURVE('',#8175,#8174,#7058,.T.);
#10078=EDGE_CURVE('',#8175,#8090,#5076,.T.);
#10079=EDGE_CURVE('',#8176,#8175,#197,.T.);
#10080=EDGE_CURVE('',#8091,#8176,#5077,.T.);
#10081=EDGE_CURVE('',#8177,#8176,#5078,.T.);
#10082=EDGE_CURVE('',#8092,#8177,#5079,.T.);
#10083=EDGE_CURVE('',#8178,#8177,#198,.T.);
#10084=EDGE_CURVE('',#8093,#8178,#5080,.T.);
#10085=EDGE_CURVE('',#8179,#8178,#7059,.T.);
#10086=EDGE_CURVE('',#8179,#8094,#5081,.T.);
#10087=EDGE_CURVE('',#8180,#8179,#199,.T.);
#10088=EDGE_CURVE('',#8095,#8180,#5082,.T.);
#10089=EDGE_CURVE('',#8181,#8180,#5083,.T.);
#10090=EDGE_CURVE('',#8096,#8181,#5084,.T.);
#10091=EDGE_CURVE('',#8182,#8181,#200,.T.);
#10092=EDGE_CURVE('',#8097,#8182,#5085,.T.);
#10093=EDGE_CURVE('',#8183,#8182,#7060,.T.);
#10094=EDGE_CURVE('',#8183,#8098,#5086,.T.);
#10095=EDGE_CURVE('',#8184,#8183,#201,.T.);
#10096=EDGE_CURVE('',#8099,#8184,#5087,.T.);
#10097=EDGE_CURVE('',#8185,#8184,#5088,.T.);
#10098=EDGE_CURVE('',#8100,#8185,#5089,.T.);
#10099=EDGE_CURVE('',#8186,#8185,#202,.T.);
#10100=EDGE_CURVE('',#8101,#8186,#5090,.T.);
#10101=EDGE_CURVE('',#8187,#8186,#7061,.T.);
#10102=EDGE_CURVE('',#8187,#8102,#5091,.T.);
#10103=EDGE_CURVE('',#8188,#8187,#203,.T.);
#10104=EDGE_CURVE('',#8103,#8188,#5092,.T.);
#10105=EDGE_CURVE('',#8189,#8188,#5093,.T.);
#10106=EDGE_CURVE('',#8104,#8189,#5094,.T.);
#10107=EDGE_CURVE('',#8190,#8189,#204,.T.);
#10108=EDGE_CURVE('',#8105,#8190,#5095,.T.);
#10109=EDGE_CURVE('',#8191,#8190,#7062,.T.);
#10110=EDGE_CURVE('',#8191,#8106,#5096,.T.);
#10111=EDGE_CURVE('',#8192,#8191,#205,.T.);
#10112=EDGE_CURVE('',#8107,#8192,#5097,.T.);
#10113=EDGE_CURVE('',#8193,#8192,#5098,.T.);
#10114=EDGE_CURVE('',#8108,#8193,#5099,.T.);
#10115=EDGE_CURVE('',#8194,#8193,#206,.T.);
#10116=EDGE_CURVE('',#8109,#8194,#5100,.T.);
#10117=EDGE_CURVE('',#8195,#8194,#7063,.T.);
#10118=EDGE_CURVE('',#8195,#8110,#5101,.T.);
#10119=EDGE_CURVE('',#8196,#8195,#207,.T.);
#10120=EDGE_CURVE('',#8111,#8196,#5102,.T.);
#10121=EDGE_CURVE('',#8197,#8196,#5103,.T.);
#10122=EDGE_CURVE('',#8112,#8197,#5104,.T.);
#10123=EDGE_CURVE('',#8198,#8197,#208,.T.);
#10124=EDGE_CURVE('',#8113,#8198,#5105,.T.);
#10125=EDGE_CURVE('',#8199,#8198,#7064,.T.);
#10126=EDGE_CURVE('',#8199,#8114,#5106,.T.);
#10127=EDGE_CURVE('',#8200,#8199,#209,.T.);
#10128=EDGE_CURVE('',#8115,#8200,#5107,.T.);
#10129=EDGE_CURVE('',#8201,#8200,#5108,.T.);
#10130=EDGE_CURVE('',#8116,#8201,#5109,.T.);
#10131=EDGE_CURVE('',#8202,#8201,#210,.T.);
#10132=EDGE_CURVE('',#8117,#8202,#5110,.T.);
#10133=EDGE_CURVE('',#8123,#8202,#7065,.T.);
#13255=ORIENTED_EDGE('',*,*,#9879,.F.);
#13256=ORIENTED_EDGE('',*,*,#9880,.F.);
#13257=ORIENTED_EDGE('',*,*,#9881,.F.);
#13258=ORIENTED_EDGE('',*,*,#9882,.F.);
#13259=ORIENTED_EDGE('',*,*,#9883,.F.);
#13260=ORIENTED_EDGE('',*,*,#9884,.T.);
#13261=ORIENTED_EDGE('',*,*,#9885,.F.);
#13262=ORIENTED_EDGE('',*,*,#9880,.T.);
#13263=ORIENTED_EDGE('',*,*,#9886,.F.);
#13264=ORIENTED_EDGE('',*,*,#9887,.F.);
#13265=ORIENTED_EDGE('',*,*,#9888,.F.);
#13266=ORIENTED_EDGE('',*,*,#9884,.F.);
#13267=ORIENTED_EDGE('',*,*,#9889,.T.);
#13268=ORIENTED_EDGE('',*,*,#9890,.T.);
#13269=ORIENTED_EDGE('',*,*,#9891,.T.);
#13270=ORIENTED_EDGE('',*,*,#9892,.T.);
#13271=ORIENTED_EDGE('',*,*,#9893,.T.);
#13272=ORIENTED_EDGE('',*,*,#9894,.T.);
#13273=ORIENTED_EDGE('',*,*,#9895,.T.);
#13274=ORIENTED_EDGE('',*,*,#9896,.T.);
#13275=ORIENTED_EDGE('',*,*,#9897,.T.);
#13276=ORIENTED_EDGE('',*,*,#9898,.T.);
#13277=ORIENTED_EDGE('',*,*,#9899,.T.);
#13278=ORIENTED_EDGE('',*,*,#9900,.T.);
#13279=ORIENTED_EDGE('',*,*,#9901,.T.);
#13280=ORIENTED_EDGE('',*,*,#9902,.T.);
#13281=ORIENTED_EDGE('',*,*,#9903,.T.);
#13282=ORIENTED_EDGE('',*,*,#9904,.T.);
#13283=ORIENTED_EDGE('',*,*,#9905,.T.);
#13284=ORIENTED_EDGE('',*,*,#9906,.T.);
#13285=ORIENTED_EDGE('',*,*,#9907,.T.);
#13286=ORIENTED_EDGE('',*,*,#9908,.T.);
#13287=ORIENTED_EDGE('',*,*,#9909,.T.);
#13288=ORIENTED_EDGE('',*,*,#9910,.T.);
#13289=ORIENTED_EDGE('',*,*,#9911,.T.);
#13290=ORIENTED_EDGE('',*,*,#9912,.T.);
#13291=ORIENTED_EDGE('',*,*,#9913,.T.);
#13292=ORIENTED_EDGE('',*,*,#9914,.T.);
#13293=ORIENTED_EDGE('',*,*,#9915,.T.);
#13294=ORIENTED_EDGE('',*,*,#9916,.T.);
#13295=ORIENTED_EDGE('',*,*,#9917,.T.);
#13296=ORIENTED_EDGE('',*,*,#9918,.T.);
#13297=ORIENTED_EDGE('',*,*,#9919,.T.);
#13298=ORIENTED_EDGE('',*,*,#9920,.T.);
#13299=ORIENTED_EDGE('',*,*,#9921,.T.);
#13300=ORIENTED_EDGE('',*,*,#9922,.T.);
#13301=ORIENTED_EDGE('',*,*,#9923,.T.);
#13302=ORIENTED_EDGE('',*,*,#9924,.T.);
#13303=ORIENTED_EDGE('',*,*,#9925,.T.);
#13304=ORIENTED_EDGE('',*,*,#9926,.T.);
#13305=ORIENTED_EDGE('',*,*,#9927,.T.);
#13306=ORIENTED_EDGE('',*,*,#9928,.T.);
#13307=ORIENTED_EDGE('',*,*,#9929,.T.);
#13308=ORIENTED_EDGE('',*,*,#9930,.T.);
#13309=ORIENTED_EDGE('',*,*,#9931,.T.);
#13310=ORIENTED_EDGE('',*,*,#9932,.T.);
#13311=ORIENTED_EDGE('',*,*,#9933,.T.);
#13312=ORIENTED_EDGE('',*,*,#9934,.T.);
#13313=ORIENTED_EDGE('',*,*,#9935,.T.);
#13314=ORIENTED_EDGE('',*,*,#9936,.T.);
#13315=ORIENTED_EDGE('',*,*,#9937,.T.);
#13316=ORIENTED_EDGE('',*,*,#9938,.T.);
#13317=ORIENTED_EDGE('',*,*,#9939,.T.);
#13318=ORIENTED_EDGE('',*,*,#9940,.T.);
#13319=ORIENTED_EDGE('',*,*,#9941,.T.);
#13320=ORIENTED_EDGE('',*,*,#9942,.T.);
#13321=ORIENTED_EDGE('',*,*,#9943,.T.);
#13322=ORIENTED_EDGE('',*,*,#9944,.T.);
#13323=ORIENTED_EDGE('',*,*,#9945,.T.);
#13324=ORIENTED_EDGE('',*,*,#9946,.T.);
#13325=ORIENTED_EDGE('',*,*,#9947,.T.);
#13326=ORIENTED_EDGE('',*,*,#9948,.T.);
#13327=ORIENTED_EDGE('',*,*,#9949,.T.);
#13328=ORIENTED_EDGE('',*,*,#9950,.T.);
#13329=ORIENTED_EDGE('',*,*,#9951,.T.);
#13330=ORIENTED_EDGE('',*,*,#9952,.T.);
#13331=ORIENTED_EDGE('',*,*,#9953,.T.);
#13332=ORIENTED_EDGE('',*,*,#9954,.T.);
#13333=ORIENTED_EDGE('',*,*,#9955,.T.);
#13334=ORIENTED_EDGE('',*,*,#9956,.T.);
#13335=ORIENTED_EDGE('',*,*,#9957,.T.);
#13336=ORIENTED_EDGE('',*,*,#9958,.T.);
#13337=ORIENTED_EDGE('',*,*,#9959,.T.);
#13338=ORIENTED_EDGE('',*,*,#9960,.T.);
#13339=ORIENTED_EDGE('',*,*,#9961,.T.);
#13340=ORIENTED_EDGE('',*,*,#9962,.T.);
#13341=ORIENTED_EDGE('',*,*,#9963,.T.);
#13342=ORIENTED_EDGE('',*,*,#9964,.T.);
#13343=ORIENTED_EDGE('',*,*,#9965,.T.);
#13344=ORIENTED_EDGE('',*,*,#9966,.T.);
#13345=ORIENTED_EDGE('',*,*,#9967,.T.);
#13346=ORIENTED_EDGE('',*,*,#9968,.T.);
#13347=ORIENTED_EDGE('',*,*,#9881,.T.);
#13348=ORIENTED_EDGE('',*,*,#9885,.T.);
#13349=ORIENTED_EDGE('',*,*,#9888,.T.);
#13350=ORIENTED_EDGE('',*,*,#9969,.T.);
#13351=ORIENTED_EDGE('',*,*,#9882,.T.);
#13352=ORIENTED_EDGE('',*,*,#9969,.F.);
#13353=ORIENTED_EDGE('',*,*,#9887,.T.);
#13354=ORIENTED_EDGE('',*,*,#9970,.F.);
#13355=ORIENTED_EDGE('',*,*,#9971,.F.);
#13356=ORIENTED_EDGE('',*,*,#9972,.T.);
#13357=ORIENTED_EDGE('',*,*,#9973,.F.);
#13358=ORIENTED_EDGE('',*,*,#9972,.F.);
#13359=ORIENTED_EDGE('',*,*,#9971,.T.);
#13360=ORIENTED_EDGE('',*,*,#9879,.T.);
#13361=ORIENTED_EDGE('',*,*,#9970,.T.);
#13362=ORIENTED_EDGE('',*,*,#9886,.T.);
#13363=ORIENTED_EDGE('',*,*,#9883,.T.);
#13364=ORIENTED_EDGE('',*,*,#9974,.F.);
#13365=ORIENTED_EDGE('',*,*,#9975,.F.);
#13366=ORIENTED_EDGE('',*,*,#9976,.F.);
#13367=ORIENTED_EDGE('',*,*,#9966,.F.);
#13368=ORIENTED_EDGE('',*,*,#9976,.T.);
#13369=ORIENTED_EDGE('',*,*,#9977,.F.);
#13370=ORIENTED_EDGE('',*,*,#9978,.F.);
#13371=ORIENTED_EDGE('',*,*,#9967,.F.);
#13372=ORIENTED_EDGE('',*,*,#9978,.T.);
#13373=ORIENTED_EDGE('',*,*,#9979,.F.);
#13374=ORIENTED_EDGE('',*,*,#9980,.F.);
#13375=ORIENTED_EDGE('',*,*,#9968,.F.);
#13376=ORIENTED_EDGE('',*,*,#9980,.T.);
#13377=ORIENTED_EDGE('',*,*,#9981,.F.);
#13378=ORIENTED_EDGE('',*,*,#9982,.T.);
#13379=ORIENTED_EDGE('',*,*,#9889,.F.);
#13380=ORIENTED_EDGE('',*,*,#9982,.F.);
#13381=ORIENTED_EDGE('',*,*,#9983,.F.);
#13382=ORIENTED_EDGE('',*,*,#9984,.F.);
#13383=ORIENTED_EDGE('',*,*,#9890,.F.);
#13384=ORIENTED_EDGE('',*,*,#9984,.T.);
#13385=ORIENTED_EDGE('',*,*,#9985,.F.);
#13386=ORIENTED_EDGE('',*,*,#9986,.F.);
#13387=ORIENTED_EDGE('',*,*,#9891,.F.);
#13388=ORIENTED_EDGE('',*,*,#9986,.T.);
#13389=ORIENTED_EDGE('',*,*,#9987,.F.);
#13390=ORIENTED_EDGE('',*,*,#9988,.F.);
#13391=ORIENTED_EDGE('',*,*,#9892,.F.);
#13392=ORIENTED_EDGE('',*,*,#9988,.T.);
#13393=ORIENTED_EDGE('',*,*,#9989,.F.);
#13394=ORIENTED_EDGE('',*,*,#9990,.T.);
#13395=ORIENTED_EDGE('',*,*,#9893,.F.);
#13396=ORIENTED_EDGE('',*,*,#9990,.F.);
#13397=ORIENTED_EDGE('',*,*,#9991,.F.);
#13398=ORIENTED_EDGE('',*,*,#9992,.F.);
#13399=ORIENTED_EDGE('',*,*,#9894,.F.);
#13400=ORIENTED_EDGE('',*,*,#9992,.T.);
#13401=ORIENTED_EDGE('',*,*,#9993,.F.);
#13402=ORIENTED_EDGE('',*,*,#9994,.F.);
#13403=ORIENTED_EDGE('',*,*,#9895,.F.);
#13404=ORIENTED_EDGE('',*,*,#9994,.T.);
#13405=ORIENTED_EDGE('',*,*,#9995,.F.);
#13406=ORIENTED_EDGE('',*,*,#9996,.F.);
#13407=ORIENTED_EDGE('',*,*,#9896,.F.);
#13408=ORIENTED_EDGE('',*,*,#9996,.T.);
#13409=ORIENTED_EDGE('',*,*,#9997,.F.);
#13410=ORIENTED_EDGE('',*,*,#9998,.T.);
#13411=ORIENTED_EDGE('',*,*,#9897,.F.);
#13412=ORIENTED_EDGE('',*,*,#9998,.F.);
#13413=ORIENTED_EDGE('',*,*,#9999,.F.);
#13414=ORIENTED_EDGE('',*,*,#10000,.F.);
#13415=ORIENTED_EDGE('',*,*,#9898,.F.);
#13416=ORIENTED_EDGE('',*,*,#10000,.T.);
#13417=ORIENTED_EDGE('',*,*,#10001,.F.);
#13418=ORIENTED_EDGE('',*,*,#10002,.F.);
#13419=ORIENTED_EDGE('',*,*,#9899,.F.);
#13420=ORIENTED_EDGE('',*,*,#10002,.T.);
#13421=ORIENTED_EDGE('',*,*,#10003,.F.);
#13422=ORIENTED_EDGE('',*,*,#10004,.F.);
#13423=ORIENTED_EDGE('',*,*,#9900,.F.);
#13424=ORIENTED_EDGE('',*,*,#10004,.T.);
#13425=ORIENTED_EDGE('',*,*,#10005,.F.);
#13426=ORIENTED_EDGE('',*,*,#10006,.T.);
#13427=ORIENTED_EDGE('',*,*,#9901,.F.);
#13428=ORIENTED_EDGE('',*,*,#10006,.F.);
#13429=ORIENTED_EDGE('',*,*,#10007,.F.);
#13430=ORIENTED_EDGE('',*,*,#10008,.F.);
#13431=ORIENTED_EDGE('',*,*,#9902,.F.);
#13432=ORIENTED_EDGE('',*,*,#10008,.T.);
#13433=ORIENTED_EDGE('',*,*,#10009,.F.);
#13434=ORIENTED_EDGE('',*,*,#10010,.F.);
#13435=ORIENTED_EDGE('',*,*,#9903,.F.);
#13436=ORIENTED_EDGE('',*,*,#10010,.T.);
#13437=ORIENTED_EDGE('',*,*,#10011,.F.);
#13438=ORIENTED_EDGE('',*,*,#10012,.F.);
#13439=ORIENTED_EDGE('',*,*,#9904,.F.);
#13440=ORIENTED_EDGE('',*,*,#10012,.T.);
#13441=ORIENTED_EDGE('',*,*,#10013,.F.);
#13442=ORIENTED_EDGE('',*,*,#10014,.T.);
#13443=ORIENTED_EDGE('',*,*,#9905,.F.);
#13444=ORIENTED_EDGE('',*,*,#10014,.F.);
#13445=ORIENTED_EDGE('',*,*,#10015,.F.);
#13446=ORIENTED_EDGE('',*,*,#10016,.F.);
#13447=ORIENTED_EDGE('',*,*,#9906,.F.);
#13448=ORIENTED_EDGE('',*,*,#10016,.T.);
#13449=ORIENTED_EDGE('',*,*,#10017,.F.);
#13450=ORIENTED_EDGE('',*,*,#10018,.F.);
#13451=ORIENTED_EDGE('',*,*,#9907,.F.);
#13452=ORIENTED_EDGE('',*,*,#10018,.T.);
#13453=ORIENTED_EDGE('',*,*,#10019,.F.);
#13454=ORIENTED_EDGE('',*,*,#10020,.F.);
#13455=ORIENTED_EDGE('',*,*,#9908,.F.);
#13456=ORIENTED_EDGE('',*,*,#10020,.T.);
#13457=ORIENTED_EDGE('',*,*,#10021,.F.);
#13458=ORIENTED_EDGE('',*,*,#10022,.T.);
#13459=ORIENTED_EDGE('',*,*,#9909,.F.);
#13460=ORIENTED_EDGE('',*,*,#10022,.F.);
#13461=ORIENTED_EDGE('',*,*,#10023,.F.);
#13462=ORIENTED_EDGE('',*,*,#10024,.F.);
#13463=ORIENTED_EDGE('',*,*,#9910,.F.);
#13464=ORIENTED_EDGE('',*,*,#10024,.T.);
#13465=ORIENTED_EDGE('',*,*,#10025,.F.);
#13466=ORIENTED_EDGE('',*,*,#10026,.F.);
#13467=ORIENTED_EDGE('',*,*,#9911,.F.);
#13468=ORIENTED_EDGE('',*,*,#10026,.T.);
#13469=ORIENTED_EDGE('',*,*,#10027,.F.);
#13470=ORIENTED_EDGE('',*,*,#10028,.F.);
#13471=ORIENTED_EDGE('',*,*,#9912,.F.);
#13472=ORIENTED_EDGE('',*,*,#10028,.T.);
#13473=ORIENTED_EDGE('',*,*,#10029,.F.);
#13474=ORIENTED_EDGE('',*,*,#10030,.T.);
#13475=ORIENTED_EDGE('',*,*,#9913,.F.);
#13476=ORIENTED_EDGE('',*,*,#10030,.F.);
#13477=ORIENTED_EDGE('',*,*,#10031,.F.);
#13478=ORIENTED_EDGE('',*,*,#10032,.F.);
#13479=ORIENTED_EDGE('',*,*,#9914,.F.);
#13480=ORIENTED_EDGE('',*,*,#10032,.T.);
#13481=ORIENTED_EDGE('',*,*,#10033,.F.);
#13482=ORIENTED_EDGE('',*,*,#10034,.F.);
#13483=ORIENTED_EDGE('',*,*,#9915,.F.);
#13484=ORIENTED_EDGE('',*,*,#10034,.T.);
#13485=ORIENTED_EDGE('',*,*,#10035,.F.);
#13486=ORIENTED_EDGE('',*,*,#10036,.F.);
#13487=ORIENTED_EDGE('',*,*,#9916,.F.);
#13488=ORIENTED_EDGE('',*,*,#10036,.T.);
#13489=ORIENTED_EDGE('',*,*,#10037,.F.);
#13490=ORIENTED_EDGE('',*,*,#10038,.T.);
#13491=ORIENTED_EDGE('',*,*,#9917,.F.);
#13492=ORIENTED_EDGE('',*,*,#10038,.F.);
#13493=ORIENTED_EDGE('',*,*,#10039,.F.);
#13494=ORIENTED_EDGE('',*,*,#10040,.F.);
#13495=ORIENTED_EDGE('',*,*,#9918,.F.);
#13496=ORIENTED_EDGE('',*,*,#10040,.T.);
#13497=ORIENTED_EDGE('',*,*,#10041,.F.);
#13498=ORIENTED_EDGE('',*,*,#10042,.F.);
#13499=ORIENTED_EDGE('',*,*,#9919,.F.);
#13500=ORIENTED_EDGE('',*,*,#10042,.T.);
#13501=ORIENTED_EDGE('',*,*,#10043,.F.);
#13502=ORIENTED_EDGE('',*,*,#10044,.F.);
#13503=ORIENTED_EDGE('',*,*,#9920,.F.);
#13504=ORIENTED_EDGE('',*,*,#10044,.T.);
#13505=ORIENTED_EDGE('',*,*,#10045,.F.);
#13506=ORIENTED_EDGE('',*,*,#10046,.T.);
#13507=ORIENTED_EDGE('',*,*,#9921,.F.);
#13508=ORIENTED_EDGE('',*,*,#10046,.F.);
#13509=ORIENTED_EDGE('',*,*,#10047,.F.);
#13510=ORIENTED_EDGE('',*,*,#10048,.F.);
#13511=ORIENTED_EDGE('',*,*,#9922,.F.);
#13512=ORIENTED_EDGE('',*,*,#10048,.T.);
#13513=ORIENTED_EDGE('',*,*,#10049,.F.);
#13514=ORIENTED_EDGE('',*,*,#10050,.F.);
#13515=ORIENTED_EDGE('',*,*,#9923,.F.);
#13516=ORIENTED_EDGE('',*,*,#10050,.T.);
#13517=ORIENTED_EDGE('',*,*,#10051,.F.);
#13518=ORIENTED_EDGE('',*,*,#10052,.F.);
#13519=ORIENTED_EDGE('',*,*,#9924,.F.);
#13520=ORIENTED_EDGE('',*,*,#10052,.T.);
#13521=ORIENTED_EDGE('',*,*,#10053,.F.);
#13522=ORIENTED_EDGE('',*,*,#10054,.T.);
#13523=ORIENTED_EDGE('',*,*,#9925,.F.);
#13524=ORIENTED_EDGE('',*,*,#10054,.F.);
#13525=ORIENTED_EDGE('',*,*,#10055,.F.);
#13526=ORIENTED_EDGE('',*,*,#10056,.F.);
#13527=ORIENTED_EDGE('',*,*,#9926,.F.);
#13528=ORIENTED_EDGE('',*,*,#10056,.T.);
#13529=ORIENTED_EDGE('',*,*,#10057,.F.);
#13530=ORIENTED_EDGE('',*,*,#10058,.F.);
#13531=ORIENTED_EDGE('',*,*,#9927,.F.);
#13532=ORIENTED_EDGE('',*,*,#10058,.T.);
#13533=ORIENTED_EDGE('',*,*,#10059,.F.);
#13534=ORIENTED_EDGE('',*,*,#10060,.F.);
#13535=ORIENTED_EDGE('',*,*,#9928,.F.);
#13536=ORIENTED_EDGE('',*,*,#10060,.T.);
#13537=ORIENTED_EDGE('',*,*,#10061,.F.);
#13538=ORIENTED_EDGE('',*,*,#10062,.T.);
#13539=ORIENTED_EDGE('',*,*,#9929,.F.);
#13540=ORIENTED_EDGE('',*,*,#10062,.F.);
#13541=ORIENTED_EDGE('',*,*,#10063,.F.);
#13542=ORIENTED_EDGE('',*,*,#10064,.F.);
#13543=ORIENTED_EDGE('',*,*,#9930,.F.);
#13544=ORIENTED_EDGE('',*,*,#10064,.T.);
#13545=ORIENTED_EDGE('',*,*,#10065,.F.);
#13546=ORIENTED_EDGE('',*,*,#10066,.F.);
#13547=ORIENTED_EDGE('',*,*,#9931,.F.);
#13548=ORIENTED_EDGE('',*,*,#10066,.T.);
#13549=ORIENTED_EDGE('',*,*,#10067,.F.);
#13550=ORIENTED_EDGE('',*,*,#10068,.F.);
#13551=ORIENTED_EDGE('',*,*,#9932,.F.);
#13552=ORIENTED_EDGE('',*,*,#10068,.T.);
#13553=ORIENTED_EDGE('',*,*,#10069,.F.);
#13554=ORIENTED_EDGE('',*,*,#10070,.T.);
#13555=ORIENTED_EDGE('',*,*,#9933,.F.);
#13556=ORIENTED_EDGE('',*,*,#10070,.F.);
#13557=ORIENTED_EDGE('',*,*,#10071,.F.);
#13558=ORIENTED_EDGE('',*,*,#10072,.F.);
#13559=ORIENTED_EDGE('',*,*,#9934,.F.);
#13560=ORIENTED_EDGE('',*,*,#10072,.T.);
#13561=ORIENTED_EDGE('',*,*,#10073,.F.);
#13562=ORIENTED_EDGE('',*,*,#10074,.F.);
#13563=ORIENTED_EDGE('',*,*,#9935,.F.);
#13564=ORIENTED_EDGE('',*,*,#10074,.T.);
#13565=ORIENTED_EDGE('',*,*,#10075,.F.);
#13566=ORIENTED_EDGE('',*,*,#10076,.F.);
#13567=ORIENTED_EDGE('',*,*,#9936,.F.);
#13568=ORIENTED_EDGE('',*,*,#10076,.T.);
#13569=ORIENTED_EDGE('',*,*,#10077,.F.);
#13570=ORIENTED_EDGE('',*,*,#10078,.T.);
#13571=ORIENTED_EDGE('',*,*,#9937,.F.);
#13572=ORIENTED_EDGE('',*,*,#10078,.F.);
#13573=ORIENTED_EDGE('',*,*,#10079,.F.);
#13574=ORIENTED_EDGE('',*,*,#10080,.F.);
#13575=ORIENTED_EDGE('',*,*,#9938,.F.);
#13576=ORIENTED_EDGE('',*,*,#10080,.T.);
#13577=ORIENTED_EDGE('',*,*,#10081,.F.);
#13578=ORIENTED_EDGE('',*,*,#10082,.F.);
#13579=ORIENTED_EDGE('',*,*,#9939,.F.);
#13580=ORIENTED_EDGE('',*,*,#10082,.T.);
#13581=ORIENTED_EDGE('',*,*,#10083,.F.);
#13582=ORIENTED_EDGE('',*,*,#10084,.F.);
#13583=ORIENTED_EDGE('',*,*,#9940,.F.);
#13584=ORIENTED_EDGE('',*,*,#10084,.T.);
#13585=ORIENTED_EDGE('',*,*,#10085,.F.);
#13586=ORIENTED_EDGE('',*,*,#10086,.T.);
#13587=ORIENTED_EDGE('',*,*,#9941,.F.);
#13588=ORIENTED_EDGE('',*,*,#10086,.F.);
#13589=ORIENTED_EDGE('',*,*,#10087,.F.);
#13590=ORIENTED_EDGE('',*,*,#10088,.F.);
#13591=ORIENTED_EDGE('',*,*,#9942,.F.);
#13592=ORIENTED_EDGE('',*,*,#10088,.T.);
#13593=ORIENTED_EDGE('',*,*,#10089,.F.);
#13594=ORIENTED_EDGE('',*,*,#10090,.F.);
#13595=ORIENTED_EDGE('',*,*,#9943,.F.);
#13596=ORIENTED_EDGE('',*,*,#10090,.T.);
#13597=ORIENTED_EDGE('',*,*,#10091,.F.);
#13598=ORIENTED_EDGE('',*,*,#10092,.F.);
#13599=ORIENTED_EDGE('',*,*,#9944,.F.);
#13600=ORIENTED_EDGE('',*,*,#10092,.T.);
#13601=ORIENTED_EDGE('',*,*,#10093,.F.);
#13602=ORIENTED_EDGE('',*,*,#10094,.T.);
#13603=ORIENTED_EDGE('',*,*,#9945,.F.);
#13604=ORIENTED_EDGE('',*,*,#10094,.F.);
#13605=ORIENTED_EDGE('',*,*,#10095,.F.);
#13606=ORIENTED_EDGE('',*,*,#10096,.F.);
#13607=ORIENTED_EDGE('',*,*,#9946,.F.);
#13608=ORIENTED_EDGE('',*,*,#10096,.T.);
#13609=ORIENTED_EDGE('',*,*,#10097,.F.);
#13610=ORIENTED_EDGE('',*,*,#10098,.F.);
#13611=ORIENTED_EDGE('',*,*,#9947,.F.);
#13612=ORIENTED_EDGE('',*,*,#10098,.T.);
#13613=ORIENTED_EDGE('',*,*,#10099,.F.);
#13614=ORIENTED_EDGE('',*,*,#10100,.F.);
#13615=ORIENTED_EDGE('',*,*,#9948,.F.);
#13616=ORIENTED_EDGE('',*,*,#10100,.T.);
#13617=ORIENTED_EDGE('',*,*,#10101,.F.);
#13618=ORIENTED_EDGE('',*,*,#10102,.T.);
#13619=ORIENTED_EDGE('',*,*,#9949,.F.);
#13620=ORIENTED_EDGE('',*,*,#10102,.F.);
#13621=ORIENTED_EDGE('',*,*,#10103,.F.);
#13622=ORIENTED_EDGE('',*,*,#10104,.F.);
#13623=ORIENTED_EDGE('',*,*,#9950,.F.);
#13624=ORIENTED_EDGE('',*,*,#10104,.T.);
#13625=ORIENTED_EDGE('',*,*,#10105,.F.);
#13626=ORIENTED_EDGE('',*,*,#10106,.F.);
#13627=ORIENTED_EDGE('',*,*,#9951,.F.);
#13628=ORIENTED_EDGE('',*,*,#10106,.T.);
#13629=ORIENTED_EDGE('',*,*,#10107,.F.);
#13630=ORIENTED_EDGE('',*,*,#10108,.F.);
#13631=ORIENTED_EDGE('',*,*,#9952,.F.);
#13632=ORIENTED_EDGE('',*,*,#10108,.T.);
#13633=ORIENTED_EDGE('',*,*,#10109,.F.);
#13634=ORIENTED_EDGE('',*,*,#10110,.T.);
#13635=ORIENTED_EDGE('',*,*,#9953,.F.);
#13636=ORIENTED_EDGE('',*,*,#10110,.F.);
#13637=ORIENTED_EDGE('',*,*,#10111,.F.);
#13638=ORIENTED_EDGE('',*,*,#10112,.F.);
#13639=ORIENTED_EDGE('',*,*,#9954,.F.);
#13640=ORIENTED_EDGE('',*,*,#10112,.T.);
#13641=ORIENTED_EDGE('',*,*,#10113,.F.);
#13642=ORIENTED_EDGE('',*,*,#10114,.F.);
#13643=ORIENTED_EDGE('',*,*,#9955,.F.);
#13644=ORIENTED_EDGE('',*,*,#10114,.T.);
#13645=ORIENTED_EDGE('',*,*,#10115,.F.);
#13646=ORIENTED_EDGE('',*,*,#10116,.F.);
#13647=ORIENTED_EDGE('',*,*,#9956,.F.);
#13648=ORIENTED_EDGE('',*,*,#10116,.T.);
#13649=ORIENTED_EDGE('',*,*,#10117,.F.);
#13650=ORIENTED_EDGE('',*,*,#10118,.T.);
#13651=ORIENTED_EDGE('',*,*,#9957,.F.);
#13652=ORIENTED_EDGE('',*,*,#10118,.F.);
#13653=ORIENTED_EDGE('',*,*,#10119,.F.);
#13654=ORIENTED_EDGE('',*,*,#10120,.F.);
#13655=ORIENTED_EDGE('',*,*,#9958,.F.);
#13656=ORIENTED_EDGE('',*,*,#10120,.T.);
#13657=ORIENTED_EDGE('',*,*,#10121,.F.);
#13658=ORIENTED_EDGE('',*,*,#10122,.F.);
#13659=ORIENTED_EDGE('',*,*,#9959,.F.);
#13660=ORIENTED_EDGE('',*,*,#10122,.T.);
#13661=ORIENTED_EDGE('',*,*,#10123,.F.);
#13662=ORIENTED_EDGE('',*,*,#10124,.F.);
#13663=ORIENTED_EDGE('',*,*,#9960,.F.);
#13664=ORIENTED_EDGE('',*,*,#10124,.T.);
#13665=ORIENTED_EDGE('',*,*,#10125,.F.);
#13666=ORIENTED_EDGE('',*,*,#10126,.T.);
#13667=ORIENTED_EDGE('',*,*,#9961,.F.);
#13668=ORIENTED_EDGE('',*,*,#10126,.F.);
#13669=ORIENTED_EDGE('',*,*,#10127,.F.);
#13670=ORIENTED_EDGE('',*,*,#10128,.F.);
#13671=ORIENTED_EDGE('',*,*,#9962,.F.);
#13672=ORIENTED_EDGE('',*,*,#10128,.T.);
#13673=ORIENTED_EDGE('',*,*,#10129,.F.);
#13674=ORIENTED_EDGE('',*,*,#10130,.F.);
#13675=ORIENTED_EDGE('',*,*,#9963,.F.);
#13676=ORIENTED_EDGE('',*,*,#10130,.T.);
#13677=ORIENTED_EDGE('',*,*,#10131,.F.);
#13678=ORIENTED_EDGE('',*,*,#10132,.F.);
#13679=ORIENTED_EDGE('',*,*,#9964,.F.);
#13680=ORIENTED_EDGE('',*,*,#10133,.T.);
#13681=ORIENTED_EDGE('',*,*,#10131,.T.);
#13682=ORIENTED_EDGE('',*,*,#10129,.T.);
#13683=ORIENTED_EDGE('',*,*,#10127,.T.);
#13684=ORIENTED_EDGE('',*,*,#10125,.T.);
#13685=ORIENTED_EDGE('',*,*,#10123,.T.);
#13686=ORIENTED_EDGE('',*,*,#10121,.T.);
#13687=ORIENTED_EDGE('',*,*,#10119,.T.);
#13688=ORIENTED_EDGE('',*,*,#10117,.T.);
#13689=ORIENTED_EDGE('',*,*,#10115,.T.);
#13690=ORIENTED_EDGE('',*,*,#10113,.T.);
#13691=ORIENTED_EDGE('',*,*,#10111,.T.);
#13692=ORIENTED_EDGE('',*,*,#10109,.T.);
#13693=ORIENTED_EDGE('',*,*,#10107,.T.);
#13694=ORIENTED_EDGE('',*,*,#10105,.T.);
#13695=ORIENTED_EDGE('',*,*,#10103,.T.);
#13696=ORIENTED_EDGE('',*,*,#10101,.T.);
#13697=ORIENTED_EDGE('',*,*,#10099,.T.);
#13698=ORIENTED_EDGE('',*,*,#10097,.T.);
#13699=ORIENTED_EDGE('',*,*,#10095,.T.);
#13700=ORIENTED_EDGE('',*,*,#10093,.T.);
#13701=ORIENTED_EDGE('',*,*,#10091,.T.);
#13702=ORIENTED_EDGE('',*,*,#10089,.T.);
#13703=ORIENTED_EDGE('',*,*,#10087,.T.);
#13704=ORIENTED_EDGE('',*,*,#10085,.T.);
#13705=ORIENTED_EDGE('',*,*,#10083,.T.);
#13706=ORIENTED_EDGE('',*,*,#10081,.T.);
#13707=ORIENTED_EDGE('',*,*,#10079,.T.);
#13708=ORIENTED_EDGE('',*,*,#10077,.T.);
#13709=ORIENTED_EDGE('',*,*,#10075,.T.);
#13710=ORIENTED_EDGE('',*,*,#10073,.T.);
#13711=ORIENTED_EDGE('',*,*,#10071,.T.);
#13712=ORIENTED_EDGE('',*,*,#10069,.T.);
#13713=ORIENTED_EDGE('',*,*,#10067,.T.);
#13714=ORIENTED_EDGE('',*,*,#10065,.T.);
#13715=ORIENTED_EDGE('',*,*,#10063,.T.);
#13716=ORIENTED_EDGE('',*,*,#10061,.T.);
#13717=ORIENTED_EDGE('',*,*,#10059,.T.);
#13718=ORIENTED_EDGE('',*,*,#10057,.T.);
#13719=ORIENTED_EDGE('',*,*,#10055,.T.);
#13720=ORIENTED_EDGE('',*,*,#10053,.T.);
#13721=ORIENTED_EDGE('',*,*,#10051,.T.);
#13722=ORIENTED_EDGE('',*,*,#10049,.T.);
#13723=ORIENTED_EDGE('',*,*,#10047,.T.);
#13724=ORIENTED_EDGE('',*,*,#10045,.T.);
#13725=ORIENTED_EDGE('',*,*,#10043,.T.);
#13726=ORIENTED_EDGE('',*,*,#10041,.T.);
#13727=ORIENTED_EDGE('',*,*,#10039,.T.);
#13728=ORIENTED_EDGE('',*,*,#10037,.T.);
#13729=ORIENTED_EDGE('',*,*,#10035,.T.);
#13730=ORIENTED_EDGE('',*,*,#10033,.T.);
#13731=ORIENTED_EDGE('',*,*,#10031,.T.);
#13732=ORIENTED_EDGE('',*,*,#10029,.T.);
#13733=ORIENTED_EDGE('',*,*,#10027,.T.);
#13734=ORIENTED_EDGE('',*,*,#10025,.T.);
#13735=ORIENTED_EDGE('',*,*,#10023,.T.);
#13736=ORIENTED_EDGE('',*,*,#10021,.T.);
#13737=ORIENTED_EDGE('',*,*,#10019,.T.);
#13738=ORIENTED_EDGE('',*,*,#10017,.T.);
#13739=ORIENTED_EDGE('',*,*,#10015,.T.);
#13740=ORIENTED_EDGE('',*,*,#10013,.T.);
#13741=ORIENTED_EDGE('',*,*,#10011,.T.);
#13742=ORIENTED_EDGE('',*,*,#10009,.T.);
#13743=ORIENTED_EDGE('',*,*,#10007,.T.);
#13744=ORIENTED_EDGE('',*,*,#10005,.T.);
#13745=ORIENTED_EDGE('',*,*,#10003,.T.);
#13746=ORIENTED_EDGE('',*,*,#10001,.T.);
#13747=ORIENTED_EDGE('',*,*,#9999,.T.);
#13748=ORIENTED_EDGE('',*,*,#9997,.T.);
#13749=ORIENTED_EDGE('',*,*,#9995,.T.);
#13750=ORIENTED_EDGE('',*,*,#9993,.T.);
#13751=ORIENTED_EDGE('',*,*,#9991,.T.);
#13752=ORIENTED_EDGE('',*,*,#9989,.T.);
#13753=ORIENTED_EDGE('',*,*,#9987,.T.);
#13754=ORIENTED_EDGE('',*,*,#9985,.T.);
#13755=ORIENTED_EDGE('',*,*,#9983,.T.);
#13756=ORIENTED_EDGE('',*,*,#9981,.T.);
#13757=ORIENTED_EDGE('',*,*,#9979,.T.);
#13758=ORIENTED_EDGE('',*,*,#9977,.T.);
#13759=ORIENTED_EDGE('',*,*,#9975,.T.);
#13760=ORIENTED_EDGE('',*,*,#9973,.T.);
#13761=ORIENTED_EDGE('',*,*,#9974,.T.);
#13762=ORIENTED_EDGE('',*,*,#9965,.F.);
#13763=ORIENTED_EDGE('',*,*,#10132,.T.);
#13764=ORIENTED_EDGE('',*,*,#10133,.F.);
#15344=CYLINDRICAL_SURFACE('',#18297,0.6);
#15345=CYLINDRICAL_SURFACE('',#18299,1.4);
#15346=CYLINDRICAL_SURFACE('',#18304,1.75);
#15347=CYLINDRICAL_SURFACE('',#18307,1.75);
#15348=CYLINDRICAL_SURFACE('',#18310,1.75);
#15349=CYLINDRICAL_SURFACE('',#18313,1.75);
#15350=CYLINDRICAL_SURFACE('',#18316,1.75);
#15351=CYLINDRICAL_SURFACE('',#18319,1.75);
#15352=CYLINDRICAL_SURFACE('',#18322,1.75);
#15353=CYLINDRICAL_SURFACE('',#18325,1.75);
#15354=CYLINDRICAL_SURFACE('',#18328,1.75);
#15355=CYLINDRICAL_SURFACE('',#18331,1.75);
#15356=CYLINDRICAL_SURFACE('',#18334,1.75);
#15357=CYLINDRICAL_SURFACE('',#18337,1.75);
#15358=CYLINDRICAL_SURFACE('',#18340,1.75);
#15359=CYLINDRICAL_SURFACE('',#18343,1.75);
#15360=CYLINDRICAL_SURFACE('',#18346,1.75);
#15361=CYLINDRICAL_SURFACE('',#18349,1.75);
#15362=CYLINDRICAL_SURFACE('',#18352,1.75);
#15363=CYLINDRICAL_SURFACE('',#18355,1.75);
#15364=CYLINDRICAL_SURFACE('',#18358,1.75);
#15365=CYLINDRICAL_SURFACE('',#18363,1.75);
#16008=ADVANCED_FACE('',(#2698),#1977,.F.);
#16009=ADVANCED_FACE('',(#2699),#1978,.F.);
#16010=ADVANCED_FACE('',(#2700),#1979,.F.);
#16011=ADVANCED_FACE('',(#2701,#1600),#1980,.F.);
#16012=ADVANCED_FACE('',(#2702),#15344,.F.);
#16013=ADVANCED_FACE('',(#2703),#15345,.T.);
#16014=ADVANCED_FACE('',(#2704,#1601),#1981,.T.);
#16015=ADVANCED_FACE('',(#2705),#11,.T.);
#16016=ADVANCED_FACE('',(#2706),#1982,.T.);
#16017=ADVANCED_FACE('',(#2707),#12,.T.);
#16018=ADVANCED_FACE('',(#2708),#15346,.T.);
#16019=ADVANCED_FACE('',(#2709),#13,.T.);
#16020=ADVANCED_FACE('',(#2710),#1983,.T.);
#16021=ADVANCED_FACE('',(#2711),#14,.T.);
#16022=ADVANCED_FACE('',(#2712),#15347,.T.);
#16023=ADVANCED_FACE('',(#2713),#15,.T.);
#16024=ADVANCED_FACE('',(#2714),#1984,.T.);
#16025=ADVANCED_FACE('',(#2715),#16,.T.);
#16026=ADVANCED_FACE('',(#2716),#15348,.T.);
#16027=ADVANCED_FACE('',(#2717),#17,.T.);
#16028=ADVANCED_FACE('',(#2718),#1985,.T.);
#16029=ADVANCED_FACE('',(#2719),#18,.T.);
#16030=ADVANCED_FACE('',(#2720),#15349,.T.);
#16031=ADVANCED_FACE('',(#2721),#19,.T.);
#16032=ADVANCED_FACE('',(#2722),#1986,.T.);
#16033=ADVANCED_FACE('',(#2723),#20,.T.);
#16034=ADVANCED_FACE('',(#2724),#15350,.T.);
#16035=ADVANCED_FACE('',(#2725),#21,.T.);
#16036=ADVANCED_FACE('',(#2726),#1987,.T.);
#16037=ADVANCED_FACE('',(#2727),#22,.T.);
#16038=ADVANCED_FACE('',(#2728),#15351,.T.);
#16039=ADVANCED_FACE('',(#2729),#23,.T.);
#16040=ADVANCED_FACE('',(#2730),#1988,.T.);
#16041=ADVANCED_FACE('',(#2731),#24,.T.);
#16042=ADVANCED_FACE('',(#2732),#15352,.T.);
#16043=ADVANCED_FACE('',(#2733),#25,.T.);
#16044=ADVANCED_FACE('',(#2734),#1989,.T.);
#16045=ADVANCED_FACE('',(#2735),#26,.T.);
#16046=ADVANCED_FACE('',(#2736),#15353,.T.);
#16047=ADVANCED_FACE('',(#2737),#27,.T.);
#16048=ADVANCED_FACE('',(#2738),#1990,.T.);
#16049=ADVANCED_FACE('',(#2739),#28,.T.);
#16050=ADVANCED_FACE('',(#2740),#15354,.T.);
#16051=ADVANCED_FACE('',(#2741),#29,.T.);
#16052=ADVANCED_FACE('',(#2742),#1991,.T.);
#16053=ADVANCED_FACE('',(#2743),#30,.T.);
#16054=ADVANCED_FACE('',(#2744),#15355,.T.);
#16055=ADVANCED_FACE('',(#2745),#31,.T.);
#16056=ADVANCED_FACE('',(#2746),#1992,.T.);
#16057=ADVANCED_FACE('',(#2747),#32,.T.);
#16058=ADVANCED_FACE('',(#2748),#15356,.T.);
#16059=ADVANCED_FACE('',(#2749),#33,.T.);
#16060=ADVANCED_FACE('',(#2750),#1993,.T.);
#16061=ADVANCED_FACE('',(#2751),#34,.T.);
#16062=ADVANCED_FACE('',(#2752),#15357,.T.);
#16063=ADVANCED_FACE('',(#2753),#35,.T.);
#16064=ADVANCED_FACE('',(#2754),#1994,.T.);
#16065=ADVANCED_FACE('',(#2755),#36,.T.);
#16066=ADVANCED_FACE('',(#2756),#15358,.T.);
#16067=ADVANCED_FACE('',(#2757),#37,.T.);
#16068=ADVANCED_FACE('',(#2758),#1995,.T.);
#16069=ADVANCED_FACE('',(#2759),#38,.T.);
#16070=ADVANCED_FACE('',(#2760),#15359,.T.);
#16071=ADVANCED_FACE('',(#2761),#39,.T.);
#16072=ADVANCED_FACE('',(#2762),#1996,.T.);
#16073=ADVANCED_FACE('',(#2763),#40,.T.);
#16074=ADVANCED_FACE('',(#2764),#15360,.T.);
#16075=ADVANCED_FACE('',(#2765),#41,.T.);
#16076=ADVANCED_FACE('',(#2766),#1997,.T.);
#16077=ADVANCED_FACE('',(#2767),#42,.T.);
#16078=ADVANCED_FACE('',(#2768),#15361,.T.);
#16079=ADVANCED_FACE('',(#2769),#43,.T.);
#16080=ADVANCED_FACE('',(#2770),#1998,.T.);
#16081=ADVANCED_FACE('',(#2771),#44,.T.);
#16082=ADVANCED_FACE('',(#2772),#15362,.T.);
#16083=ADVANCED_FACE('',(#2773),#45,.T.);
#16084=ADVANCED_FACE('',(#2774),#1999,.T.);
#16085=ADVANCED_FACE('',(#2775),#46,.T.);
#16086=ADVANCED_FACE('',(#2776),#15363,.T.);
#16087=ADVANCED_FACE('',(#2777),#47,.T.);
#16088=ADVANCED_FACE('',(#2778),#2000,.T.);
#16089=ADVANCED_FACE('',(#2779),#48,.T.);
#16090=ADVANCED_FACE('',(#2780),#15364,.T.);
#16091=ADVANCED_FACE('',(#2781),#49,.T.);
#16092=ADVANCED_FACE('',(#2782),#2001,.T.);
#16093=ADVANCED_FACE('',(#2783),#50,.T.);
#16094=ADVANCED_FACE('',(#2784,#1602),#2002,.T.);
#16095=ADVANCED_FACE('',(#2785),#15365,.T.);
#16437=CLOSED_SHELL('',(#16008,#16009,#16010,#16011,#16012,#16013,#16014,
#16015,#16016,#16017,#16018,#16019,#16020,#16021,#16022,#16023,#16024,#16025,
#16026,#16027,#16028,#16029,#16030,#16031,#16032,#16033,#16034,#16035,#16036,
#16037,#16038,#16039,#16040,#16041,#16042,#16043,#16044,#16045,#16046,#16047,
#16048,#16049,#16050,#16051,#16052,#16053,#16054,#16055,#16056,#16057,#16058,
#16059,#16060,#16061,#16062,#16063,#16064,#16065,#16066,#16067,#16068,#16069,
#16070,#16071,#16072,#16073,#16074,#16075,#16076,#16077,#16078,#16079,#16080,
#16081,#16082,#16083,#16084,#16085,#16086,#16087,#16088,#16089,#16090,#16091,
#16092,#16093,#16094,#16095));
#18271=AXIS2_PLACEMENT_3D('',#26777,#21751,#21752);
#18272=AXIS2_PLACEMENT_3D('',#26778,#21753,#21754);
#18273=AXIS2_PLACEMENT_3D('',#26787,#21759,#21760);
#18274=AXIS2_PLACEMENT_3D('',#26793,#21764,#21765);
#18275=AXIS2_PLACEMENT_3D('',#26799,#21769,#21770);
#18276=AXIS2_PLACEMENT_3D('',#26802,#21771,#21772);
#18277=AXIS2_PLACEMENT_3D('',#26948,#21774,#21775);
#18278=AXIS2_PLACEMENT_3D('',#27094,#21777,#21778);
#18279=AXIS2_PLACEMENT_3D('',#27240,#21780,#21781);
#18280=AXIS2_PLACEMENT_3D('',#27386,#21783,#21784);
#18281=AXIS2_PLACEMENT_3D('',#27532,#21786,#21787);
#18282=AXIS2_PLACEMENT_3D('',#27678,#21789,#21790);
#18283=AXIS2_PLACEMENT_3D('',#27824,#21792,#21793);
#18284=AXIS2_PLACEMENT_3D('',#27970,#21795,#21796);
#18285=AXIS2_PLACEMENT_3D('',#28116,#21798,#21799);
#18286=AXIS2_PLACEMENT_3D('',#28262,#21801,#21802);
#18287=AXIS2_PLACEMENT_3D('',#28408,#21804,#21805);
#18288=AXIS2_PLACEMENT_3D('',#28554,#21807,#21808);
#18289=AXIS2_PLACEMENT_3D('',#28700,#21810,#21811);
#18290=AXIS2_PLACEMENT_3D('',#28846,#21813,#21814);
#18291=AXIS2_PLACEMENT_3D('',#28992,#21816,#21817);
#18292=AXIS2_PLACEMENT_3D('',#29138,#21819,#21820);
#18293=AXIS2_PLACEMENT_3D('',#29284,#21822,#21823);
#18294=AXIS2_PLACEMENT_3D('',#29430,#21825,#21826);
#18295=AXIS2_PLACEMENT_3D('',#29576,#21828,#21829);
#18296=AXIS2_PLACEMENT_3D('',#29720,#21831,#21832);
#18297=AXIS2_PLACEMENT_3D('',#29721,#21833,#21834);
#18298=AXIS2_PLACEMENT_3D('',#29722,#21835,#21836);
#18299=AXIS2_PLACEMENT_3D('',#29723,#21837,#21838);
#18300=AXIS2_PLACEMENT_3D('',#29725,#21839,#21840);
#18301=AXIS2_PLACEMENT_3D('',#29728,#21842,#21843);
#18302=AXIS2_PLACEMENT_3D('',#29729,#21844,#21845);
#18303=AXIS2_PLACEMENT_3D('',#29944,#21848,#21849);
#18304=AXIS2_PLACEMENT_3D('',#30160,#21853,#21854);
#18305=AXIS2_PLACEMENT_3D('',#30162,#21855,#21856);
#18306=AXIS2_PLACEMENT_3D('',#30376,#21859,#21860);
#18307=AXIS2_PLACEMENT_3D('',#30592,#21864,#21865);
#18308=AXIS2_PLACEMENT_3D('',#30594,#21866,#21867);
#18309=AXIS2_PLACEMENT_3D('',#30808,#21870,#21871);
#18310=AXIS2_PLACEMENT_3D('',#31024,#21875,#21876);
#18311=AXIS2_PLACEMENT_3D('',#31026,#21877,#21878);
#18312=AXIS2_PLACEMENT_3D('',#31240,#21881,#21882);
#18313=AXIS2_PLACEMENT_3D('',#31456,#21886,#21887);
#18314=AXIS2_PLACEMENT_3D('',#31458,#21888,#21889);
#18315=AXIS2_PLACEMENT_3D('',#31672,#21892,#21893);
#18316=AXIS2_PLACEMENT_3D('',#31888,#21897,#21898);
#18317=AXIS2_PLACEMENT_3D('',#31890,#21899,#21900);
#18318=AXIS2_PLACEMENT_3D('',#32104,#21903,#21904);
#18319=AXIS2_PLACEMENT_3D('',#32320,#21908,#21909);
#18320=AXIS2_PLACEMENT_3D('',#32322,#21910,#21911);
#18321=AXIS2_PLACEMENT_3D('',#32536,#21914,#21915);
#18322=AXIS2_PLACEMENT_3D('',#32752,#21919,#21920);
#18323=AXIS2_PLACEMENT_3D('',#32754,#21921,#21922);
#18324=AXIS2_PLACEMENT_3D('',#32968,#21925,#21926);
#18325=AXIS2_PLACEMENT_3D('',#33184,#21930,#21931);
#18326=AXIS2_PLACEMENT_3D('',#33186,#21932,#21933);
#18327=AXIS2_PLACEMENT_3D('',#33400,#21936,#21937);
#18328=AXIS2_PLACEMENT_3D('',#33616,#21941,#21942);
#18329=AXIS2_PLACEMENT_3D('',#33618,#21943,#21944);
#18330=AXIS2_PLACEMENT_3D('',#33832,#21947,#21948);
#18331=AXIS2_PLACEMENT_3D('',#34048,#21952,#21953);
#18332=AXIS2_PLACEMENT_3D('',#34050,#21954,#21955);
#18333=AXIS2_PLACEMENT_3D('',#34264,#21958,#21959);
#18334=AXIS2_PLACEMENT_3D('',#34480,#21963,#21964);
#18335=AXIS2_PLACEMENT_3D('',#34482,#21965,#21966);
#18336=AXIS2_PLACEMENT_3D('',#34696,#21969,#21970);
#18337=AXIS2_PLACEMENT_3D('',#34912,#21974,#21975);
#18338=AXIS2_PLACEMENT_3D('',#34914,#21976,#21977);
#18339=AXIS2_PLACEMENT_3D('',#35128,#21980,#21981);
#18340=AXIS2_PLACEMENT_3D('',#35344,#21985,#21986);
#18341=AXIS2_PLACEMENT_3D('',#35346,#21987,#21988);
#18342=AXIS2_PLACEMENT_3D('',#35560,#21991,#21992);
#18343=AXIS2_PLACEMENT_3D('',#35776,#21996,#21997);
#18344=AXIS2_PLACEMENT_3D('',#35778,#21998,#21999);
#18345=AXIS2_PLACEMENT_3D('',#35992,#22002,#22003);
#18346=AXIS2_PLACEMENT_3D('',#36208,#22007,#22008);
#18347=AXIS2_PLACEMENT_3D('',#36210,#22009,#22010);
#18348=AXIS2_PLACEMENT_3D('',#36424,#22013,#22014);
#18349=AXIS2_PLACEMENT_3D('',#36640,#22018,#22019);
#18350=AXIS2_PLACEMENT_3D('',#36642,#22020,#22021);
#18351=AXIS2_PLACEMENT_3D('',#36856,#22024,#22025);
#18352=AXIS2_PLACEMENT_3D('',#37072,#22029,#22030);
#18353=AXIS2_PLACEMENT_3D('',#37074,#22031,#22032);
#18354=AXIS2_PLACEMENT_3D('',#37288,#22035,#22036);
#18355=AXIS2_PLACEMENT_3D('',#37504,#22040,#22041);
#18356=AXIS2_PLACEMENT_3D('',#37506,#22042,#22043);
#18357=AXIS2_PLACEMENT_3D('',#37720,#22046,#22047);
#18358=AXIS2_PLACEMENT_3D('',#37936,#22051,#22052);
#18359=AXIS2_PLACEMENT_3D('',#37938,#22053,#22054);
#18360=AXIS2_PLACEMENT_3D('',#38152,#22057,#22058);
#18361=AXIS2_PLACEMENT_3D('',#38368,#22062,#22063);
#18362=AXIS2_PLACEMENT_3D('',#38369,#22064,#22065);
#18363=AXIS2_PLACEMENT_3D('',#38370,#22066,#22067);
#21751=DIRECTION('axis',(0.,0.,1.));
#21752=DIRECTION('refdir',(1.,0.,0.));
#21753=DIRECTION('center_axis',(1.,0.,0.));
#21754=DIRECTION('ref_axis',(0.,0.,-1.));
#21755=DIRECTION('',(0.,0.,1.));
#21756=DIRECTION('',(0.,1.,0.));
#21757=DIRECTION('',(0.,0.,-1.));
#21758=DIRECTION('',(0.,-1.,0.));
#21759=DIRECTION('center_axis',(0.,0.,-1.));
#21760=DIRECTION('ref_axis',(-1.,0.,0.));
#21761=DIRECTION('',(1.,0.,0.));
#21762=DIRECTION('',(0.,-1.,0.));
#21763=DIRECTION('',(-1.,0.,0.));
#21764=DIRECTION('center_axis',(-1.,0.,0.));
#21765=DIRECTION('ref_axis',(0.,0.,1.));
#21766=DIRECTION('',(0.,0.,-1.));
#21767=DIRECTION('',(0.,1.,0.));
#21768=DIRECTION('',(0.,0.,1.));
#21769=DIRECTION('center_axis',(0.,1.,0.));
#21770=DIRECTION('ref_axis',(1.,0.,0.));
#21771=DIRECTION('center_axis',(0.,-1.,0.));
#21772=DIRECTION('ref_axis',(1.,0.,0.));
#21773=DIRECTION('',(-0.587785252292473,0.,0.809016994374947));
#21774=DIRECTION('center_axis',(0.,-1.,0.));
#21775=DIRECTION('ref_axis',(1.,0.,0.));
#21776=DIRECTION('',(-0.809016994374948,0.,0.587785252292473));
#21777=DIRECTION('center_axis',(0.,-1.,0.));
#21778=DIRECTION('ref_axis',(1.,0.,0.));
#21779=DIRECTION('',(-0.951056516295154,0.,0.309016994374947));
#21780=DIRECTION('center_axis',(0.,-1.,0.));
#21781=DIRECTION('ref_axis',(1.,0.,0.));
#21782=DIRECTION('',(-1.,0.,-1.83697019872103E-16));
#21783=DIRECTION('center_axis',(0.,-1.,0.));
#21784=DIRECTION('ref_axis',(1.,0.,0.));
#21785=DIRECTION('',(-0.951056516295154,0.,-0.309016994374948));
#21786=DIRECTION('center_axis',(0.,-1.,0.));
#21787=DIRECTION('ref_axis',(1.,0.,0.));
#21788=DIRECTION('',(-0.809016994374947,0.,-0.587785252292473));
#21789=DIRECTION('center_axis',(0.,-1.,0.));
#21790=DIRECTION('ref_axis',(1.,0.,0.));
#21791=DIRECTION('',(-0.587785252292473,0.,-0.809016994374948));
#21792=DIRECTION('center_axis',(0.,-1.,0.));
#21793=DIRECTION('ref_axis',(1.,0.,0.));
#21794=DIRECTION('',(-0.309016994374947,0.,-0.951056516295154));
#21795=DIRECTION('center_axis',(0.,-1.,0.));
#21796=DIRECTION('ref_axis',(1.,0.,0.));
#21797=DIRECTION('',(1.22464679914735E-16,0.,-1.));
#21798=DIRECTION('center_axis',(0.,-1.,0.));
#21799=DIRECTION('ref_axis',(1.,0.,0.));
#21800=DIRECTION('',(0.309016994374948,0.,-0.951056516295154));
#21801=DIRECTION('center_axis',(0.,-1.,0.));
#21802=DIRECTION('ref_axis',(1.,0.,0.));
#21803=DIRECTION('',(0.587785252292473,0.,-0.809016994374947));
#21804=DIRECTION('center_axis',(0.,-1.,0.));
#21805=DIRECTION('ref_axis',(1.,0.,0.));
#21806=DIRECTION('',(0.809016994374948,0.,-0.587785252292473));
#21807=DIRECTION('center_axis',(0.,-1.,0.));
#21808=DIRECTION('ref_axis',(1.,0.,0.));
#21809=DIRECTION('',(0.951056516295154,0.,-0.309016994374947));
#21810=DIRECTION('center_axis',(0.,-1.,0.));
#21811=DIRECTION('ref_axis',(1.,0.,0.));
#21812=DIRECTION('',(1.,0.,6.12323399573677E-17));
#21813=DIRECTION('center_axis',(0.,-1.,0.));
#21814=DIRECTION('ref_axis',(1.,0.,0.));
#21815=DIRECTION('',(0.951056516295154,0.,0.309016994374948));
#21816=DIRECTION('center_axis',(0.,-1.,0.));
#21817=DIRECTION('ref_axis',(1.,0.,0.));
#21818=DIRECTION('',(0.809016994374947,0.,0.587785252292473));
#21819=DIRECTION('center_axis',(0.,-1.,0.));
#21820=DIRECTION('ref_axis',(1.,0.,0.));
#21821=DIRECTION('',(0.587785252292473,0.,0.809016994374947));
#21822=DIRECTION('center_axis',(0.,-1.,0.));
#21823=DIRECTION('ref_axis',(1.,0.,0.));
#21824=DIRECTION('',(0.309016994374947,0.,0.951056516295154));
#21825=DIRECTION('center_axis',(0.,-1.,0.));
#21826=DIRECTION('ref_axis',(1.,0.,0.));
#21827=DIRECTION('',(0.,0.,1.));
#21828=DIRECTION('center_axis',(0.,-1.,0.));
#21829=DIRECTION('ref_axis',(1.,0.,0.));
#21830=DIRECTION('',(-0.309016994374948,0.,0.951056516295154));
#21831=DIRECTION('center_axis',(0.,1.,0.));
#21832=DIRECTION('ref_axis',(1.,0.,0.));
#21833=DIRECTION('center_axis',(0.,1.,0.));
#21834=DIRECTION('ref_axis',(6.12323399573677E-17,0.,1.));
#21835=DIRECTION('center_axis',(0.,-1.,0.));
#21836=DIRECTION('ref_axis',(1.,0.,0.));
#21837=DIRECTION('center_axis',(0.,1.,0.));
#21838=DIRECTION('ref_axis',(1.,0.,0.));
#21839=DIRECTION('center_axis',(0.,1.,0.));
#21840=DIRECTION('ref_axis',(1.,0.,0.));
#21841=DIRECTION('',(0.,-1.,0.));
#21842=DIRECTION('center_axis',(0.,-1.,0.));
#21843=DIRECTION('ref_axis',(1.,0.,0.));
#21844=DIRECTION('center_axis',(0.,1.,0.));
#21845=DIRECTION('ref_axis',(1.,0.,0.));
#21846=DIRECTION('',(0.,-1.,0.));
#21847=DIRECTION('',(0.,1.,0.));
#21848=DIRECTION('center_axis',(0.951056516295154,0.,0.309016994374948));
#21849=DIRECTION('ref_axis',(0.309016994374948,0.,-0.951056516295154));
#21850=DIRECTION('',(0.309016994374948,0.,-0.951056516295154));
#21851=DIRECTION('',(0.,1.,0.));
#21852=DIRECTION('',(0.,1.,0.));
#21853=DIRECTION('center_axis',(0.,1.,0.));
#21854=DIRECTION('ref_axis',(1.,0.,0.));
#21855=DIRECTION('center_axis',(0.,1.,0.));
#21856=DIRECTION('ref_axis',(1.,0.,0.));
#21857=DIRECTION('',(0.,-1.,0.));
#21858=DIRECTION('',(0.,1.,0.));
#21859=DIRECTION('center_axis',(0.809016994374947,0.,0.587785252292473));
#21860=DIRECTION('ref_axis',(0.587785252292473,0.,-0.809016994374947));
#21861=DIRECTION('',(0.587785252292473,0.,-0.809016994374947));
#21862=DIRECTION('',(0.,1.,0.));
#21863=DIRECTION('',(0.,1.,0.));
#21864=DIRECTION('center_axis',(0.,1.,0.));
#21865=DIRECTION('ref_axis',(1.,0.,0.));
#21866=DIRECTION('center_axis',(0.,1.,0.));
#21867=DIRECTION('ref_axis',(1.,0.,0.));
#21868=DIRECTION('',(0.,-1.,0.));
#21869=DIRECTION('',(0.,1.,0.));
#21870=DIRECTION('center_axis',(0.587785252292473,0.,0.809016994374948));
#21871=DIRECTION('ref_axis',(0.809016994374948,0.,-0.587785252292473));
#21872=DIRECTION('',(0.809016994374948,0.,-0.587785252292473));
#21873=DIRECTION('',(0.,1.,0.));
#21874=DIRECTION('',(0.,1.,0.));
#21875=DIRECTION('center_axis',(0.,1.,0.));
#21876=DIRECTION('ref_axis',(1.,0.,0.));
#21877=DIRECTION('center_axis',(0.,1.,0.));
#21878=DIRECTION('ref_axis',(1.,0.,0.));
#21879=DIRECTION('',(0.,-1.,0.));
#21880=DIRECTION('',(0.,1.,0.));
#21881=DIRECTION('center_axis',(0.309016994374947,0.,0.951056516295154));
#21882=DIRECTION('ref_axis',(0.951056516295154,0.,-0.309016994374947));
#21883=DIRECTION('',(0.951056516295154,0.,-0.309016994374947));
#21884=DIRECTION('',(0.,1.,0.));
#21885=DIRECTION('',(0.,1.,0.));
#21886=DIRECTION('center_axis',(0.,1.,0.));
#21887=DIRECTION('ref_axis',(1.,0.,0.));
#21888=DIRECTION('center_axis',(0.,1.,0.));
#21889=DIRECTION('ref_axis',(1.,0.,0.));
#21890=DIRECTION('',(0.,-1.,0.));
#21891=DIRECTION('',(0.,1.,0.));
#21892=DIRECTION('center_axis',(-1.83697019872103E-16,0.,1.));
#21893=DIRECTION('ref_axis',(1.,0.,1.83697019872103E-16));
#21894=DIRECTION('',(1.,0.,1.83697019872103E-16));
#21895=DIRECTION('',(0.,1.,0.));
#21896=DIRECTION('',(0.,1.,0.));
#21897=DIRECTION('center_axis',(0.,1.,0.));
#21898=DIRECTION('ref_axis',(1.,0.,0.));
#21899=DIRECTION('center_axis',(0.,1.,0.));
#21900=DIRECTION('ref_axis',(1.,0.,0.));
#21901=DIRECTION('',(0.,-1.,0.));
#21902=DIRECTION('',(0.,1.,0.));
#21903=DIRECTION('center_axis',(-0.309016994374948,0.,0.951056516295154));
#21904=DIRECTION('ref_axis',(0.951056516295154,0.,0.309016994374948));
#21905=DIRECTION('',(0.951056516295154,0.,0.309016994374948));
#21906=DIRECTION('',(0.,1.,0.));
#21907=DIRECTION('',(0.,1.,0.));
#21908=DIRECTION('center_axis',(0.,1.,0.));
#21909=DIRECTION('ref_axis',(1.,0.,0.));
#21910=DIRECTION('center_axis',(0.,1.,0.));
#21911=DIRECTION('ref_axis',(1.,0.,0.));
#21912=DIRECTION('',(0.,-1.,0.));
#21913=DIRECTION('',(0.,1.,0.));
#21914=DIRECTION('center_axis',(-0.587785252292473,0.,0.809016994374947));
#21915=DIRECTION('ref_axis',(0.809016994374947,0.,0.587785252292473));
#21916=DIRECTION('',(0.809016994374947,0.,0.587785252292473));
#21917=DIRECTION('',(0.,1.,0.));
#21918=DIRECTION('',(0.,1.,0.));
#21919=DIRECTION('center_axis',(0.,1.,0.));
#21920=DIRECTION('ref_axis',(1.,0.,0.));
#21921=DIRECTION('center_axis',(0.,1.,0.));
#21922=DIRECTION('ref_axis',(1.,0.,0.));
#21923=DIRECTION('',(0.,-1.,0.));
#21924=DIRECTION('',(0.,1.,0.));
#21925=DIRECTION('center_axis',(-0.809016994374948,0.,0.587785252292473));
#21926=DIRECTION('ref_axis',(0.587785252292473,0.,0.809016994374948));
#21927=DIRECTION('',(0.587785252292473,0.,0.809016994374948));
#21928=DIRECTION('',(0.,1.,0.));
#21929=DIRECTION('',(0.,1.,0.));
#21930=DIRECTION('center_axis',(0.,1.,0.));
#21931=DIRECTION('ref_axis',(1.,0.,0.));
#21932=DIRECTION('center_axis',(0.,1.,0.));
#21933=DIRECTION('ref_axis',(1.,0.,0.));
#21934=DIRECTION('',(0.,-1.,0.));
#21935=DIRECTION('',(0.,1.,0.));
#21936=DIRECTION('center_axis',(-0.951056516295154,0.,0.309016994374947));
#21937=DIRECTION('ref_axis',(0.309016994374947,0.,0.951056516295154));
#21938=DIRECTION('',(0.309016994374947,0.,0.951056516295154));
#21939=DIRECTION('',(0.,1.,0.));
#21940=DIRECTION('',(0.,1.,0.));
#21941=DIRECTION('center_axis',(0.,1.,0.));
#21942=DIRECTION('ref_axis',(1.,0.,0.));
#21943=DIRECTION('center_axis',(0.,1.,0.));
#21944=DIRECTION('ref_axis',(1.,0.,0.));
#21945=DIRECTION('',(0.,-1.,0.));
#21946=DIRECTION('',(0.,1.,0.));
#21947=DIRECTION('center_axis',(-1.,0.,-1.22464679914735E-16));
#21948=DIRECTION('ref_axis',(-1.22464679914735E-16,0.,1.));
#21949=DIRECTION('',(-1.22464679914735E-16,0.,1.));
#21950=DIRECTION('',(0.,1.,0.));
#21951=DIRECTION('',(0.,1.,0.));
#21952=DIRECTION('center_axis',(0.,1.,0.));
#21953=DIRECTION('ref_axis',(1.,0.,0.));
#21954=DIRECTION('center_axis',(0.,1.,0.));
#21955=DIRECTION('ref_axis',(1.,0.,0.));
#21956=DIRECTION('',(0.,-1.,0.));
#21957=DIRECTION('',(0.,1.,0.));
#21958=DIRECTION('center_axis',(-0.951056516295154,0.,-0.309016994374948));
#21959=DIRECTION('ref_axis',(-0.309016994374948,0.,0.951056516295154));
#21960=DIRECTION('',(-0.309016994374948,0.,0.951056516295154));
#21961=DIRECTION('',(0.,1.,0.));
#21962=DIRECTION('',(0.,1.,0.));
#21963=DIRECTION('center_axis',(0.,1.,0.));
#21964=DIRECTION('ref_axis',(1.,0.,0.));
#21965=DIRECTION('center_axis',(0.,1.,0.));
#21966=DIRECTION('ref_axis',(1.,0.,0.));
#21967=DIRECTION('',(0.,-1.,0.));
#21968=DIRECTION('',(0.,1.,0.));
#21969=DIRECTION('center_axis',(-0.809016994374947,0.,-0.587785252292473));
#21970=DIRECTION('ref_axis',(-0.587785252292473,0.,0.809016994374947));
#21971=DIRECTION('',(-0.587785252292473,0.,0.809016994374947));
#21972=DIRECTION('',(0.,1.,0.));
#21973=DIRECTION('',(0.,1.,0.));
#21974=DIRECTION('center_axis',(0.,1.,0.));
#21975=DIRECTION('ref_axis',(1.,0.,0.));
#21976=DIRECTION('center_axis',(0.,1.,0.));
#21977=DIRECTION('ref_axis',(1.,0.,0.));
#21978=DIRECTION('',(0.,-1.,0.));
#21979=DIRECTION('',(0.,1.,0.));
#21980=DIRECTION('center_axis',(-0.587785252292473,0.,-0.809016994374948));
#21981=DIRECTION('ref_axis',(-0.809016994374948,0.,0.587785252292473));
#21982=DIRECTION('',(-0.809016994374948,0.,0.587785252292473));
#21983=DIRECTION('',(0.,1.,0.));
#21984=DIRECTION('',(0.,1.,0.));
#21985=DIRECTION('center_axis',(0.,1.,0.));
#21986=DIRECTION('ref_axis',(1.,0.,0.));
#21987=DIRECTION('center_axis',(0.,1.,0.));
#21988=DIRECTION('ref_axis',(1.,0.,0.));
#21989=DIRECTION('',(0.,-1.,0.));
#21990=DIRECTION('',(0.,1.,0.));
#21991=DIRECTION('center_axis',(-0.309016994374947,0.,-0.951056516295154));
#21992=DIRECTION('ref_axis',(-0.951056516295154,0.,0.309016994374947));
#21993=DIRECTION('',(-0.951056516295154,0.,0.309016994374947));
#21994=DIRECTION('',(0.,1.,0.));
#21995=DIRECTION('',(0.,1.,0.));
#21996=DIRECTION('center_axis',(0.,1.,0.));
#21997=DIRECTION('ref_axis',(1.,0.,0.));
#21998=DIRECTION('center_axis',(0.,1.,0.));
#21999=DIRECTION('ref_axis',(1.,0.,0.));
#22000=DIRECTION('',(0.,-1.,0.));
#22001=DIRECTION('',(0.,1.,0.));
#22002=DIRECTION('center_axis',(6.12323399573677E-17,0.,-1.));
#22003=DIRECTION('ref_axis',(-1.,0.,-6.12323399573677E-17));
#22004=DIRECTION('',(-1.,0.,-6.12323399573677E-17));
#22005=DIRECTION('',(0.,1.,0.));
#22006=DIRECTION('',(0.,1.,0.));
#22007=DIRECTION('center_axis',(0.,1.,0.));
#22008=DIRECTION('ref_axis',(1.,0.,0.));
#22009=DIRECTION('center_axis',(0.,1.,0.));
#22010=DIRECTION('ref_axis',(1.,0.,0.));
#22011=DIRECTION('',(0.,-1.,0.));
#22012=DIRECTION('',(0.,1.,0.));
#22013=DIRECTION('center_axis',(0.309016994374948,0.,-0.951056516295154));
#22014=DIRECTION('ref_axis',(-0.951056516295154,0.,-0.309016994374948));
#22015=DIRECTION('',(-0.951056516295154,0.,-0.309016994374948));
#22016=DIRECTION('',(0.,1.,0.));
#22017=DIRECTION('',(0.,1.,0.));
#22018=DIRECTION('center_axis',(0.,1.,0.));
#22019=DIRECTION('ref_axis',(1.,0.,0.));
#22020=DIRECTION('center_axis',(0.,1.,0.));
#22021=DIRECTION('ref_axis',(1.,0.,0.));
#22022=DIRECTION('',(0.,-1.,0.));
#22023=DIRECTION('',(0.,1.,0.));
#22024=DIRECTION('center_axis',(0.587785252292473,0.,-0.809016994374947));
#22025=DIRECTION('ref_axis',(-0.809016994374947,0.,-0.587785252292473));
#22026=DIRECTION('',(-0.809016994374947,0.,-0.587785252292473));
#22027=DIRECTION('',(0.,1.,0.));
#22028=DIRECTION('',(0.,1.,0.));
#22029=DIRECTION('center_axis',(0.,1.,0.));
#22030=DIRECTION('ref_axis',(1.,0.,0.));
#22031=DIRECTION('center_axis',(0.,1.,0.));
#22032=DIRECTION('ref_axis',(1.,0.,0.));
#22033=DIRECTION('',(0.,-1.,0.));
#22034=DIRECTION('',(0.,1.,0.));
#22035=DIRECTION('center_axis',(0.809016994374947,0.,-0.587785252292473));
#22036=DIRECTION('ref_axis',(-0.587785252292473,0.,-0.809016994374947));
#22037=DIRECTION('',(-0.587785252292473,0.,-0.809016994374947));
#22038=DIRECTION('',(0.,1.,0.));
#22039=DIRECTION('',(0.,1.,0.));
#22040=DIRECTION('center_axis',(0.,1.,0.));
#22041=DIRECTION('ref_axis',(1.,0.,0.));
#22042=DIRECTION('center_axis',(0.,1.,0.));
#22043=DIRECTION('ref_axis',(1.,0.,0.));
#22044=DIRECTION('',(0.,-1.,0.));
#22045=DIRECTION('',(0.,1.,0.));
#22046=DIRECTION('center_axis',(0.951056516295154,0.,-0.309016994374947));
#22047=DIRECTION('ref_axis',(-0.309016994374947,0.,-0.951056516295154));
#22048=DIRECTION('',(-0.309016994374947,0.,-0.951056516295154));
#22049=DIRECTION('',(0.,1.,0.));
#22050=DIRECTION('',(0.,1.,0.));
#22051=DIRECTION('center_axis',(0.,1.,0.));
#22052=DIRECTION('ref_axis',(1.,0.,0.));
#22053=DIRECTION('center_axis',(0.,1.,0.));
#22054=DIRECTION('ref_axis',(1.,0.,0.));
#22055=DIRECTION('',(0.,-1.,0.));
#22056=DIRECTION('',(0.,1.,0.));
#22057=DIRECTION('center_axis',(1.,0.,0.));
#22058=DIRECTION('ref_axis',(0.,0.,-1.));
#22059=DIRECTION('',(0.,0.,-1.));
#22060=DIRECTION('',(0.,1.,0.));
#22061=DIRECTION('',(0.,1.,0.));
#22062=DIRECTION('center_axis',(0.,1.,0.));
#22063=DIRECTION('ref_axis',(1.,0.,0.));
#22064=DIRECTION('center_axis',(0.,1.,0.));
#22065=DIRECTION('ref_axis',(1.,0.,0.));
#22066=DIRECTION('center_axis',(0.,1.,0.));
#22067=DIRECTION('ref_axis',(1.,0.,0.));
#26777=CARTESIAN_POINT('',(0.,0.,0.));
#26778=CARTESIAN_POINT('Origin',(0.2,0.,0.));
#26779=CARTESIAN_POINT('',(0.2,2.2,-0.78));
#26780=CARTESIAN_POINT('',(0.2,2.2,-0.565685424949238));
#26781=CARTESIAN_POINT('',(0.2,2.2,0.));
#26782=CARTESIAN_POINT('',(0.2,-1.,-0.78));
#26783=CARTESIAN_POINT('',(0.2,0.,-0.78));
#26784=CARTESIAN_POINT('',(0.2,-1.,-0.565685424949238));
#26785=CARTESIAN_POINT('',(0.2,-1.,0.));
#26786=CARTESIAN_POINT('',(0.2,0.,-0.565685424949238));
#26787=CARTESIAN_POINT('Origin',(0.2,0.,-0.78));
#26788=CARTESIAN_POINT('',(-0.2,2.2,-0.78));
#26789=CARTESIAN_POINT('',(0.1,2.2,-0.78));
#26790=CARTESIAN_POINT('',(-0.2,-1.,-0.78));
#26791=CARTESIAN_POINT('',(-0.2,0.,-0.78));
#26792=CARTESIAN_POINT('',(0.1,-1.,-0.78));
#26793=CARTESIAN_POINT('Origin',(-0.2,0.,-0.78));
#26794=CARTESIAN_POINT('',(-0.2,2.2,-0.565685424949238));
#26795=CARTESIAN_POINT('',(-0.2,2.2,-0.39));
#26796=CARTESIAN_POINT('',(-0.2,-1.,-0.565685424949238));
#26797=CARTESIAN_POINT('',(-0.2,0.,-0.565685424949238));
#26798=CARTESIAN_POINT('',(-0.2,-1.,-0.39));
#26799=CARTESIAN_POINT('Origin',(0.,-1.,0.));
#26800=CARTESIAN_POINT('',(1.60662857109684,-1.,0.693717979106306));
#26801=CARTESIAN_POINT('',(1.5055822144029,-1.,0.892032620296856));
#26802=CARTESIAN_POINT('Origin',(0.,-1.,0.));
#26803=CARTESIAN_POINT('',(1.81978687191668,-1.,1.23627494547115));
#26804=CARTESIAN_POINT('Ctrl Pts',(1.5055822144029,-1.,0.892032620296856));
#26805=CARTESIAN_POINT('Ctrl Pts',(1.50980486806688,-1.,0.894452006964544));
#26806=CARTESIAN_POINT('Ctrl Pts',(1.51805569590094,-1.,0.899185047483511));
#26807=CARTESIAN_POINT('Ctrl Pts',(1.52984849887993,-1.,0.905967409625651));
#26808=CARTESIAN_POINT('Ctrl Pts',(1.54440491149498,-1.,0.914375919026456));
#26809=CARTESIAN_POINT('Ctrl Pts',(1.56065988578893,-1.,0.923832188944341));
#26810=CARTESIAN_POINT('Ctrl Pts',(1.57499388382243,-1.,0.932246680108685));
#26811=CARTESIAN_POINT('Ctrl Pts',(1.58744937487176,-1.,0.939646377893399));
#26812=CARTESIAN_POINT('Ctrl Pts',(1.59810042043673,-1.,0.946078063315257));
#26813=CARTESIAN_POINT('Ctrl Pts',(1.60706069896936,-1.,0.951613284356035));
#26814=CARTESIAN_POINT('Ctrl Pts',(1.61449324337085,-1.,0.956354422920671));
#26815=CARTESIAN_POINT('Ctrl Pts',(1.62061638140221,-1.,0.960438326101729));
#26816=CARTESIAN_POINT('Ctrl Pts',(1.62571930670187,-1.,0.964046107040536));
#26817=CARTESIAN_POINT('Ctrl Pts',(1.63013849959461,-1.,0.967387853230345));
#26818=CARTESIAN_POINT('Ctrl Pts',(1.63420665729798,-1.,0.970669715997509));
#26819=CARTESIAN_POINT('Ctrl Pts',(1.63820952658144,-1.,0.974066058287419));
#26820=CARTESIAN_POINT('Ctrl Pts',(1.64233990826687,-1.,0.977689794119417));
#26821=CARTESIAN_POINT('Ctrl Pts',(1.64665139190656,-1.,0.981562530939489));
#26822=CARTESIAN_POINT('Ctrl Pts',(1.65110016612638,-1.,0.985642622920821));
#26823=CARTESIAN_POINT('Ctrl Pts',(1.65559044289699,-1.,0.989855627854165));
#26824=CARTESIAN_POINT('Ctrl Pts',(1.66001553809947,-1.,0.994121836661306));
#26825=CARTESIAN_POINT('Ctrl Pts',(1.66430758030376,-1.,0.998389654952758));
#26826=CARTESIAN_POINT('Ctrl Pts',(1.66846059277303,-1.,1.00265091003727));
#26827=CARTESIAN_POINT('Ctrl Pts',(1.67250335383293,-1.,1.00692206696414));
#26828=CARTESIAN_POINT('Ctrl Pts',(1.67648246776464,-1.,1.01123236493511));
#26829=CARTESIAN_POINT('Ctrl Pts',(1.68044289894798,-1.,1.01561026162773));
#26830=CARTESIAN_POINT('Ctrl Pts',(1.68440578021706,-1.,1.02006795074201));
#26831=CARTESIAN_POINT('Ctrl Pts',(1.68836910178447,-1.,1.02460180535255));
#26832=CARTESIAN_POINT('Ctrl Pts',(1.69231840863458,-1.,1.02919977579147));
#26833=CARTESIAN_POINT('Ctrl Pts',(1.69623414782771,-1.,1.03384646003588));
#26834=CARTESIAN_POINT('Ctrl Pts',(1.70010052930962,-1.,1.03852922490789));
#26835=CARTESIAN_POINT('Ctrl Pts',(1.70391338707982,-1.,1.04324363334554));
#26836=CARTESIAN_POINT('Ctrl Pts',(1.70767646263649,-1.,1.04799085404995));
#26837=CARTESIAN_POINT('Ctrl Pts',(1.71139783543989,-1.,1.05277517202855));
#26838=CARTESIAN_POINT('Ctrl Pts',(1.7150865442702,-1.,1.05760163192479));
#26839=CARTESIAN_POINT('Ctrl Pts',(1.71874858456904,-1.,1.06247324680647));
#26840=CARTESIAN_POINT('Ctrl Pts',(1.72238500928453,-1.,1.06738966975462));
#26841=CARTESIAN_POINT('Ctrl Pts',(1.72599406198488,-1.,1.07234866990252));
#26842=CARTESIAN_POINT('Ctrl Pts',(1.72957248977424,-1.,1.0773470373727));
#26843=CARTESIAN_POINT('Ctrl Pts',(1.73311705663407,-1.,1.08238162784749));
#26844=CARTESIAN_POINT('Ctrl Pts',(1.73662628326091,-1.,1.08745056285427));
#26845=CARTESIAN_POINT('Ctrl Pts',(1.74010053962247,-1.,1.09255329056493));
#26846=CARTESIAN_POINT('Ctrl Pts',(1.74354119236208,-1.,1.09768999241226));
#26847=CARTESIAN_POINT('Ctrl Pts',(1.74695004214923,-1.,1.10286118991143));
#26848=CARTESIAN_POINT('Ctrl Pts',(1.7503286607592,-1.,1.10806728183007));
#26849=CARTESIAN_POINT('Ctrl Pts',(1.7536777209463,-1.,1.11330807582551));
#26850=CARTESIAN_POINT('Ctrl Pts',(1.75699720772105,-1.,1.11858293216763));
#26851=CARTESIAN_POINT('Ctrl Pts',(1.76028671825096,-1.,1.12389096855086));
#26852=CARTESIAN_POINT('Ctrl Pts',(1.7635457196617,-1.,1.12923123555075));
#26853=CARTESIAN_POINT('Ctrl Pts',(1.76677384551862,-1.,1.1346029180462));
#26854=CARTESIAN_POINT('Ctrl Pts',(1.76997111386769,-1.,1.14000548336975));
#26855=CARTESIAN_POINT('Ctrl Pts',(1.77313777896194,-1.,1.1454385822692));
#26856=CARTESIAN_POINT('Ctrl Pts',(1.7762742255701,-1.,1.15090197841515));
#26857=CARTESIAN_POINT('Ctrl Pts',(1.77938085564275,-1.,1.15639547194698));
#26858=CARTESIAN_POINT('Ctrl Pts',(1.78245795881009,-1.,1.16191881298499));
#26859=CARTESIAN_POINT('Ctrl Pts',(1.78550566040443,-1.,1.16747166312303));
#26860=CARTESIAN_POINT('Ctrl Pts',(1.78852398877616,-1.,1.17305363177328));
#26861=CARTESIAN_POINT('Ctrl Pts',(1.79151291552689,-1.,1.17866429440809));
#26862=CARTESIAN_POINT('Ctrl Pts',(1.79447240321515,-1.,1.18430321697432));
#26863=CARTESIAN_POINT('Ctrl Pts',(1.79740245923478,-1.,1.18996997934445));
#26864=CARTESIAN_POINT('Ctrl Pts',(1.80030314369879,-1.,1.19566418930242));
#26865=CARTESIAN_POINT('Ctrl Pts',(1.80317454838603,-1.,1.20138548938974));
#26866=CARTESIAN_POINT('Ctrl Pts',(1.80601678480707,-1.,1.20713356605475));
#26867=CARTESIAN_POINT('Ctrl Pts',(1.80882996917129,-1.,1.21290815708314));
#26868=CARTESIAN_POINT('Ctrl Pts',(1.81161420806656,-1.,1.21870906103557));
#26869=CARTESIAN_POINT('Ctrl Pts',(1.81436959210434,-1.,1.2245361330495));
#26870=CARTESIAN_POINT('Ctrl Pts',(1.8165508718364,-1.,1.2292186489137));
#26871=CARTESIAN_POINT('Ctrl Pts',(1.81817389921279,-1.,1.2327422452705));
#26872=CARTESIAN_POINT('Ctrl Pts',(1.81925017193666,-1.,1.23509651170476));
#26873=CARTESIAN_POINT('Ctrl Pts',(1.81978687191668,-1.,1.23627494547115));
#26874=CARTESIAN_POINT('',(1.73811241238545,-1.,1.34869019493419));
#26875=CARTESIAN_POINT('',(1.81978687191668,-1.,1.23627494547115));
#26876=CARTESIAN_POINT('',(1.31362392696032,-1.,1.15624053661742));
#26877=CARTESIAN_POINT('Ctrl Pts',(1.73811241238545,-1.,1.34869019493419));
#26878=CARTESIAN_POINT('Ctrl Pts',(1.73682580585691,-1.,1.34854391898045));
#26879=CARTESIAN_POINT('Ctrl Pts',(1.73425417885907,-1.,1.34824783112887));
#26880=CARTESIAN_POINT('Ctrl Pts',(1.7304014965394,-1.,1.34779309152035));
#26881=CARTESIAN_POINT('Ctrl Pts',(1.72527410680674,-1.,1.34716554819527));
#26882=CARTESIAN_POINT('Ctrl Pts',(1.7188807715049,-1.,1.34634568653227));
#26883=CARTESIAN_POINT('Ctrl Pts',(1.71250340686822,-1.,1.34549029589416));
#26884=CARTESIAN_POINT('Ctrl Pts',(1.70614212266738,-1.,1.34459924533831));
#26885=CARTESIAN_POINT('Ctrl Pts',(1.69979707754427,-1.,1.34367237124483));
#26886=CARTESIAN_POINT('Ctrl Pts',(1.6934684849687,-1.,1.34270948206319));
#26887=CARTESIAN_POINT('Ctrl Pts',(1.68715660868764,-1.,1.341710374848));
#26888=CARTESIAN_POINT('Ctrl Pts',(1.68086176030362,-1.,1.34067485185203));
#26889=CARTESIAN_POINT('Ctrl Pts',(1.67458429426086,-1.,1.3396027347034));
#26890=CARTESIAN_POINT('Ctrl Pts',(1.66832460783989,-1.,1.33849388654388));
#26891=CARTESIAN_POINT('Ctrl Pts',(1.66208312541983,-1.,1.33734820885262));
#26892=CARTESIAN_POINT('Ctrl Pts',(1.65586025952593,-1.,1.33616559745172));
#26893=CARTESIAN_POINT('Ctrl Pts',(1.6496563728683,-1.,1.33494590467993));
#26894=CARTESIAN_POINT('Ctrl Pts',(1.6434717485603,-1.,1.33368890676572));
#26895=CARTESIAN_POINT('Ctrl Pts',(1.63730653475089,-1.,1.33239425103724));
#26896=CARTESIAN_POINT('Ctrl Pts',(1.63116079730923,-1.,1.33106149345645));
#26897=CARTESIAN_POINT('Ctrl Pts',(1.62503464209797,-1.,1.3296901950568));
#26898=CARTESIAN_POINT('Ctrl Pts',(1.61892832270724,-1.,1.32828000610449));
#26899=CARTESIAN_POINT('Ctrl Pts',(1.6128423401575,-1.,1.32683074483356));
#26900=CARTESIAN_POINT('Ctrl Pts',(1.60677758290954,-1.,1.32534250785782));
#26901=CARTESIAN_POINT('Ctrl Pts',(1.60073511858687,-1.,1.32381550858256));
#26902=CARTESIAN_POINT('Ctrl Pts',(1.59471591079403,-1.,1.32224985747682));
#26903=CARTESIAN_POINT('Ctrl Pts',(1.58872057258245,-1.,1.32064537110892));
#26904=CARTESIAN_POINT('Ctrl Pts',(1.58274907898834,-1.,1.31900135021432));
#26905=CARTESIAN_POINT('Ctrl Pts',(1.5768005650559,-1.,1.31731642317187));
#26906=CARTESIAN_POINT('Ctrl Pts',(1.57087397835723,-1.,1.31558903860016));
#26907=CARTESIAN_POINT('Ctrl Pts',(1.56496872402353,-1.,1.31381795281002));
#26908=CARTESIAN_POINT('Ctrl Pts',(1.55908521254821,-1.,1.31200264341696));
#26909=CARTESIAN_POINT('Ctrl Pts',(1.55322568759481,-1.,1.31014393684222));
#26910=CARTESIAN_POINT('Ctrl Pts',(1.54739413957185,-1.,1.30824393907473));
#26911=CARTESIAN_POINT('Ctrl Pts',(1.54159462645432,-1.,1.30630475189556));
#26912=CARTESIAN_POINT('Ctrl Pts',(1.53582981268977,-1.,1.30432735639489));
#26913=CARTESIAN_POINT('Ctrl Pts',(1.53009970283891,-1.,1.30231064395568));
#26914=CARTESIAN_POINT('Ctrl Pts',(1.52439957861062,-1.,1.30024984366328));
#26915=CARTESIAN_POINT('Ctrl Pts',(1.51872184912724,-1.,1.29813791800747));
#26916=CARTESIAN_POINT('Ctrl Pts',(1.51305994241402,-1.,1.29596850710509));
#26917=CARTESIAN_POINT('Ctrl Pts',(1.50741159078365,-1.,1.29373841372842));
#26918=CARTESIAN_POINT('Ctrl Pts',(1.50178230149776,-1.,1.29145022885181));
#26919=CARTESIAN_POINT('Ctrl Pts',(1.49618896881754,-1.,1.28911506584254));
#26920=CARTESIAN_POINT('Ctrl Pts',(1.4906522831278,-1.,1.2867467611644));
#26921=CARTESIAN_POINT('Ctrl Pts',(1.4851881711891,-1.,1.28435533880201));
#26922=CARTESIAN_POINT('Ctrl Pts',(1.47980070347095,-1.,1.28194158939517));
#26923=CARTESIAN_POINT('Ctrl Pts',(1.4744717526707,-1.,1.2794891824849));
#26924=CARTESIAN_POINT('Ctrl Pts',(1.46916035917133,-1.,1.2769641483109));
#26925=CARTESIAN_POINT('Ctrl Pts',(1.46382431332476,-1.,1.27433119897822));
#26926=CARTESIAN_POINT('Ctrl Pts',(1.45843906294697,-1.,1.27156805265289));
#26927=CARTESIAN_POINT('Ctrl Pts',(1.45301422764247,-1.,1.2686778680489));
#26928=CARTESIAN_POINT('Ctrl Pts',(1.44761985001662,-1.,1.26570925118868));
#26929=CARTESIAN_POINT('Ctrl Pts',(1.44236470511303,-1.,1.26273903323859));
#26930=CARTESIAN_POINT('Ctrl Pts',(1.43734919180847,-1.,1.25983531012005));
#26931=CARTESIAN_POINT('Ctrl Pts',(1.43262645609691,-1.,1.25702687965755));
#26932=CARTESIAN_POINT('Ctrl Pts',(1.42815938799387,-1.,1.25426945222639));
#26933=CARTESIAN_POINT('Ctrl Pts',(1.42378102115575,-1.,1.2514145557001));
#26934=CARTESIAN_POINT('Ctrl Pts',(1.41923722596025,-1.,1.24824430986571));
#26935=CARTESIAN_POINT('Ctrl Pts',(1.41422913175179,-1.,1.24450600513056));
#26936=CARTESIAN_POINT('Ctrl Pts',(1.40845295531283,-1.,1.23994455029534));
#26937=CARTESIAN_POINT('Ctrl Pts',(1.40164708206106,-1.,1.23434087290423));
#26938=CARTESIAN_POINT('Ctrl Pts',(1.39361389568796,-1.,1.22752961899387));
#26939=CARTESIAN_POINT('Ctrl Pts',(1.38420564527715,-1.,1.21938737280852));
#26940=CARTESIAN_POINT('Ctrl Pts',(1.37331915607905,-1.,1.20982812925645));
#26941=CARTESIAN_POINT('Ctrl Pts',(1.36088705043885,-1.,1.1987959077932));
#26942=CARTESIAN_POINT('Ctrl Pts',(1.34687054001093,-1.,1.18625865667441));
#26943=CARTESIAN_POINT('Ctrl Pts',(1.33437539347008,-1.,1.17501305789857));
#26944=CARTESIAN_POINT('Ctrl Pts',(1.32428080721772,-1.,1.16589330093588));
#26945=CARTESIAN_POINT('Ctrl Pts',(1.31722977216397,-1.,1.15950888730809));
#26946=CARTESIAN_POINT('Ctrl Pts',(1.31362392696032,-1.,1.15624053661742));
#26947=CARTESIAN_POINT('',(1.15624053661742,-1.,1.31362392696033));
#26948=CARTESIAN_POINT('Origin',(0.,-1.,0.));
#26949=CARTESIAN_POINT('',(1.34869019493419,-1.,1.73811241238545));
#26950=CARTESIAN_POINT('Ctrl Pts',(1.15624053661742,-1.,1.31362392696033));
#26951=CARTESIAN_POINT('Ctrl Pts',(1.15950888730433,-1.,1.3172297721596));
#26952=CARTESIAN_POINT('Ctrl Pts',(1.16589330092532,-1.,1.32428080720544));
#26953=CARTESIAN_POINT('Ctrl Pts',(1.17501305787994,-1.,1.33437539344842));
#26954=CARTESIAN_POINT('Ctrl Pts',(1.18625865664915,-1.,1.34687053998157));
#26955=CARTESIAN_POINT('Ctrl Pts',(1.1987959077656,-1.,1.36088705040677));
#26956=CARTESIAN_POINT('Ctrl Pts',(1.20982812923113,-1.,1.37331915604962));
#26957=CARTESIAN_POINT('Ctrl Pts',(1.21938737278853,-1.,1.38420564525391));
#26958=CARTESIAN_POINT('Ctrl Pts',(1.22752961898063,-1.,1.39361389567257));
#26959=CARTESIAN_POINT('Ctrl Pts',(1.23434087289768,-1.,1.40164708205345));
#26960=CARTESIAN_POINT('Ctrl Pts',(1.23994455029421,-1.,1.40845295531151));
#26961=CARTESIAN_POINT('Ctrl Pts',(1.24450600513278,-1.,1.41422913175437));
#26962=CARTESIAN_POINT('Ctrl Pts',(1.24824430986911,-1.,1.41923722596421));
#26963=CARTESIAN_POINT('Ctrl Pts',(1.25141455570299,-1.,1.42378102115911));
#26964=CARTESIAN_POINT('Ctrl Pts',(1.25426945222783,-1.,1.42815938799555));
#26965=CARTESIAN_POINT('Ctrl Pts',(1.25702687965744,-1.,1.43262645609679));
#26966=CARTESIAN_POINT('Ctrl Pts',(1.25983531011894,-1.,1.43734919180719));
#26967=CARTESIAN_POINT('Ctrl Pts',(1.26273903323723,-1.,1.44236470511145));
#26968=CARTESIAN_POINT('Ctrl Pts',(1.26570925118767,-1.,1.44761985001544));
#26969=CARTESIAN_POINT('Ctrl Pts',(1.26867786804854,-1.,1.45301422764205));
#26970=CARTESIAN_POINT('Ctrl Pts',(1.27156805265312,-1.,1.45843906294725));
#26971=CARTESIAN_POINT('Ctrl Pts',(1.27433119897877,-1.,1.4638243133254));
#26972=CARTESIAN_POINT('Ctrl Pts',(1.27696414831144,-1.,1.46916035917197));
#26973=CARTESIAN_POINT('Ctrl Pts',(1.27948918248524,-1.,1.4744717526711));
#26974=CARTESIAN_POINT('Ctrl Pts',(1.28194158939522,-1.,1.47980070347102));
#26975=CARTESIAN_POINT('Ctrl Pts',(1.28435533880184,-1.,1.48518817118891));
#26976=CARTESIAN_POINT('Ctrl Pts',(1.28674676116415,-1.,1.4906522831275));
#26977=CARTESIAN_POINT('Ctrl Pts',(1.28911506584232,-1.,1.49618896881729));
#26978=CARTESIAN_POINT('Ctrl Pts',(1.29145022885171,-1.,1.50178230149764));
#26979=CARTESIAN_POINT('Ctrl Pts',(1.29373841372843,-1.,1.50741159078367));
#26980=CARTESIAN_POINT('Ctrl Pts',(1.29596850710518,-1.,1.51305994241412));
#26981=CARTESIAN_POINT('Ctrl Pts',(1.29813791800757,-1.,1.51872184912735));
#26982=CARTESIAN_POINT('Ctrl Pts',(1.30024984366334,-1.,1.5243995786107));
#26983=CARTESIAN_POINT('Ctrl Pts',(1.3023106439557,-1.,1.53009970283893));
#26984=CARTESIAN_POINT('Ctrl Pts',(1.30432735639487,-1.,1.53582981268976));
#26985=CARTESIAN_POINT('Ctrl Pts',(1.30630475189553,-1.,1.54159462645428));
#26986=CARTESIAN_POINT('Ctrl Pts',(1.30824393907471,-1.,1.54739413957183));
#26987=CARTESIAN_POINT('Ctrl Pts',(1.31014393684221,-1.,1.55322568759481));
#26988=CARTESIAN_POINT('Ctrl Pts',(1.31200264341696,-1.,1.55908521254822));
#26989=CARTESIAN_POINT('Ctrl Pts',(1.31381795281002,-1.,1.56496872402352));
#26990=CARTESIAN_POINT('Ctrl Pts',(1.31558903860015,-1.,1.57087397835721));
#26991=CARTESIAN_POINT('Ctrl Pts',(1.31731642317183,-1.,1.57680056505585));
#26992=CARTESIAN_POINT('Ctrl Pts',(1.31900135021428,-1.,1.58274907898829));
#26993=CARTESIAN_POINT('Ctrl Pts',(1.32064537110891,-1.,1.58872057258244));
#26994=CARTESIAN_POINT('Ctrl Pts',(1.32224985747686,-1.,1.59471591079408));
#26995=CARTESIAN_POINT('Ctrl Pts',(1.32381550858266,-1.,1.600735118587));
#26996=CARTESIAN_POINT('Ctrl Pts',(1.32534250785794,-1.,1.6067775829097));
#26997=CARTESIAN_POINT('Ctrl Pts',(1.32683074483365,-1.,1.61284234015762));
#26998=CARTESIAN_POINT('Ctrl Pts',(1.32828000610448,-1.,1.61892832270723));
#26999=CARTESIAN_POINT('Ctrl Pts',(1.32969019505665,-1.,1.62503464209777));
#27000=CARTESIAN_POINT('Ctrl Pts',(1.33106149345618,-1.,1.63116079730887));
#27001=CARTESIAN_POINT('Ctrl Pts',(1.33239425103694,-1.,1.6373065347505));
#27002=CARTESIAN_POINT('Ctrl Pts',(1.33368890676554,-1.,1.64347174856007));
#27003=CARTESIAN_POINT('Ctrl Pts',(1.33494590468003,-1.,1.64965637286843));
#27004=CARTESIAN_POINT('Ctrl Pts',(1.33616559745217,-1.,1.65586025952651));
#27005=CARTESIAN_POINT('Ctrl Pts',(1.33734820885331,-1.,1.66208312542073));
#27006=CARTESIAN_POINT('Ctrl Pts',(1.33849388654458,-1.,1.66832460784078));
#27007=CARTESIAN_POINT('Ctrl Pts',(1.33960273470372,-1.,1.67458429426126));
#27008=CARTESIAN_POINT('Ctrl Pts',(1.3406748518516,-1.,1.68086176030308));
#27009=CARTESIAN_POINT('Ctrl Pts',(1.34171037484673,-1.,1.68715660868602));
#27010=CARTESIAN_POINT('Ctrl Pts',(1.34270948206139,-1.,1.6934684849664));
#27011=CARTESIAN_POINT('Ctrl Pts',(1.34367237124322,-1.,1.69979707754221));
#27012=CARTESIAN_POINT('Ctrl Pts',(1.34459924533783,-1.,1.70614212266676));
#27013=CARTESIAN_POINT('Ctrl Pts',(1.34549029589563,-1.,1.71250340687011));
#27014=CARTESIAN_POINT('Ctrl Pts',(1.34634568653586,-1.,1.7188807715095));
#27015=CARTESIAN_POINT('Ctrl Pts',(1.34716554820013,-1.,1.72527410681298));
#27016=CARTESIAN_POINT('Ctrl Pts',(1.3477930915247,-1.,1.73040149654497));
#27017=CARTESIAN_POINT('Ctrl Pts',(1.34824783113158,-1.,1.73425417886255));
#27018=CARTESIAN_POINT('Ctrl Pts',(1.34854391898145,-1.,1.73682580585819));
#27019=CARTESIAN_POINT('Ctrl Pts',(1.34869019493419,-1.,1.73811241238545));
#27020=CARTESIAN_POINT('',(1.23627494547115,-1.,1.81978687191668));
#27021=CARTESIAN_POINT('',(1.34869019493419,-1.,1.73811241238545));
#27022=CARTESIAN_POINT('',(0.892032620296855,-1.,1.5055822144029));
#27023=CARTESIAN_POINT('Ctrl Pts',(1.23627494547115,-1.,1.81978687191668));
#27024=CARTESIAN_POINT('Ctrl Pts',(1.23509651170384,-1.,1.81925017193531));
#27025=CARTESIAN_POINT('Ctrl Pts',(1.23274224526804,-1.,1.81817389920914));
#27026=CARTESIAN_POINT('Ctrl Pts',(1.22921864890975,-1.,1.81655087183054));
#27027=CARTESIAN_POINT('Ctrl Pts',(1.22453613304507,-1.,1.81436959209778));
#27028=CARTESIAN_POINT('Ctrl Pts',(1.2187090610323,-1.,1.81161420806172));
#27029=CARTESIAN_POINT('Ctrl Pts',(1.2129081570818,-1.,1.80882996916931));
#27030=CARTESIAN_POINT('Ctrl Pts',(1.20713356605519,-1.,1.80601678480772));
#27031=CARTESIAN_POINT('Ctrl Pts',(1.2013854893912,-1.,1.8031745483882));
#27032=CARTESIAN_POINT('Ctrl Pts',(1.19566418930405,-1.,1.80030314370121));
#27033=CARTESIAN_POINT('Ctrl Pts',(1.1899699793456,-1.,1.79740245923649));
#27034=CARTESIAN_POINT('Ctrl Pts',(1.18430321697471,-1.,1.79447240321572));
#27035=CARTESIAN_POINT('Ctrl Pts',(1.17866429440781,-1.,1.79151291552646));
#27036=CARTESIAN_POINT('Ctrl Pts',(1.17305363177265,-1.,1.78852398877523));
#27037=CARTESIAN_POINT('Ctrl Pts',(1.16747166312239,-1.,1.78550566040349));
#27038=CARTESIAN_POINT('Ctrl Pts',(1.16191881298458,-1.,1.78245795880949));
#27039=CARTESIAN_POINT('Ctrl Pts',(1.15639547194689,-1.,1.77938085564261));
#27040=CARTESIAN_POINT('Ctrl Pts',(1.15090197841531,-1.,1.77627422557034));
#27041=CARTESIAN_POINT('Ctrl Pts',(1.14543858226948,-1.,1.77313777896234));
#27042=CARTESIAN_POINT('Ctrl Pts',(1.14000548337,-1.,1.76997111386806));
#27043=CARTESIAN_POINT('Ctrl Pts',(1.13460291804634,-1.,1.76677384551883));
#27044=CARTESIAN_POINT('Ctrl Pts',(1.12923123555076,-1.,1.76354571966171));
#27045=CARTESIAN_POINT('Ctrl Pts',(1.12389096855078,-1.,1.76028671825084));
#27046=CARTESIAN_POINT('Ctrl Pts',(1.11858293216752,-1.,1.75699720772089));
#27047=CARTESIAN_POINT('Ctrl Pts',(1.11330807582542,-1.,1.75367772094617));
#27048=CARTESIAN_POINT('Ctrl Pts',(1.10806728183003,-1.,1.75032866075914));
#27049=CARTESIAN_POINT('Ctrl Pts',(1.10286118991144,-1.,1.74695004214924));
#27050=CARTESIAN_POINT('Ctrl Pts',(1.09768999241229,-1.,1.74354119236212));
#27051=CARTESIAN_POINT('Ctrl Pts',(1.09255329056496,-1.,1.74010053962252));
#27052=CARTESIAN_POINT('Ctrl Pts',(1.08745056285429,-1.,1.73662628326093));
#27053=CARTESIAN_POINT('Ctrl Pts',(1.08238162784749,-1.,1.73311705663407));
#27054=CARTESIAN_POINT('Ctrl Pts',(1.0773470373727,-1.,1.72957248977424));
#27055=CARTESIAN_POINT('Ctrl Pts',(1.07234866990252,-1.,1.72599406198489));
#27056=CARTESIAN_POINT('Ctrl Pts',(1.06738966975463,-1.,1.72238500928456));
#27057=CARTESIAN_POINT('Ctrl Pts',(1.06247324680649,-1.,1.71874858456908));
#27058=CARTESIAN_POINT('Ctrl Pts',(1.05760163192481,-1.,1.71508654427022));
#27059=CARTESIAN_POINT('Ctrl Pts',(1.05277517202853,-1.,1.71139783543986));
#27060=CARTESIAN_POINT('Ctrl Pts',(1.0479908540499,-1.,1.70767646263641));
#27061=CARTESIAN_POINT('Ctrl Pts',(1.04324363334546,-1.,1.70391338707969));
#27062=CARTESIAN_POINT('Ctrl Pts',(1.03852922490782,-1.,1.70010052930951));
#27063=CARTESIAN_POINT('Ctrl Pts',(1.03384646003587,-1.,1.69623414782769));
#27064=CARTESIAN_POINT('Ctrl Pts',(1.02919977579155,-1.,1.69231840863471));
#27065=CARTESIAN_POINT('Ctrl Pts',(1.02460180535272,-1.,1.68836910178475));
#27066=CARTESIAN_POINT('Ctrl Pts',(1.02006795074222,-1.,1.68440578021739));
#27067=CARTESIAN_POINT('Ctrl Pts',(1.01561026162786,-1.,1.6804428989482));
#27068=CARTESIAN_POINT('Ctrl Pts',(1.01123236493507,-1.,1.67648246776457));
#27069=CARTESIAN_POINT('Ctrl Pts',(1.00692206696387,-1.,1.67250335383248));
#27070=CARTESIAN_POINT('Ctrl Pts',(1.00265091003682,-1.,1.66846059277231));
#27071=CARTESIAN_POINT('Ctrl Pts',(0.998389654952317,-1.,1.66430758030304));
#27072=CARTESIAN_POINT('Ctrl Pts',(0.994121836661115,-1.,1.66001553809916));
#27073=CARTESIAN_POINT('Ctrl Pts',(0.98985562785445,-1.,1.65559044289746));
#27074=CARTESIAN_POINT('Ctrl Pts',(0.985642622921626,-1.,1.6511001661277));
#27075=CARTESIAN_POINT('Ctrl Pts',(0.981562530940574,-1.,1.64665139190834));
#27076=CARTESIAN_POINT('Ctrl Pts',(0.977689794120296,-1.,1.64233990826831));
#27077=CARTESIAN_POINT('Ctrl Pts',(0.974066058287501,-1.,1.63820952658157));
#27078=CARTESIAN_POINT('Ctrl Pts',(0.970669715996356,-1.,1.63420665729609));
#27079=CARTESIAN_POINT('Ctrl Pts',(0.967387853228041,-1.,1.63013849959083));
#27080=CARTESIAN_POINT('Ctrl Pts',(0.964046107037821,-1.,1.6257193066974));
#27081=CARTESIAN_POINT('Ctrl Pts',(0.960438326099958,-1.,1.62061638139929));
#27082=CARTESIAN_POINT('Ctrl Pts',(0.956354422921572,-1.,1.61449324337233));
#27083=CARTESIAN_POINT('Ctrl Pts',(0.951613284361247,-1.,1.60706069897794));
#27084=CARTESIAN_POINT('Ctrl Pts',(0.946078063325795,-1.,1.59810042045408));
#27085=CARTESIAN_POINT('Ctrl Pts',(0.939646377909319,-1.,1.58744937489796));
#27086=CARTESIAN_POINT('Ctrl Pts',(0.932246680128848,-1.,1.57499388385561));
#27087=CARTESIAN_POINT('Ctrl Pts',(0.923832188966322,-1.,1.56065988582509));
#27088=CARTESIAN_POINT('Ctrl Pts',(0.914375919046579,-1.,1.54440491152808));
#27089=CARTESIAN_POINT('Ctrl Pts',(0.905967409640498,-1.,1.52984849890434));
#27090=CARTESIAN_POINT('Ctrl Pts',(0.89918504749193,-1.,1.51805569591479));
#27091=CARTESIAN_POINT('Ctrl Pts',(0.894452006967538,-1.,1.50980486807181));
#27092=CARTESIAN_POINT('Ctrl Pts',(0.892032620296855,-1.,1.5055822144029));
#27093=CARTESIAN_POINT('',(0.693717979106305,-1.,1.60662857109684));
#27094=CARTESIAN_POINT('Origin',(0.,-1.,0.));
#27095=CARTESIAN_POINT('',(0.7455743247944,-1.,2.0698113262342));
#27096=CARTESIAN_POINT('Ctrl Pts',(0.693717979106305,-1.,1.60662857109684));
#27097=CARTESIAN_POINT('Ctrl Pts',(0.69571209787897,-1.,1.61106790957619));
#27098=CARTESIAN_POINT('Ctrl Pts',(0.699605146398836,-1.,1.61974673471117));
#27099=CARTESIAN_POINT('Ctrl Pts',(0.705159151977294,-1.,1.6321654166204));
#27100=CARTESIAN_POINT('Ctrl Pts',(0.711993139340447,-1.,1.64752408828442));
#27101=CARTESIAN_POINT('Ctrl Pts',(0.719585433787949,-1.,1.66472880551777));
#27102=CARTESIAN_POINT('Ctrl Pts',(0.726235967982445,-1.,1.67996158451922));
#27103=CARTESIAN_POINT('Ctrl Pts',(0.731963238685357,-1.,1.69326921972915));
#27104=CARTESIAN_POINT('Ctrl Pts',(0.736799665716932,-1.,1.70473309004249));
#27105=CARTESIAN_POINT('Ctrl Pts',(0.74079516202821,-1.,1.71447789751001));
#27106=CARTESIAN_POINT('Ctrl Pts',(0.744021445433093,-1.,1.72268229916769));
#27107=CARTESIAN_POINT('Ctrl Pts',(0.746574710097752,-1.,1.72958533647714));
#27108=CARTESIAN_POINT('Ctrl Pts',(0.74858246295687,-1.,1.7355035168033));
#27109=CARTESIAN_POINT('Ctrl Pts',(0.750193435981249,-1.,1.74080458267114));
#27110=CARTESIAN_POINT('Ctrl Pts',(0.751555614164482,-1.,1.74585086852502));
#27111=CARTESIAN_POINT('Ctrl Pts',(0.752797683531314,-1.,1.75095139468794));
#27112=CARTESIAN_POINT('Ctrl Pts',(0.754009254027828,-1.,1.75631083600019));
#27113=CARTESIAN_POINT('Ctrl Pts',(0.755220979974461,-1.,1.76197817240128));
#27114=CARTESIAN_POINT('Ctrl Pts',(0.75642189602781,-1.,1.76789396002998));
#27115=CARTESIAN_POINT('Ctrl Pts',(0.757578264077028,-1.,1.77394167108292));
#27116=CARTESIAN_POINT('Ctrl Pts',(0.758650626677518,-1.,1.77999411220945));
#27117=CARTESIAN_POINT('Ctrl Pts',(0.759614401110189,-1.,1.78596964884604));
#27118=CARTESIAN_POINT('Ctrl Pts',(0.760469555880749,-1.,1.7918581561088));
#27119=CARTESIAN_POINT('Ctrl Pts',(0.761229695230558,-1.,1.79768986997783));
#27120=CARTESIAN_POINT('Ctrl Pts',(0.761915336443547,-1.,1.80351583877342));
#27121=CARTESIAN_POINT('Ctrl Pts',(0.762546129463938,-1.,1.80938551463965));
#27122=CARTESIAN_POINT('Ctrl Pts',(0.763132003836634,-1.,1.8153211840553));
#27123=CARTESIAN_POINT('Ctrl Pts',(0.763673465462726,-1.,1.82131873145266));
#27124=CARTESIAN_POINT('Ctrl Pts',(0.764165902605995,-1.,1.82735991200065));
#27125=CARTESIAN_POINT('Ctrl Pts',(0.764602549687853,-1.,1.83342077227142));
#27126=CARTESIAN_POINT('Ctrl Pts',(0.764978057881737,-1.,1.83948181064835));
#27127=CARTESIAN_POINT('Ctrl Pts',(0.765291664862029,-1.,1.84553698875924));
#27128=CARTESIAN_POINT('Ctrl Pts',(0.765545710619062,-1.,1.85158945130063));
#27129=CARTESIAN_POINT('Ctrl Pts',(0.765744212909318,-1.,1.85764741390394));
#27130=CARTESIAN_POINT('Ctrl Pts',(0.765891519092547,-1.,1.86372027063312));
#27131=CARTESIAN_POINT('Ctrl Pts',(0.765990708546091,-1.,1.86981398314341));
#27132=CARTESIAN_POINT('Ctrl Pts',(0.766042837036744,-1.,1.87592888967883));
#27133=CARTESIAN_POINT('Ctrl Pts',(0.766047794851864,-1.,1.88206215302561));
#27134=CARTESIAN_POINT('Ctrl Pts',(0.766004837062091,-1.,1.88820926433409));
#27135=CARTESIAN_POINT('Ctrl Pts',(0.765913193856978,-1.,1.89436577771388));
#27136=CARTESIAN_POINT('Ctrl Pts',(0.765772772593386,-1.,1.90052930393596));
#27137=CARTESIAN_POINT('Ctrl Pts',(0.765584196937919,-1.,1.90669961402356));
#27138=CARTESIAN_POINT('Ctrl Pts',(0.765348465884722,-1.,1.91287765805169));
#27139=CARTESIAN_POINT('Ctrl Pts',(0.765066729667088,-1.,1.91906491634196));
#27140=CARTESIAN_POINT('Ctrl Pts',(0.764740025488211,-1.,1.92526263537048));
#27141=CARTESIAN_POINT('Ctrl Pts',(0.76436901067394,-1.,1.93147105496382));
#27142=CARTESIAN_POINT('Ctrl Pts',(0.763954049121458,-1.,1.93768964875886));
#27143=CARTESIAN_POINT('Ctrl Pts',(0.763495333538629,-1.,1.9439174661764));
#27144=CARTESIAN_POINT('Ctrl Pts',(0.762992990878769,-1.,1.95015342590024));
#27145=CARTESIAN_POINT('Ctrl Pts',(0.762447203806178,-1.,1.95639665309869));
#27146=CARTESIAN_POINT('Ctrl Pts',(0.761858300014423,-1.,1.96264672744186));
#27147=CARTESIAN_POINT('Ctrl Pts',(0.76122669048382,-1.,1.96890351582499));
#27148=CARTESIAN_POINT('Ctrl Pts',(0.760552825409757,-1.,1.97516705321494));
#27149=CARTESIAN_POINT('Ctrl Pts',(0.75983714745219,-1.,1.98143741418172));
#27150=CARTESIAN_POINT('Ctrl Pts',(0.759080037802488,-1.,1.98771456680874));
#27151=CARTESIAN_POINT('Ctrl Pts',(0.758281796766761,-1.,1.99399831098817));
#27152=CARTESIAN_POINT('Ctrl Pts',(0.757442676862724,-1.,2.00028834739178));
#27153=CARTESIAN_POINT('Ctrl Pts',(0.75656290464667,-1.,2.0065843158773));
#27154=CARTESIAN_POINT('Ctrl Pts',(0.755642704957865,-1.,2.01288584328084));
#27155=CARTESIAN_POINT('Ctrl Pts',(0.754682330722816,-1.,2.01919259405809));
#27156=CARTESIAN_POINT('Ctrl Pts',(0.753682061112768,-1.,2.02550428623313));
#27157=CARTESIAN_POINT('Ctrl Pts',(0.75264218048721,-1.,2.03182068456221));
#27158=CARTESIAN_POINT('Ctrl Pts',(0.751562963361115,-1.,2.03814160092099));
#27159=CARTESIAN_POINT('Ctrl Pts',(0.750444657875575,-1.,2.04446689147979));
#27160=CARTESIAN_POINT('Ctrl Pts',(0.749287468665046,-1.,2.05079645592154));
#27161=CARTESIAN_POINT('Ctrl Pts',(0.748091554183802,-1.,2.05713023031007));
#27162=CARTESIAN_POINT('Ctrl Pts',(0.747103932787919,-1.,2.06220058927826));
#27163=CARTESIAN_POINT('Ctrl Pts',(0.7463458715442,-1.,2.06600523016815));
#27164=CARTESIAN_POINT('Ctrl Pts',(0.745832791378367,-1.,2.06854248895728));
#27165=CARTESIAN_POINT('Ctrl Pts',(0.7455743247944,-1.,2.0698113262342));
#27166=CARTESIAN_POINT('',(0.61342227326009,-1.,2.11275013067528));
#27167=CARTESIAN_POINT('',(0.7455743247944,-1.,2.0698113262342));
#27168=CARTESIAN_POINT('',(0.383122945602004,-1.,1.7075470150345));
#27169=CARTESIAN_POINT('Ctrl Pts',(0.61342227326009,-1.,2.11275013067528));
#27170=CARTESIAN_POINT('Ctrl Pts',(0.6124673655618,-1.,2.11187554259986));
#27171=CARTESIAN_POINT('Ctrl Pts',(0.610560911689898,-1.,2.11012443807238));
#27172=CARTESIAN_POINT('Ctrl Pts',(0.607711315454876,-1.,2.1074919961518));
#27173=CARTESIAN_POINT('Ctrl Pts',(0.60393203073603,-1.,2.10397049886949));
#27174=CARTESIAN_POINT('Ctrl Pts',(0.599241616420533,-1.,2.0995493086477));
#27175=CARTESIAN_POINT('Ctrl Pts',(0.594585006052162,-1.,2.0951087622027));
#27176=CARTESIAN_POINT('Ctrl Pts',(0.589962365403406,-1.,2.09064881812129));
#27177=CARTESIAN_POINT('Ctrl Pts',(0.585373918991617,-1.,2.08616943727951));
#27178=CARTESIAN_POINT('Ctrl Pts',(0.580819952108063,-1.,2.08167059018418));
#27179=CARTESIAN_POINT('Ctrl Pts',(0.576300797416844,-1.,2.07715226767559));
#27180=CARTESIAN_POINT('Ctrl Pts',(0.571816823242602,-1.,2.07261449292824));
#27181=CARTESIAN_POINT('Ctrl Pts',(0.567368421181087,-1.,2.06805732997334));
#27182=CARTESIAN_POINT('Ctrl Pts',(0.562955993082261,-1.,2.06348090160589));
#27183=CARTESIAN_POINT('Ctrl Pts',(0.558579940185151,-1.,2.05888537756462));
#27184=CARTESIAN_POINT('Ctrl Pts',(0.554240657463906,-1.,2.05427091604413));
#27185=CARTESIAN_POINT('Ctrl Pts',(0.549938525150295,-1.,2.04963761077958));
#27186=CARTESIAN_POINT('Ctrl Pts',(0.54567390381743,-1.,2.04498544714588));
#27187=CARTESIAN_POINT('Ctrl Pts',(0.541447120615659,-1.,2.04031422690527));
#27188=CARTESIAN_POINT('Ctrl Pts',(0.537258489833262,-1.,2.03562362954037));
#27189=CARTESIAN_POINT('Ctrl Pts',(0.533108355132976,-1.,2.03091336214426));
#27190=CARTESIAN_POINT('Ctrl Pts',(0.528997127241914,-1.,2.0261832908329));
#27191=CARTESIAN_POINT('Ctrl Pts',(0.524925318333476,-1.,2.02143356304698));
#27192=CARTESIAN_POINT('Ctrl Pts',(0.52089359039937,-1.,2.01666477917286));
#27193=CARTESIAN_POINT('Ctrl Pts',(0.516902681728687,-1.,2.01187773939242));
#27194=CARTESIAN_POINT('Ctrl Pts',(0.512953306961792,-1.,2.00707309946949));
#27195=CARTESIAN_POINT('Ctrl Pts',(0.509046069886157,-1.,2.00225107134734));
#27196=CARTESIAN_POINT('Ctrl Pts',(0.505181361323026,-1.,1.99741107463572));
#27197=CARTESIAN_POINT('Ctrl Pts',(0.501359287727146,-1.,1.99255149126155));
#27198=CARTESIAN_POINT('Ctrl Pts',(0.497579909545574,-1.,1.98767044752932));
#27199=CARTESIAN_POINT('Ctrl Pts',(0.493843476541494,-1.,1.98276658761821));
#27200=CARTESIAN_POINT('Ctrl Pts',(0.490150627860952,-1.,1.97783973019229));
#27201=CARTESIAN_POINT('Ctrl Pts',(0.486502692907658,-1.,1.97289186263272));
#27202=CARTESIAN_POINT('Ctrl Pts',(0.48290166212069,-1.,1.96792703422362));
#27203=CARTESIAN_POINT('Ctrl Pts',(0.479349583074855,-1.,1.96294933055943));
#27204=CARTESIAN_POINT('Ctrl Pts',(0.475848034683176,-1.,1.95796111148177));
#27205=CARTESIAN_POINT('Ctrl Pts',(0.472397672264072,-1.,1.95296148278133));
#27206=CARTESIAN_POINT('Ctrl Pts',(0.468997482913135,-1.,1.94794381136514));
#27207=CARTESIAN_POINT('Ctrl Pts',(0.46564546202603,-1.,1.9428979419619));
#27208=CARTESIAN_POINT('Ctrl Pts',(0.462340031009056,-1.,1.93781486640821));
#27209=CARTESIAN_POINT('Ctrl Pts',(0.459081234547926,-1.,1.93269066517934));
#27210=CARTESIAN_POINT('Ctrl Pts',(0.45587200517437,-1.,1.92753067150476));
#27211=CARTESIAN_POINT('Ctrl Pts',(0.452719478359432,-1.,1.92235380648502));
#27212=CARTESIAN_POINT('Ctrl Pts',(0.449632260106662,-1.,1.91718342555755));
#27213=CARTESIAN_POINT('Ctrl Pts',(0.446617343485711,-1.,1.9120369998112));
#27214=CARTESIAN_POINT('Ctrl Pts',(0.44367755684915,-1.,1.90691756144898));
#27215=CARTESIAN_POINT('Ctrl Pts',(0.440807833704038,-1.,1.90180124389086));
#27216=CARTESIAN_POINT('Ctrl Pts',(0.437995003948244,-1.,1.89663648956466));
#27217=CARTESIAN_POINT('Ctrl Pts',(0.435225660963383,-1.,1.89136993975504));
#27218=CARTESIAN_POINT('Ctrl Pts',(0.432493038548748,-1.,1.88596913666793));
#27219=CARTESIAN_POINT('Ctrl Pts',(0.429803062482344,-1.,1.88044229001832));
#27220=CARTESIAN_POINT('Ctrl Pts',(0.427183828519102,-1.,1.87486989291484));
#27221=CARTESIAN_POINT('Ctrl Pts',(0.424678177291358,-1.,1.86937803944323));
#27222=CARTESIAN_POINT('Ctrl Pts',(0.422327307418275,-1.,1.86408083334028));
#27223=CARTESIAN_POINT('Ctrl Pts',(0.420157287975619,-1.,1.85903281096686));
#27224=CARTESIAN_POINT('Ctrl Pts',(0.418164129143534,-1.,1.85417632856234));
#27225=CARTESIAN_POINT('Ctrl Pts',(0.416300022038864,-1.,1.84929312929882));
#27226=CARTESIAN_POINT('Ctrl Pts',(0.41448743825434,-1.,1.8440575707371));
#27227=CARTESIAN_POINT('Ctrl Pts',(0.412633125322161,-1.,1.83808953475839));
#27228=CARTESIAN_POINT('Ctrl Pts',(0.410641256301674,-1.,1.83100408895216));
#27229=CARTESIAN_POINT('Ctrl Pts',(0.408428948108533,-1.,1.8224702267854));
#27230=CARTESIAN_POINT('Ctrl Pts',(0.405933518411838,-1.,1.81223801813988));
#27231=CARTESIAN_POINT('Ctrl Pts',(0.403107976170441,-1.,1.80012077176221));
#27232=CARTESIAN_POINT('Ctrl Pts',(0.39991940378308,-1.,1.78598826347533));
#27233=CARTESIAN_POINT('Ctrl Pts',(0.39634619612042,-1.,1.7697556004756));
#27234=CARTESIAN_POINT('Ctrl Pts',(0.392375812294307,-1.,1.75137405313962));
#27235=CARTESIAN_POINT('Ctrl Pts',(0.388877023509191,-1.,1.7349317097561));
#27236=CARTESIAN_POINT('Ctrl Pts',(0.38607079032701,-1.,1.72162022246158));
#27237=CARTESIAN_POINT('Ctrl Pts',(0.384119047315541,-1.,1.71231062891958));
#27238=CARTESIAN_POINT('Ctrl Pts',(0.383122945602004,-1.,1.7075470150345));
#27239=CARTESIAN_POINT('',(0.163289472382896,-1.,1.74236521665491));
#27240=CARTESIAN_POINT('Origin',(0.,-1.,0.));
#27241=CARTESIAN_POINT('',(0.0694764450219578,-1.,2.19890268624765));
#27242=CARTESIAN_POINT('Ctrl Pts',(0.163289472382896,-1.,1.74236521665491));
#27243=CARTESIAN_POINT('Ctrl Pts',(0.163814161002002,-1.,1.7472034950333));
#27244=CARTESIAN_POINT('Ctrl Pts',(0.164834765707158,-1.,1.75666056638427));
#27245=CARTESIAN_POINT('Ctrl Pts',(0.1662793551464,-1.,1.77018771684844));
#27246=CARTESIAN_POINT('Ctrl Pts',(0.168032772805197,-1.,1.7869064998507));
#27247=CARTESIAN_POINT('Ctrl Pts',(0.169936923904608,-1.,1.80561530629706));
#27248=CARTESIAN_POINT('Ctrl Pts',(0.171554770204119,-1.,1.82215766811545));
#27249=CARTESIAN_POINT('Ctrl Pts',(0.1728894428919,-1.,1.83658380527692));
#27250=CARTESIAN_POINT('Ctrl Pts',(0.173946627587731,-1.,1.8489811319852));
#27251=CARTESIAN_POINT('Ctrl Pts',(0.17473525927603,-1.,1.85948367088837));
#27252=CARTESIAN_POINT('Ctrl Pts',(0.175268337590757,-1.,1.86828349694799));
#27253=CARTESIAN_POINT('Ctrl Pts',(0.175563480746485,-1.,1.87563767773588));
#27254=CARTESIAN_POINT('Ctrl Pts',(0.175644148889698,-1.,1.88188663145367));
#27255=CARTESIAN_POINT('Ctrl Pts',(0.175538155840648,-1.,1.88742606273259));
#27256=CARTESIAN_POINT('Ctrl Pts',(0.175274276190844,-1.,1.892646301985));
#27257=CARTESIAN_POINT('Ctrl Pts',(0.174879405091263,-1.,1.89788101117132));
#27258=CARTESIAN_POINT('Ctrl Pts',(0.174375518661085,-1.,1.90335253862834));
#27259=CARTESIAN_POINT('Ctrl Pts',(0.173776635257816,-1.,1.90911693975267));
#27260=CARTESIAN_POINT('Ctrl Pts',(0.173090695383496,-1.,1.91511429159527));
#27261=CARTESIAN_POINT('Ctrl Pts',(0.172321621259513,-1.,1.9212233439798));
#27262=CARTESIAN_POINT('Ctrl Pts',(0.171471191532988,-1.,1.92731093582036));
#27263=CARTESIAN_POINT('Ctrl Pts',(0.170541253116201,-1.,1.93329183155539));
#27264=CARTESIAN_POINT('Ctrl Pts',(0.16953490481749,-1.,1.93915639211581));
#27265=CARTESIAN_POINT('Ctrl Pts',(0.168455741607556,-1.,1.94493757756931));
#27266=CARTESIAN_POINT('Ctrl Pts',(0.167307501784475,-1.,1.95069027794294));
#27267=CARTESIAN_POINT('Ctrl Pts',(0.166093592002812,-1.,1.9564675971873));
#27268=CARTESIAN_POINT('Ctrl Pts',(0.164816568920269,-1.,1.96229379940136));
#27269=CARTESIAN_POINT('Ctrl Pts',(0.163478185457734,-1.,1.96816512677967));
#27270=CARTESIAN_POINT('Ctrl Pts',(0.162079693556288,-1.,1.97406280235188));
#27271=CARTESIAN_POINT('Ctrl Pts',(0.160622060784611,-1.,1.97996195437559));
#27272=CARTESIAN_POINT('Ctrl Pts',(0.159106226437299,-1.,1.98584238283292));
#27273=CARTESIAN_POINT('Ctrl Pts',(0.157533331459227,-1.,1.99169810931908));
#27274=CARTESIAN_POINT('Ctrl Pts',(0.155904629548783,-1.,1.99753284771497));
#27275=CARTESIAN_POINT('Ctrl Pts',(0.154221403049722,-1.,2.00335565310543));
#27276=CARTESIAN_POINT('Ctrl Pts',(0.152484883621449,-1.,2.00917680318424));
#27277=CARTESIAN_POINT('Ctrl Pts',(0.150696157673078,-1.,2.01500291940238));
#27278=CARTESIAN_POINT('Ctrl Pts',(0.148856124775337,-1.,2.02083464969894));
#27279=CARTESIAN_POINT('Ctrl Pts',(0.146965557332583,-1.,2.02666926182017));
#27280=CARTESIAN_POINT('Ctrl Pts',(0.145025140186057,-1.,2.03250223739942));
#27281=CARTESIAN_POINT('Ctrl Pts',(0.143035515058208,-1.,2.03832911025912));
#27282=CARTESIAN_POINT('Ctrl Pts',(0.140997332152546,-1.,2.04414757947916));
#27283=CARTESIAN_POINT('Ctrl Pts',(0.138911255368966,-1.,2.04995762001328));
#27284=CARTESIAN_POINT('Ctrl Pts',(0.136777941218043,-1.,2.05576044414264));
#27285=CARTESIAN_POINT('Ctrl Pts',(0.134598026192106,-1.,2.06155781517842));
#27286=CARTESIAN_POINT('Ctrl Pts',(0.13237211154771,-1.,2.06735123910326));
#27287=CARTESIAN_POINT('Ctrl Pts',(0.130100748328403,-1.,2.07314114713063));
#27288=CARTESIAN_POINT('Ctrl Pts',(0.12778444527612,-1.,2.07892715110987));
#27289=CARTESIAN_POINT('Ctrl Pts',(0.125423679412061,-1.,2.08470840653643));
#27290=CARTESIAN_POINT('Ctrl Pts',(0.123018905621083,-1.,2.09048392424825));
#27291=CARTESIAN_POINT('Ctrl Pts',(0.120570567965122,-1.,2.0962529286773));
#27292=CARTESIAN_POINT('Ctrl Pts',(0.118079107988355,-1.,2.102015121329));
#27293=CARTESIAN_POINT('Ctrl Pts',(0.115544957687926,-1.,2.10777050261309));
#27294=CARTESIAN_POINT('Ctrl Pts',(0.112968534419737,-1.,2.11351924490306));
#27295=CARTESIAN_POINT('Ctrl Pts',(0.110350236135025,-1.,2.11926155590865));
#27296=CARTESIAN_POINT('Ctrl Pts',(0.10769043523109,-1.,2.12499752307));
#27297=CARTESIAN_POINT('Ctrl Pts',(0.104989479152739,-1.,2.13072704887293));
#27298=CARTESIAN_POINT('Ctrl Pts',(0.1022477005561,-1.,2.13644992667165));
#27299=CARTESIAN_POINT('Ctrl Pts',(0.0994654261990913,-1.,2.14216588396025));
#27300=CARTESIAN_POINT('Ctrl Pts',(0.0966429852305456,-1.,2.14787463531795));
#27301=CARTESIAN_POINT('Ctrl Pts',(0.0937807218867641,-1.,2.1535759397817));
#27302=CARTESIAN_POINT('Ctrl Pts',(0.0908789888107263,-1.,2.15926961544516));
#27303=CARTESIAN_POINT('Ctrl Pts',(0.087938129138692,-1.,2.16495552645014));
#27304=CARTESIAN_POINT('Ctrl Pts',(0.084958462083537,-1.,2.17063357870952));
#27305=CARTESIAN_POINT('Ctrl Pts',(0.0819402680872763,-1.,2.176303712113));
#27306=CARTESIAN_POINT('Ctrl Pts',(0.078883772768524,-1.,2.18196589448887));
#27307=CARTESIAN_POINT('Ctrl Pts',(0.0757891465836145,-1.,2.1876201139953));
#27308=CARTESIAN_POINT('Ctrl Pts',(0.0732830357306722,-1.,2.19213712013662));
#27309=CARTESIAN_POINT('Ctrl Pts',(0.0713863779526151,-1.,2.19552129484002));
#27310=CARTESIAN_POINT('Ctrl Pts',(0.0701143536325487,-1.,2.19777582085423));
#27311=CARTESIAN_POINT('Ctrl Pts',(0.0694764450219578,-1.,2.19890268624765));
#27312=CARTESIAN_POINT('',(-0.0694764450219586,-1.,2.19890268624765));
#27313=CARTESIAN_POINT('',(0.0694764450219578,-1.,2.19890268624765));
#27314=CARTESIAN_POINT('',(-0.163289472382896,-1.,1.74236521665491));
#27315=CARTESIAN_POINT('Ctrl Pts',(-0.0694764450219586,-1.,2.19890268624765));
#27316=CARTESIAN_POINT('Ctrl Pts',(-0.0701143536324929,-1.,2.19777582085261));
#27317=CARTESIAN_POINT('Ctrl Pts',(-0.071386377952463,-1.,2.19552129483562));
#27318=CARTESIAN_POINT('Ctrl Pts',(-0.0732830357304279,-1.,2.19213712012956));
#27319=CARTESIAN_POINT('Ctrl Pts',(-0.0757891465833414,-1.,2.1876201139874));
#27320=CARTESIAN_POINT('Ctrl Pts',(-0.078883772768323,-1.,2.18196589448304));
#27321=CARTESIAN_POINT('Ctrl Pts',(-0.0819402680871942,-1.,2.1763037121106));
#27322=CARTESIAN_POINT('Ctrl Pts',(-0.0849584620835646,-1.,2.17063357871031));
#27323=CARTESIAN_POINT('Ctrl Pts',(-0.0879381291387825,-1.,2.16495552645275));
#27324=CARTESIAN_POINT('Ctrl Pts',(-0.0908789888108269,-1.,2.15926961544808));
#27325=CARTESIAN_POINT('Ctrl Pts',(-0.0937807218868348,-1.,2.15357593978377));
#27326=CARTESIAN_POINT('Ctrl Pts',(-0.0966429852305691,-1.,2.14787463531864));
#27327=CARTESIAN_POINT('Ctrl Pts',(-0.0994654261990745,-1.,2.14216588395974));
#27328=CARTESIAN_POINT('Ctrl Pts',(-0.102247700556064,-1.,2.13644992667052));
#27329=CARTESIAN_POINT('Ctrl Pts',(-0.104989479152703,-1.,2.1307270488718));
#27330=CARTESIAN_POINT('Ctrl Pts',(-0.107690435231068,-1.,2.12499752306927));
#27331=CARTESIAN_POINT('Ctrl Pts',(-0.11035023613502,-1.,2.11926155590849));
#27332=CARTESIAN_POINT('Ctrl Pts',(-0.112968534419746,-1.,2.11351924490335));
#27333=CARTESIAN_POINT('Ctrl Pts',(-0.115544957687941,-1.,2.10777050261359));
#27334=CARTESIAN_POINT('Ctrl Pts',(-0.118079107988368,-1.,2.10201512132945));
#27335=CARTESIAN_POINT('Ctrl Pts',(-0.120570567965129,-1.,2.09625292867756));
#27336=CARTESIAN_POINT('Ctrl Pts',(-0.123018905621083,-1.,2.09048392424826));
#27337=CARTESIAN_POINT('Ctrl Pts',(-0.125423679412058,-1.,2.08470840653628));
#27338=CARTESIAN_POINT('Ctrl Pts',(-0.127784445276116,-1.,2.07892715110967));
#27339=CARTESIAN_POINT('Ctrl Pts',(-0.130100748328401,-1.,2.07314114713047));
#27340=CARTESIAN_POINT('Ctrl Pts',(-0.13237211154771,-1.,2.06735123910319));
#27341=CARTESIAN_POINT('Ctrl Pts',(-0.134598026192107,-1.,2.06155781517844));
#27342=CARTESIAN_POINT('Ctrl Pts',(-0.136777941218044,-1.,2.0557604441427));
#27343=CARTESIAN_POINT('Ctrl Pts',(-0.138911255368966,-1.,2.04995762001333));
#27344=CARTESIAN_POINT('Ctrl Pts',(-0.140997332152546,-1.,2.04414757947919));
#27345=CARTESIAN_POINT('Ctrl Pts',(-0.143035515058208,-1.,2.03832911025913));
#27346=CARTESIAN_POINT('Ctrl Pts',(-0.145025140186058,-1.,2.03250223739941));
#27347=CARTESIAN_POINT('Ctrl Pts',(-0.146965557332586,-1.,2.02666926182017));
#27348=CARTESIAN_POINT('Ctrl Pts',(-0.148856124775343,-1.,2.02083464969897));
#27349=CARTESIAN_POINT('Ctrl Pts',(-0.150696157673084,-1.,2.01500291940243));
#27350=CARTESIAN_POINT('Ctrl Pts',(-0.152484883621452,-1.,2.00917680318426));
#27351=CARTESIAN_POINT('Ctrl Pts',(-0.154221403049719,-1.,2.00335565310539));
#27352=CARTESIAN_POINT('Ctrl Pts',(-0.155904629548775,-1.,1.99753284771487));
#27353=CARTESIAN_POINT('Ctrl Pts',(-0.157533331459215,-1.,1.99169810931893));
#27354=CARTESIAN_POINT('Ctrl Pts',(-0.159106226437289,-1.,1.98584238283279));
#27355=CARTESIAN_POINT('Ctrl Pts',(-0.16062206078461,-1.,1.97996195437557));
#27356=CARTESIAN_POINT('Ctrl Pts',(-0.162079693556302,-1.,1.97406280235204));
#27357=CARTESIAN_POINT('Ctrl Pts',(-0.16347818545776,-1.,1.96816512678));
#27358=CARTESIAN_POINT('Ctrl Pts',(-0.1648165689203,-1.,1.96229379940174));
#27359=CARTESIAN_POINT('Ctrl Pts',(-0.166093592002833,-1.,1.95646759718755));
#27360=CARTESIAN_POINT('Ctrl Pts',(-0.167307501784469,-1.,1.95069027794286));
#27361=CARTESIAN_POINT('Ctrl Pts',(-0.168455741607516,-1.,1.94493757756879));
#27362=CARTESIAN_POINT('Ctrl Pts',(-0.169534904817425,-1.,1.93915639211497));
#27363=CARTESIAN_POINT('Ctrl Pts',(-0.170541253116136,-1.,1.93329183155455));
#27364=CARTESIAN_POINT('Ctrl Pts',(-0.17147119153296,-1.,1.92731093582));
#27365=CARTESIAN_POINT('Ctrl Pts',(-0.172321621259557,-1.,1.92122334398034));
#27366=CARTESIAN_POINT('Ctrl Pts',(-0.173090695383619,-1.,1.91511429159681));
#27367=CARTESIAN_POINT('Ctrl Pts',(-0.173776635257984,-1.,1.90911693975475));
#27368=CARTESIAN_POINT('Ctrl Pts',(-0.174375518661222,-1.,1.90335253863003));
#27369=CARTESIAN_POINT('Ctrl Pts',(-0.174879405091277,-1.,1.89788101117148));
#27370=CARTESIAN_POINT('Ctrl Pts',(-0.175274276190664,-1.,1.89264630198279));
#27371=CARTESIAN_POINT('Ctrl Pts',(-0.175538155840286,-1.,1.88742606272818));
#27372=CARTESIAN_POINT('Ctrl Pts',(-0.175644148889271,-1.,1.88188663144846));
#27373=CARTESIAN_POINT('Ctrl Pts',(-0.175563480746206,-1.,1.87563767773249));
#27374=CARTESIAN_POINT('Ctrl Pts',(-0.175268337590901,-1.,1.86828349694972));
#27375=CARTESIAN_POINT('Ctrl Pts',(-0.174735259276856,-1.,1.85948367089838));
#27376=CARTESIAN_POINT('Ctrl Pts',(-0.173946627589401,-1.,1.84898113200543));
#27377=CARTESIAN_POINT('Ctrl Pts',(-0.17288944289442,-1.,1.83658380530747));
#27378=CARTESIAN_POINT('Ctrl Pts',(-0.171554770207306,-1.,1.82215766815414));
#27379=CARTESIAN_POINT('Ctrl Pts',(-0.169936923908078,-1.,1.80561530633924));
#27380=CARTESIAN_POINT('Ctrl Pts',(-0.16803277280837,-1.,1.78690649988931));
#27381=CARTESIAN_POINT('Ctrl Pts',(-0.166279355148738,-1.,1.77018771687692));
#27382=CARTESIAN_POINT('Ctrl Pts',(-0.164834765708484,-1.,1.75666056640041));
#27383=CARTESIAN_POINT('Ctrl Pts',(-0.163814161002474,-1.,1.74720349503904));
#27384=CARTESIAN_POINT('Ctrl Pts',(-0.163289472382896,-1.,1.74236521665491));
#27385=CARTESIAN_POINT('',(-0.383122945602004,-1.,1.7075470150345));
#27386=CARTESIAN_POINT('Origin',(0.,-1.,0.));
#27387=CARTESIAN_POINT('',(-0.61342227326009,-1.,2.11275013067528));
#27388=CARTESIAN_POINT('Ctrl Pts',(-0.383122945602004,-1.,1.7075470150345));
#27389=CARTESIAN_POINT('Ctrl Pts',(-0.384119047314215,-1.,1.71231062891398));
#27390=CARTESIAN_POINT('Ctrl Pts',(-0.386070790323281,-1.,1.72162022244582));
#27391=CARTESIAN_POINT('Ctrl Pts',(-0.388877023502615,-1.,1.73493170972829));
#27392=CARTESIAN_POINT('Ctrl Pts',(-0.392375812285395,-1.,1.75137405310193));
#27393=CARTESIAN_POINT('Ctrl Pts',(-0.396346196110688,-1.,1.76975560043442));
#27394=CARTESIAN_POINT('Ctrl Pts',(-0.399919403774155,-1.,1.78598826343754));
#27395=CARTESIAN_POINT('Ctrl Pts',(-0.403107976163396,-1.,1.80012077173238));
#27396=CARTESIAN_POINT('Ctrl Pts',(-0.405933518407175,-1.,1.81223801812013));
#27397=CARTESIAN_POINT('Ctrl Pts',(-0.408428948106227,-1.,1.82247022677562));
#27398=CARTESIAN_POINT('Ctrl Pts',(-0.410641256301276,-1.,1.83100408895047));
#27399=CARTESIAN_POINT('Ctrl Pts',(-0.412633125322945,-1.,1.8380895347617));
#27400=CARTESIAN_POINT('Ctrl Pts',(-0.414487438255542,-1.,1.84405757074218));
#27401=CARTESIAN_POINT('Ctrl Pts',(-0.416300022039885,-1.,1.84929312930314));
#27402=CARTESIAN_POINT('Ctrl Pts',(-0.418164129144045,-1.,1.8541763285645));
#27403=CARTESIAN_POINT('Ctrl Pts',(-0.420157287975583,-1.,1.8590328109667));
#27404=CARTESIAN_POINT('Ctrl Pts',(-0.422327307417885,-1.,1.86408083333863));
#27405=CARTESIAN_POINT('Ctrl Pts',(-0.424678177290876,-1.,1.8693780394412));
#27406=CARTESIAN_POINT('Ctrl Pts',(-0.427183828518743,-1.,1.87486989291333));
#27407=CARTESIAN_POINT('Ctrl Pts',(-0.429803062482217,-1.,1.88044229001778));
#27408=CARTESIAN_POINT('Ctrl Pts',(-0.432493038548833,-1.,1.88596913666828));
#27409=CARTESIAN_POINT('Ctrl Pts',(-0.43522566096358,-1.,1.89136993975585));
#27410=CARTESIAN_POINT('Ctrl Pts',(-0.437995003948443,-1.,1.89663648956549));
#27411=CARTESIAN_POINT('Ctrl Pts',(-0.440807833704161,-1.,1.90180124389137));
#27412=CARTESIAN_POINT('Ctrl Pts',(-0.44367755684917,-1.,1.90691756144906));
#27413=CARTESIAN_POINT('Ctrl Pts',(-0.446617343485651,-1.,1.91203699981095));
#27414=CARTESIAN_POINT('Ctrl Pts',(-0.449632260106572,-1.,1.91718342555717));
#27415=CARTESIAN_POINT('Ctrl Pts',(-0.452719478359356,-1.,1.9223538064847));
#27416=CARTESIAN_POINT('Ctrl Pts',(-0.455872005174335,-1.,1.92753067150461));
#27417=CARTESIAN_POINT('Ctrl Pts',(-0.459081234547931,-1.,1.93269066517936));
#27418=CARTESIAN_POINT('Ctrl Pts',(-0.462340031009087,-1.,1.93781486640834));
#27419=CARTESIAN_POINT('Ctrl Pts',(-0.465645462026065,-1.,1.94289794196205));
#27420=CARTESIAN_POINT('Ctrl Pts',(-0.468997482913158,-1.,1.94794381136524));
#27421=CARTESIAN_POINT('Ctrl Pts',(-0.47239767226408,-1.,1.95296148278136));
#27422=CARTESIAN_POINT('Ctrl Pts',(-0.475848034683172,-1.,1.95796111148175));
#27423=CARTESIAN_POINT('Ctrl Pts',(-0.479349583074846,-1.,1.96294933055938));
#27424=CARTESIAN_POINT('Ctrl Pts',(-0.482901662120687,-1.,1.96792703422358));
#27425=CARTESIAN_POINT('Ctrl Pts',(-0.486502692907661,-1.,1.97289186263272));
#27426=CARTESIAN_POINT('Ctrl Pts',(-0.490150627860955,-1.,1.97783973019229));
#27427=CARTESIAN_POINT('Ctrl Pts',(-0.493843476541492,-1.,1.9827665876182));
#27428=CARTESIAN_POINT('Ctrl Pts',(-0.497579909545564,-1.,1.98767044752929));
#27429=CARTESIAN_POINT('Ctrl Pts',(-0.501359287727129,-1.,1.9925514912615));
#27430=CARTESIAN_POINT('Ctrl Pts',(-0.505181361323011,-1.,1.99741107463567));
#27431=CARTESIAN_POINT('Ctrl Pts',(-0.509046069886152,-1.,2.00225107134733));
#27432=CARTESIAN_POINT('Ctrl Pts',(-0.512953306961814,-1.,2.00707309946955));
#27433=CARTESIAN_POINT('Ctrl Pts',(-0.516902681728733,-1.,2.01187773939257));
#27434=CARTESIAN_POINT('Ctrl Pts',(-0.520893590399428,-1.,2.01666477917305));
#27435=CARTESIAN_POINT('Ctrl Pts',(-0.524925318333518,-1.,2.02143356304712));
#27436=CARTESIAN_POINT('Ctrl Pts',(-0.528997127241911,-1.,2.02618329083289));
#27437=CARTESIAN_POINT('Ctrl Pts',(-0.533108355132905,-1.,2.03091336214401));
#27438=CARTESIAN_POINT('Ctrl Pts',(-0.537258489833134,-1.,2.03562362953993));
#27439=CARTESIAN_POINT('Ctrl Pts',(-0.54144712061552,-1.,2.0403142269048));
#27440=CARTESIAN_POINT('Ctrl Pts',(-0.545673903817348,-1.,2.0449854471456));
#27441=CARTESIAN_POINT('Ctrl Pts',(-0.549938525150342,-1.,2.04963761077974));
#27442=CARTESIAN_POINT('Ctrl Pts',(-0.55424065746411,-1.,2.05427091604482));
#27443=CARTESIAN_POINT('Ctrl Pts',(-0.558579940185467,-1.,2.05888537756571));
#27444=CARTESIAN_POINT('Ctrl Pts',(-0.562955993082574,-1.,2.06348090160697));
#27445=CARTESIAN_POINT('Ctrl Pts',(-0.567368421181229,-1.,2.06805732997383));
#27446=CARTESIAN_POINT('Ctrl Pts',(-0.571816823242411,-1.,2.07261449292757));
#27447=CARTESIAN_POINT('Ctrl Pts',(-0.576300797416275,-1.,2.07715226767361));
#27448=CARTESIAN_POINT('Ctrl Pts',(-0.580819952107257,-1.,2.08167059018138));
#27449=CARTESIAN_POINT('Ctrl Pts',(-0.585373918990895,-1.,2.086169437277));
#27450=CARTESIAN_POINT('Ctrl Pts',(-0.589962365403189,-1.,2.09064881812053));
#27451=CARTESIAN_POINT('Ctrl Pts',(-0.594585006052824,-1.,2.09510876220501));
#27452=CARTESIAN_POINT('Ctrl Pts',(-0.599241616422144,-1.,2.09954930865331));
#27453=CARTESIAN_POINT('Ctrl Pts',(-0.603932030738212,-1.,2.10397049887709));
#27454=CARTESIAN_POINT('Ctrl Pts',(-0.607711315456826,-1.,2.10749199615859));
#27455=CARTESIAN_POINT('Ctrl Pts',(-0.610560911691113,-1.,2.11012443807661));
#27456=CARTESIAN_POINT('Ctrl Pts',(-0.61246736556225,-1.,2.11187554260142));
#27457=CARTESIAN_POINT('Ctrl Pts',(-0.61342227326009,-1.,2.11275013067528));
#27458=CARTESIAN_POINT('',(-0.745574324794401,-1.,2.0698113262342));
#27459=CARTESIAN_POINT('',(-0.61342227326009,-1.,2.11275013067528));
#27460=CARTESIAN_POINT('',(-0.693717979106306,-1.,1.60662857109684));
#27461=CARTESIAN_POINT('Ctrl Pts',(-0.745574324794401,-1.,2.0698113262342));
#27462=CARTESIAN_POINT('Ctrl Pts',(-0.74583279137781,-1.,2.06854248895575));
#27463=CARTESIAN_POINT('Ctrl Pts',(-0.746345871542696,-1.,2.06600523016401));
#27464=CARTESIAN_POINT('Ctrl Pts',(-0.747103932785504,-1.,2.06220058927162));
#27465=CARTESIAN_POINT('Ctrl Pts',(-0.748091554181101,-1.,2.05713023030263));
#27466=CARTESIAN_POINT('Ctrl Pts',(-0.749287468663053,-1.,2.05079645591606));
#27467=CARTESIAN_POINT('Ctrl Pts',(-0.750444657874758,-1.,2.04446689147754));
#27468=CARTESIAN_POINT('Ctrl Pts',(-0.751562963361384,-1.,2.03814160092173));
#27469=CARTESIAN_POINT('Ctrl Pts',(-0.752642180488104,-1.,2.03182068456467));
#27470=CARTESIAN_POINT('Ctrl Pts',(-0.753682061113766,-1.,2.02550428623587));
#27471=CARTESIAN_POINT('Ctrl Pts',(-0.75468233072352,-1.,2.01919259406003));
#27472=CARTESIAN_POINT('Ctrl Pts',(-0.7556427049581,-1.,2.01288584328149));
#27473=CARTESIAN_POINT('Ctrl Pts',(-0.756562904646496,-1.,2.00658431587682));
#27474=CARTESIAN_POINT('Ctrl Pts',(-0.757442676862341,-1.,2.00028834739072));
#27475=CARTESIAN_POINT('Ctrl Pts',(-0.758281796766377,-1.,1.9939983109871));
#27476=CARTESIAN_POINT('Ctrl Pts',(-0.759080037802243,-1.,1.98771456680806));
#27477=CARTESIAN_POINT('Ctrl Pts',(-0.759837147452135,-1.,1.98143741418156));
#27478=CARTESIAN_POINT('Ctrl Pts',(-0.760552825409855,-1.,1.97516705321521));
#27479=CARTESIAN_POINT('Ctrl Pts',(-0.761226690483986,-1.,1.96890351582545));
#27480=CARTESIAN_POINT('Ctrl Pts',(-0.761858300014575,-1.,1.96264672744229));
#27481=CARTESIAN_POINT('Ctrl Pts',(-0.762447203806263,-1.,1.95639665309893));
#27482=CARTESIAN_POINT('Ctrl Pts',(-0.762992990878774,-1.,1.95015342590025));
#27483=CARTESIAN_POINT('Ctrl Pts',(-0.76349533353858,-1.,1.94391746617626));
#27484=CARTESIAN_POINT('Ctrl Pts',(-0.763954049121393,-1.,1.93768964875867));
#27485=CARTESIAN_POINT('Ctrl Pts',(-0.764369010673889,-1.,1.93147105496367));
#27486=CARTESIAN_POINT('Ctrl Pts',(-0.764740025488189,-1.,1.92526263537041));
#27487=CARTESIAN_POINT('Ctrl Pts',(-0.765066729667095,-1.,1.91906491634197));
#27488=CARTESIAN_POINT('Ctrl Pts',(-0.765348465884739,-1.,1.91287765805174));
#27489=CARTESIAN_POINT('Ctrl Pts',(-0.765584196937936,-1.,1.90669961402362));
#27490=CARTESIAN_POINT('Ctrl Pts',(-0.765772772593395,-1.,1.90052930393599));
#27491=CARTESIAN_POINT('Ctrl Pts',(-0.765913193856979,-1.,1.89436577771389));
#27492=CARTESIAN_POINT('Ctrl Pts',(-0.76600483706209,-1.,1.88820926433409));
#27493=CARTESIAN_POINT('Ctrl Pts',(-0.766047794851869,-1.,1.88206215302561));
#27494=CARTESIAN_POINT('Ctrl Pts',(-0.766042837036759,-1.,1.87592888967886));
#27495=CARTESIAN_POINT('Ctrl Pts',(-0.765990708546111,-1.,1.86981398314345));
#27496=CARTESIAN_POINT('Ctrl Pts',(-0.765891519092557,-1.,1.86372027063314));
#27497=CARTESIAN_POINT('Ctrl Pts',(-0.765744212909305,-1.,1.85764741390391));
#27498=CARTESIAN_POINT('Ctrl Pts',(-0.765545710619023,-1.,1.85158945130054));
#27499=CARTESIAN_POINT('Ctrl Pts',(-0.765291664861971,-1.,1.8455369887591));
#27500=CARTESIAN_POINT('Ctrl Pts',(-0.764978057881687,-1.,1.83948181064823));
#27501=CARTESIAN_POINT('Ctrl Pts',(-0.764602549687845,-1.,1.8334207722714));
#27502=CARTESIAN_POINT('Ctrl Pts',(-0.764165902606055,-1.,1.8273599120008));
#27503=CARTESIAN_POINT('Ctrl Pts',(-0.763673465462854,-1.,1.82131873145297));
#27504=CARTESIAN_POINT('Ctrl Pts',(-0.763132003836783,-1.,1.81532118405566));
#27505=CARTESIAN_POINT('Ctrl Pts',(-0.762546129464036,-1.,1.80938551463989));
#27506=CARTESIAN_POINT('Ctrl Pts',(-0.761915336443516,-1.,1.80351583877334));
#27507=CARTESIAN_POINT('Ctrl Pts',(-0.761229695230359,-1.,1.79768986997735));
#27508=CARTESIAN_POINT('Ctrl Pts',(-0.760469555880425,-1.,1.79185815610802));
#27509=CARTESIAN_POINT('Ctrl Pts',(-0.759614401109868,-1.,1.78596964884526));
#27510=CARTESIAN_POINT('Ctrl Pts',(-0.75865062667738,-1.,1.77999411220912));
#27511=CARTESIAN_POINT('Ctrl Pts',(-0.757578264077238,-1.,1.77394167108342));
#27512=CARTESIAN_POINT('Ctrl Pts',(-0.756421896028403,-1.,1.76789396003141));
#27513=CARTESIAN_POINT('Ctrl Pts',(-0.755220979975262,-1.,1.7619781724032));
#27514=CARTESIAN_POINT('Ctrl Pts',(-0.75400925402848,-1.,1.75631083600175));
#27515=CARTESIAN_POINT('Ctrl Pts',(-0.752797683531377,-1.,1.75095139468809));
#27516=CARTESIAN_POINT('Ctrl Pts',(-0.751555614163629,-1.,1.74585086852298));
#27517=CARTESIAN_POINT('Ctrl Pts',(-0.75019343597954,-1.,1.74080458266705));
#27518=CARTESIAN_POINT('Ctrl Pts',(-0.748582462954855,-1.,1.73550351679848));
#27519=CARTESIAN_POINT('Ctrl Pts',(-0.746574710096436,-1.,1.72958533647399));
#27520=CARTESIAN_POINT('Ctrl Pts',(-0.744021445433764,-1.,1.7226822991693));
#27521=CARTESIAN_POINT('Ctrl Pts',(-0.740795162032088,-1.,1.71447789751927));
#27522=CARTESIAN_POINT('Ctrl Pts',(-0.736799665724771,-1.,1.70473309006121));
#27523=CARTESIAN_POINT('Ctrl Pts',(-0.731963238697195,-1.,1.69326921975743));
#27524=CARTESIAN_POINT('Ctrl Pts',(-0.726235967997433,-1.,1.67996158455503));
#27525=CARTESIAN_POINT('Ctrl Pts',(-0.719585433804282,-1.,1.6647288055568));
#27526=CARTESIAN_POINT('Ctrl Pts',(-0.711993139355394,-1.,1.64752408832016));
#27527=CARTESIAN_POINT('Ctrl Pts',(-0.705159151988319,-1.,1.63216541664676));
#27528=CARTESIAN_POINT('Ctrl Pts',(-0.699605146405088,-1.,1.61974673472612));
#27529=CARTESIAN_POINT('Ctrl Pts',(-0.695712097881194,-1.,1.61106790958151));
#27530=CARTESIAN_POINT('Ctrl Pts',(-0.693717979106306,-1.,1.60662857109684));
#27531=CARTESIAN_POINT('',(-0.892032620296855,-1.,1.5055822144029));
#27532=CARTESIAN_POINT('Origin',(0.,-1.,0.));
#27533=CARTESIAN_POINT('',(-1.23627494547115,-1.,1.81978687191668));
#27534=CARTESIAN_POINT('Ctrl Pts',(-0.892032620296855,-1.,1.5055822144029));
#27535=CARTESIAN_POINT('Ctrl Pts',(-0.894452006964543,-1.,1.50980486806688));
#27536=CARTESIAN_POINT('Ctrl Pts',(-0.899185047483511,-1.,1.51805569590094));
#27537=CARTESIAN_POINT('Ctrl Pts',(-0.905967409625651,-1.,1.52984849887993));
#27538=CARTESIAN_POINT('Ctrl Pts',(-0.914375919026456,-1.,1.54440491149498));
#27539=CARTESIAN_POINT('Ctrl Pts',(-0.923832188944341,-1.,1.56065988578893));
#27540=CARTESIAN_POINT('Ctrl Pts',(-0.932246680108685,-1.,1.57499388382243));
#27541=CARTESIAN_POINT('Ctrl Pts',(-0.939646377893399,-1.,1.58744937487176));
#27542=CARTESIAN_POINT('Ctrl Pts',(-0.946078063315257,-1.,1.59810042043673));
#27543=CARTESIAN_POINT('Ctrl Pts',(-0.951613284356035,-1.,1.60706069896936));
#27544=CARTESIAN_POINT('Ctrl Pts',(-0.956354422920671,-1.,1.61449324337085));
#27545=CARTESIAN_POINT('Ctrl Pts',(-0.960438326101729,-1.,1.62061638140221));
#27546=CARTESIAN_POINT('Ctrl Pts',(-0.964046107040536,-1.,1.62571930670187));
#27547=CARTESIAN_POINT('Ctrl Pts',(-0.967387853230345,-1.,1.63013849959461));
#27548=CARTESIAN_POINT('Ctrl Pts',(-0.970669715997509,-1.,1.63420665729798));
#27549=CARTESIAN_POINT('Ctrl Pts',(-0.974066058287418,-1.,1.63820952658144));
#27550=CARTESIAN_POINT('Ctrl Pts',(-0.977689794119416,-1.,1.64233990826687));
#27551=CARTESIAN_POINT('Ctrl Pts',(-0.981562530939489,-1.,1.64665139190656));
#27552=CARTESIAN_POINT('Ctrl Pts',(-0.985642622920821,-1.,1.65110016612638));
#27553=CARTESIAN_POINT('Ctrl Pts',(-0.989855627854165,-1.,1.65559044289699));
#27554=CARTESIAN_POINT('Ctrl Pts',(-0.994121836661306,-1.,1.66001553809947));
#27555=CARTESIAN_POINT('Ctrl Pts',(-0.998389654952758,-1.,1.66430758030376));
#27556=CARTESIAN_POINT('Ctrl Pts',(-1.00265091003727,-1.,1.66846059277303));
#27557=CARTESIAN_POINT('Ctrl Pts',(-1.00692206696414,-1.,1.67250335383293));
#27558=CARTESIAN_POINT('Ctrl Pts',(-1.01123236493511,-1.,1.67648246776464));
#27559=CARTESIAN_POINT('Ctrl Pts',(-1.01561026162773,-1.,1.68044289894798));
#27560=CARTESIAN_POINT('Ctrl Pts',(-1.02006795074201,-1.,1.68440578021706));
#27561=CARTESIAN_POINT('Ctrl Pts',(-1.02460180535255,-1.,1.68836910178447));
#27562=CARTESIAN_POINT('Ctrl Pts',(-1.02919977579147,-1.,1.69231840863458));
#27563=CARTESIAN_POINT('Ctrl Pts',(-1.03384646003588,-1.,1.69623414782771));
#27564=CARTESIAN_POINT('Ctrl Pts',(-1.03852922490789,-1.,1.70010052930962));
#27565=CARTESIAN_POINT('Ctrl Pts',(-1.04324363334554,-1.,1.70391338707982));
#27566=CARTESIAN_POINT('Ctrl Pts',(-1.04799085404995,-1.,1.70767646263649));
#27567=CARTESIAN_POINT('Ctrl Pts',(-1.05277517202855,-1.,1.71139783543989));
#27568=CARTESIAN_POINT('Ctrl Pts',(-1.05760163192479,-1.,1.7150865442702));
#27569=CARTESIAN_POINT('Ctrl Pts',(-1.06247324680647,-1.,1.71874858456904));
#27570=CARTESIAN_POINT('Ctrl Pts',(-1.06738966975462,-1.,1.72238500928453));
#27571=CARTESIAN_POINT('Ctrl Pts',(-1.07234866990252,-1.,1.72599406198488));
#27572=CARTESIAN_POINT('Ctrl Pts',(-1.0773470373727,-1.,1.72957248977424));
#27573=CARTESIAN_POINT('Ctrl Pts',(-1.08238162784749,-1.,1.73311705663407));
#27574=CARTESIAN_POINT('Ctrl Pts',(-1.08745056285427,-1.,1.73662628326091));
#27575=CARTESIAN_POINT('Ctrl Pts',(-1.09255329056493,-1.,1.74010053962247));
#27576=CARTESIAN_POINT('Ctrl Pts',(-1.09768999241225,-1.,1.74354119236208));
#27577=CARTESIAN_POINT('Ctrl Pts',(-1.10286118991143,-1.,1.74695004214923));
#27578=CARTESIAN_POINT('Ctrl Pts',(-1.10806728183007,-1.,1.7503286607592));
#27579=CARTESIAN_POINT('Ctrl Pts',(-1.11330807582551,-1.,1.7536777209463));
#27580=CARTESIAN_POINT('Ctrl Pts',(-1.11858293216763,-1.,1.75699720772105));
#27581=CARTESIAN_POINT('Ctrl Pts',(-1.12389096855086,-1.,1.76028671825096));
#27582=CARTESIAN_POINT('Ctrl Pts',(-1.12923123555075,-1.,1.7635457196617));
#27583=CARTESIAN_POINT('Ctrl Pts',(-1.1346029180462,-1.,1.76677384551862));
#27584=CARTESIAN_POINT('Ctrl Pts',(-1.14000548336975,-1.,1.76997111386769));
#27585=CARTESIAN_POINT('Ctrl Pts',(-1.1454385822692,-1.,1.77313777896194));
#27586=CARTESIAN_POINT('Ctrl Pts',(-1.15090197841515,-1.,1.7762742255701));
#27587=CARTESIAN_POINT('Ctrl Pts',(-1.15639547194698,-1.,1.77938085564275));
#27588=CARTESIAN_POINT('Ctrl Pts',(-1.16191881298499,-1.,1.78245795881009));
#27589=CARTESIAN_POINT('Ctrl Pts',(-1.16747166312303,-1.,1.78550566040443));
#27590=CARTESIAN_POINT('Ctrl Pts',(-1.17305363177328,-1.,1.78852398877616));
#27591=CARTESIAN_POINT('Ctrl Pts',(-1.17866429440809,-1.,1.79151291552689));
#27592=CARTESIAN_POINT('Ctrl Pts',(-1.18430321697432,-1.,1.79447240321515));
#27593=CARTESIAN_POINT('Ctrl Pts',(-1.18996997934445,-1.,1.79740245923478));
#27594=CARTESIAN_POINT('Ctrl Pts',(-1.19566418930242,-1.,1.80030314369879));
#27595=CARTESIAN_POINT('Ctrl Pts',(-1.20138548938974,-1.,1.80317454838603));
#27596=CARTESIAN_POINT('Ctrl Pts',(-1.20713356605475,-1.,1.80601678480707));
#27597=CARTESIAN_POINT('Ctrl Pts',(-1.21290815708314,-1.,1.80882996917129));
#27598=CARTESIAN_POINT('Ctrl Pts',(-1.21870906103557,-1.,1.81161420806656));
#27599=CARTESIAN_POINT('Ctrl Pts',(-1.2245361330495,-1.,1.81436959210434));
#27600=CARTESIAN_POINT('Ctrl Pts',(-1.2292186489137,-1.,1.8165508718364));
#27601=CARTESIAN_POINT('Ctrl Pts',(-1.2327422452705,-1.,1.81817389921279));
#27602=CARTESIAN_POINT('Ctrl Pts',(-1.23509651170476,-1.,1.81925017193666));
#27603=CARTESIAN_POINT('Ctrl Pts',(-1.23627494547115,-1.,1.81978687191668));
#27604=CARTESIAN_POINT('',(-1.34869019493419,-1.,1.73811241238545));
#27605=CARTESIAN_POINT('',(-1.23627494547115,-1.,1.81978687191668));
#27606=CARTESIAN_POINT('',(-1.15624053661742,-1.,1.31362392696032));
#27607=CARTESIAN_POINT('Ctrl Pts',(-1.34869019493419,-1.,1.73811241238545));
#27608=CARTESIAN_POINT('Ctrl Pts',(-1.34854391898045,-1.,1.73682580585691));
#27609=CARTESIAN_POINT('Ctrl Pts',(-1.34824783112887,-1.,1.73425417885907));
#27610=CARTESIAN_POINT('Ctrl Pts',(-1.34779309152035,-1.,1.7304014965394));
#27611=CARTESIAN_POINT('Ctrl Pts',(-1.34716554819527,-1.,1.72527410680674));
#27612=CARTESIAN_POINT('Ctrl Pts',(-1.34634568653227,-1.,1.7188807715049));
#27613=CARTESIAN_POINT('Ctrl Pts',(-1.34549029589416,-1.,1.71250340686822));
#27614=CARTESIAN_POINT('Ctrl Pts',(-1.34459924533831,-1.,1.70614212266738));
#27615=CARTESIAN_POINT('Ctrl Pts',(-1.34367237124483,-1.,1.69979707754427));
#27616=CARTESIAN_POINT('Ctrl Pts',(-1.34270948206319,-1.,1.6934684849687));
#27617=CARTESIAN_POINT('Ctrl Pts',(-1.341710374848,-1.,1.68715660868764));
#27618=CARTESIAN_POINT('Ctrl Pts',(-1.34067485185203,-1.,1.68086176030362));
#27619=CARTESIAN_POINT('Ctrl Pts',(-1.3396027347034,-1.,1.67458429426086));
#27620=CARTESIAN_POINT('Ctrl Pts',(-1.33849388654388,-1.,1.66832460783989));
#27621=CARTESIAN_POINT('Ctrl Pts',(-1.33734820885262,-1.,1.66208312541983));
#27622=CARTESIAN_POINT('Ctrl Pts',(-1.33616559745172,-1.,1.65586025952593));
#27623=CARTESIAN_POINT('Ctrl Pts',(-1.33494590467993,-1.,1.6496563728683));
#27624=CARTESIAN_POINT('Ctrl Pts',(-1.33368890676572,-1.,1.6434717485603));
#27625=CARTESIAN_POINT('Ctrl Pts',(-1.33239425103724,-1.,1.63730653475089));
#27626=CARTESIAN_POINT('Ctrl Pts',(-1.33106149345645,-1.,1.63116079730923));
#27627=CARTESIAN_POINT('Ctrl Pts',(-1.3296901950568,-1.,1.62503464209797));
#27628=CARTESIAN_POINT('Ctrl Pts',(-1.32828000610449,-1.,1.61892832270724));
#27629=CARTESIAN_POINT('Ctrl Pts',(-1.32683074483356,-1.,1.6128423401575));
#27630=CARTESIAN_POINT('Ctrl Pts',(-1.32534250785782,-1.,1.60677758290954));
#27631=CARTESIAN_POINT('Ctrl Pts',(-1.32381550858256,-1.,1.60073511858687));
#27632=CARTESIAN_POINT('Ctrl Pts',(-1.32224985747682,-1.,1.59471591079403));
#27633=CARTESIAN_POINT('Ctrl Pts',(-1.32064537110892,-1.,1.58872057258245));
#27634=CARTESIAN_POINT('Ctrl Pts',(-1.31900135021432,-1.,1.58274907898834));
#27635=CARTESIAN_POINT('Ctrl Pts',(-1.31731642317187,-1.,1.5768005650559));
#27636=CARTESIAN_POINT('Ctrl Pts',(-1.31558903860016,-1.,1.57087397835723));
#27637=CARTESIAN_POINT('Ctrl Pts',(-1.31381795281002,-1.,1.56496872402353));
#27638=CARTESIAN_POINT('Ctrl Pts',(-1.31200264341696,-1.,1.55908521254821));
#27639=CARTESIAN_POINT('Ctrl Pts',(-1.31014393684222,-1.,1.55322568759481));
#27640=CARTESIAN_POINT('Ctrl Pts',(-1.30824393907473,-1.,1.54739413957185));
#27641=CARTESIAN_POINT('Ctrl Pts',(-1.30630475189556,-1.,1.54159462645432));
#27642=CARTESIAN_POINT('Ctrl Pts',(-1.30432735639489,-1.,1.53582981268977));
#27643=CARTESIAN_POINT('Ctrl Pts',(-1.30231064395568,-1.,1.53009970283891));
#27644=CARTESIAN_POINT('Ctrl Pts',(-1.30024984366328,-1.,1.52439957861062));
#27645=CARTESIAN_POINT('Ctrl Pts',(-1.29813791800747,-1.,1.51872184912724));
#27646=CARTESIAN_POINT('Ctrl Pts',(-1.29596850710509,-1.,1.51305994241402));
#27647=CARTESIAN_POINT('Ctrl Pts',(-1.29373841372842,-1.,1.50741159078365));
#27648=CARTESIAN_POINT('Ctrl Pts',(-1.29145022885181,-1.,1.50178230149776));
#27649=CARTESIAN_POINT('Ctrl Pts',(-1.28911506584254,-1.,1.49618896881754));
#27650=CARTESIAN_POINT('Ctrl Pts',(-1.2867467611644,-1.,1.4906522831278));
#27651=CARTESIAN_POINT('Ctrl Pts',(-1.28435533880201,-1.,1.4851881711891));
#27652=CARTESIAN_POINT('Ctrl Pts',(-1.28194158939517,-1.,1.47980070347095));
#27653=CARTESIAN_POINT('Ctrl Pts',(-1.2794891824849,-1.,1.4744717526707));
#27654=CARTESIAN_POINT('Ctrl Pts',(-1.27696414831089,-1.,1.46916035917133));
#27655=CARTESIAN_POINT('Ctrl Pts',(-1.27433119897822,-1.,1.46382431332476));
#27656=CARTESIAN_POINT('Ctrl Pts',(-1.27156805265289,-1.,1.45843906294697));
#27657=CARTESIAN_POINT('Ctrl Pts',(-1.2686778680489,-1.,1.45301422764247));
#27658=CARTESIAN_POINT('Ctrl Pts',(-1.26570925118868,-1.,1.44761985001662));
#27659=CARTESIAN_POINT('Ctrl Pts',(-1.26273903323859,-1.,1.44236470511303));
#27660=CARTESIAN_POINT('Ctrl Pts',(-1.25983531012005,-1.,1.43734919180848));
#27661=CARTESIAN_POINT('Ctrl Pts',(-1.25702687965755,-1.,1.43262645609691));
#27662=CARTESIAN_POINT('Ctrl Pts',(-1.25426945222639,-1.,1.42815938799387));
#27663=CARTESIAN_POINT('Ctrl Pts',(-1.2514145557001,-1.,1.42378102115575));
#27664=CARTESIAN_POINT('Ctrl Pts',(-1.24824430986571,-1.,1.41923722596025));
#27665=CARTESIAN_POINT('Ctrl Pts',(-1.24450600513056,-1.,1.41422913175179));
#27666=CARTESIAN_POINT('Ctrl Pts',(-1.23994455029534,-1.,1.40845295531283));
#27667=CARTESIAN_POINT('Ctrl Pts',(-1.23434087290423,-1.,1.40164708206106));
#27668=CARTESIAN_POINT('Ctrl Pts',(-1.22752961899387,-1.,1.39361389568796));
#27669=CARTESIAN_POINT('Ctrl Pts',(-1.21938737280852,-1.,1.38420564527715));
#27670=CARTESIAN_POINT('Ctrl Pts',(-1.20982812925645,-1.,1.37331915607905));
#27671=CARTESIAN_POINT('Ctrl Pts',(-1.1987959077932,-1.,1.36088705043885));
#27672=CARTESIAN_POINT('Ctrl Pts',(-1.18625865667441,-1.,1.34687054001093));
#27673=CARTESIAN_POINT('Ctrl Pts',(-1.17501305789857,-1.,1.33437539347008));
#27674=CARTESIAN_POINT('Ctrl Pts',(-1.16589330093588,-1.,1.32428080721772));
#27675=CARTESIAN_POINT('Ctrl Pts',(-1.15950888730809,-1.,1.31722977216397));
#27676=CARTESIAN_POINT('Ctrl Pts',(-1.15624053661742,-1.,1.31362392696032));
#27677=CARTESIAN_POINT('',(-1.31362392696033,-1.,1.15624053661742));
#27678=CARTESIAN_POINT('Origin',(0.,-1.,0.));
#27679=CARTESIAN_POINT('',(-1.73811241238545,-1.,1.34869019493419));
#27680=CARTESIAN_POINT('Ctrl Pts',(-1.31362392696033,-1.,1.15624053661742));
#27681=CARTESIAN_POINT('Ctrl Pts',(-1.3172297721596,-1.,1.15950888730433));
#27682=CARTESIAN_POINT('Ctrl Pts',(-1.32428080720544,-1.,1.16589330092532));
#27683=CARTESIAN_POINT('Ctrl Pts',(-1.33437539344842,-1.,1.17501305787994));
#27684=CARTESIAN_POINT('Ctrl Pts',(-1.34687053998157,-1.,1.18625865664915));
#27685=CARTESIAN_POINT('Ctrl Pts',(-1.36088705040677,-1.,1.1987959077656));
#27686=CARTESIAN_POINT('Ctrl Pts',(-1.37331915604962,-1.,1.20982812923113));
#27687=CARTESIAN_POINT('Ctrl Pts',(-1.38420564525391,-1.,1.21938737278853));
#27688=CARTESIAN_POINT('Ctrl Pts',(-1.39361389567257,-1.,1.22752961898063));
#27689=CARTESIAN_POINT('Ctrl Pts',(-1.40164708205345,-1.,1.23434087289768));
#27690=CARTESIAN_POINT('Ctrl Pts',(-1.40845295531151,-1.,1.23994455029421));
#27691=CARTESIAN_POINT('Ctrl Pts',(-1.41422913175437,-1.,1.24450600513278));
#27692=CARTESIAN_POINT('Ctrl Pts',(-1.41923722596421,-1.,1.24824430986911));
#27693=CARTESIAN_POINT('Ctrl Pts',(-1.42378102115911,-1.,1.25141455570299));
#27694=CARTESIAN_POINT('Ctrl Pts',(-1.42815938799555,-1.,1.25426945222783));
#27695=CARTESIAN_POINT('Ctrl Pts',(-1.43262645609679,-1.,1.25702687965744));
#27696=CARTESIAN_POINT('Ctrl Pts',(-1.43734919180719,-1.,1.25983531011894));
#27697=CARTESIAN_POINT('Ctrl Pts',(-1.44236470511145,-1.,1.26273903323723));
#27698=CARTESIAN_POINT('Ctrl Pts',(-1.44761985001544,-1.,1.26570925118767));
#27699=CARTESIAN_POINT('Ctrl Pts',(-1.45301422764205,-1.,1.26867786804854));
#27700=CARTESIAN_POINT('Ctrl Pts',(-1.45843906294725,-1.,1.27156805265312));
#27701=CARTESIAN_POINT('Ctrl Pts',(-1.4638243133254,-1.,1.27433119897877));
#27702=CARTESIAN_POINT('Ctrl Pts',(-1.46916035917197,-1.,1.27696414831144));
#27703=CARTESIAN_POINT('Ctrl Pts',(-1.4744717526711,-1.,1.27948918248524));
#27704=CARTESIAN_POINT('Ctrl Pts',(-1.47980070347102,-1.,1.28194158939522));
#27705=CARTESIAN_POINT('Ctrl Pts',(-1.48518817118891,-1.,1.28435533880184));
#27706=CARTESIAN_POINT('Ctrl Pts',(-1.4906522831275,-1.,1.28674676116415));
#27707=CARTESIAN_POINT('Ctrl Pts',(-1.49618896881729,-1.,1.28911506584232));
#27708=CARTESIAN_POINT('Ctrl Pts',(-1.50178230149764,-1.,1.29145022885171));
#27709=CARTESIAN_POINT('Ctrl Pts',(-1.50741159078367,-1.,1.29373841372843));
#27710=CARTESIAN_POINT('Ctrl Pts',(-1.51305994241412,-1.,1.29596850710518));
#27711=CARTESIAN_POINT('Ctrl Pts',(-1.51872184912735,-1.,1.29813791800757));
#27712=CARTESIAN_POINT('Ctrl Pts',(-1.5243995786107,-1.,1.30024984366334));
#27713=CARTESIAN_POINT('Ctrl Pts',(-1.53009970283893,-1.,1.3023106439557));
#27714=CARTESIAN_POINT('Ctrl Pts',(-1.53582981268976,-1.,1.30432735639487));
#27715=CARTESIAN_POINT('Ctrl Pts',(-1.54159462645428,-1.,1.30630475189553));
#27716=CARTESIAN_POINT('Ctrl Pts',(-1.54739413957183,-1.,1.30824393907471));
#27717=CARTESIAN_POINT('Ctrl Pts',(-1.55322568759481,-1.,1.31014393684221));
#27718=CARTESIAN_POINT('Ctrl Pts',(-1.55908521254822,-1.,1.31200264341696));
#27719=CARTESIAN_POINT('Ctrl Pts',(-1.56496872402352,-1.,1.31381795281002));
#27720=CARTESIAN_POINT('Ctrl Pts',(-1.57087397835721,-1.,1.31558903860015));
#27721=CARTESIAN_POINT('Ctrl Pts',(-1.57680056505585,-1.,1.31731642317183));
#27722=CARTESIAN_POINT('Ctrl Pts',(-1.58274907898829,-1.,1.31900135021428));
#27723=CARTESIAN_POINT('Ctrl Pts',(-1.58872057258244,-1.,1.32064537110891));
#27724=CARTESIAN_POINT('Ctrl Pts',(-1.59471591079408,-1.,1.32224985747686));
#27725=CARTESIAN_POINT('Ctrl Pts',(-1.600735118587,-1.,1.32381550858266));
#27726=CARTESIAN_POINT('Ctrl Pts',(-1.6067775829097,-1.,1.32534250785794));
#27727=CARTESIAN_POINT('Ctrl Pts',(-1.61284234015762,-1.,1.32683074483365));
#27728=CARTESIAN_POINT('Ctrl Pts',(-1.61892832270723,-1.,1.32828000610448));
#27729=CARTESIAN_POINT('Ctrl Pts',(-1.62503464209777,-1.,1.32969019505665));
#27730=CARTESIAN_POINT('Ctrl Pts',(-1.63116079730887,-1.,1.33106149345618));
#27731=CARTESIAN_POINT('Ctrl Pts',(-1.6373065347505,-1.,1.33239425103694));
#27732=CARTESIAN_POINT('Ctrl Pts',(-1.64347174856007,-1.,1.33368890676554));
#27733=CARTESIAN_POINT('Ctrl Pts',(-1.64965637286843,-1.,1.33494590468003));
#27734=CARTESIAN_POINT('Ctrl Pts',(-1.65586025952651,-1.,1.33616559745217));
#27735=CARTESIAN_POINT('Ctrl Pts',(-1.66208312542073,-1.,1.33734820885331));
#27736=CARTESIAN_POINT('Ctrl Pts',(-1.66832460784078,-1.,1.33849388654458));
#27737=CARTESIAN_POINT('Ctrl Pts',(-1.67458429426126,-1.,1.33960273470372));
#27738=CARTESIAN_POINT('Ctrl Pts',(-1.68086176030308,-1.,1.3406748518516));
#27739=CARTESIAN_POINT('Ctrl Pts',(-1.68715660868602,-1.,1.34171037484673));
#27740=CARTESIAN_POINT('Ctrl Pts',(-1.6934684849664,-1.,1.34270948206139));
#27741=CARTESIAN_POINT('Ctrl Pts',(-1.69979707754221,-1.,1.34367237124322));
#27742=CARTESIAN_POINT('Ctrl Pts',(-1.70614212266676,-1.,1.34459924533783));
#27743=CARTESIAN_POINT('Ctrl Pts',(-1.71250340687011,-1.,1.34549029589563));
#27744=CARTESIAN_POINT('Ctrl Pts',(-1.7188807715095,-1.,1.34634568653586));
#27745=CARTESIAN_POINT('Ctrl Pts',(-1.72527410681298,-1.,1.34716554820013));
#27746=CARTESIAN_POINT('Ctrl Pts',(-1.73040149654497,-1.,1.3477930915247));
#27747=CARTESIAN_POINT('Ctrl Pts',(-1.73425417886255,-1.,1.34824783113158));
#27748=CARTESIAN_POINT('Ctrl Pts',(-1.73682580585819,-1.,1.34854391898145));
#27749=CARTESIAN_POINT('Ctrl Pts',(-1.73811241238545,-1.,1.34869019493419));
#27750=CARTESIAN_POINT('',(-1.81978687191668,-1.,1.23627494547115));
#27751=CARTESIAN_POINT('',(-1.73811241238545,-1.,1.34869019493419));
#27752=CARTESIAN_POINT('',(-1.5055822144029,-1.,0.892032620296855));
#27753=CARTESIAN_POINT('Ctrl Pts',(-1.81978687191668,-1.,1.23627494547115));
#27754=CARTESIAN_POINT('Ctrl Pts',(-1.81925017193531,-1.,1.23509651170384));
#27755=CARTESIAN_POINT('Ctrl Pts',(-1.81817389920914,-1.,1.23274224526804));
#27756=CARTESIAN_POINT('Ctrl Pts',(-1.81655087183054,-1.,1.22921864890975));
#27757=CARTESIAN_POINT('Ctrl Pts',(-1.81436959209778,-1.,1.22453613304507));
#27758=CARTESIAN_POINT('Ctrl Pts',(-1.81161420806172,-1.,1.2187090610323));
#27759=CARTESIAN_POINT('Ctrl Pts',(-1.80882996916931,-1.,1.2129081570818));
#27760=CARTESIAN_POINT('Ctrl Pts',(-1.80601678480772,-1.,1.20713356605519));
#27761=CARTESIAN_POINT('Ctrl Pts',(-1.8031745483882,-1.,1.2013854893912));
#27762=CARTESIAN_POINT('Ctrl Pts',(-1.80030314370121,-1.,1.19566418930405));
#27763=CARTESIAN_POINT('Ctrl Pts',(-1.79740245923649,-1.,1.1899699793456));
#27764=CARTESIAN_POINT('Ctrl Pts',(-1.79447240321572,-1.,1.18430321697471));
#27765=CARTESIAN_POINT('Ctrl Pts',(-1.79151291552646,-1.,1.17866429440781));
#27766=CARTESIAN_POINT('Ctrl Pts',(-1.78852398877523,-1.,1.17305363177265));
#27767=CARTESIAN_POINT('Ctrl Pts',(-1.78550566040349,-1.,1.16747166312239));
#27768=CARTESIAN_POINT('Ctrl Pts',(-1.78245795880949,-1.,1.16191881298458));
#27769=CARTESIAN_POINT('Ctrl Pts',(-1.77938085564261,-1.,1.15639547194689));
#27770=CARTESIAN_POINT('Ctrl Pts',(-1.77627422557034,-1.,1.15090197841531));
#27771=CARTESIAN_POINT('Ctrl Pts',(-1.77313777896234,-1.,1.14543858226948));
#27772=CARTESIAN_POINT('Ctrl Pts',(-1.76997111386806,-1.,1.14000548337));
#27773=CARTESIAN_POINT('Ctrl Pts',(-1.76677384551883,-1.,1.13460291804635));
#27774=CARTESIAN_POINT('Ctrl Pts',(-1.76354571966171,-1.,1.12923123555076));
#27775=CARTESIAN_POINT('Ctrl Pts',(-1.76028671825084,-1.,1.12389096855078));
#27776=CARTESIAN_POINT('Ctrl Pts',(-1.75699720772089,-1.,1.11858293216752));
#27777=CARTESIAN_POINT('Ctrl Pts',(-1.75367772094617,-1.,1.11330807582542));
#27778=CARTESIAN_POINT('Ctrl Pts',(-1.75032866075914,-1.,1.10806728183003));
#27779=CARTESIAN_POINT('Ctrl Pts',(-1.74695004214924,-1.,1.10286118991144));
#27780=CARTESIAN_POINT('Ctrl Pts',(-1.74354119236212,-1.,1.09768999241229));
#27781=CARTESIAN_POINT('Ctrl Pts',(-1.74010053962252,-1.,1.09255329056496));
#27782=CARTESIAN_POINT('Ctrl Pts',(-1.73662628326093,-1.,1.08745056285429));
#27783=CARTESIAN_POINT('Ctrl Pts',(-1.73311705663407,-1.,1.08238162784749));
#27784=CARTESIAN_POINT('Ctrl Pts',(-1.72957248977424,-1.,1.0773470373727));
#27785=CARTESIAN_POINT('Ctrl Pts',(-1.72599406198489,-1.,1.07234866990252));
#27786=CARTESIAN_POINT('Ctrl Pts',(-1.72238500928456,-1.,1.06738966975463));
#27787=CARTESIAN_POINT('Ctrl Pts',(-1.71874858456908,-1.,1.0624732468065));
#27788=CARTESIAN_POINT('Ctrl Pts',(-1.71508654427022,-1.,1.05760163192481));
#27789=CARTESIAN_POINT('Ctrl Pts',(-1.71139783543986,-1.,1.05277517202854));
#27790=CARTESIAN_POINT('Ctrl Pts',(-1.70767646263641,-1.,1.0479908540499));
#27791=CARTESIAN_POINT('Ctrl Pts',(-1.70391338707969,-1.,1.04324363334546));
#27792=CARTESIAN_POINT('Ctrl Pts',(-1.70010052930951,-1.,1.03852922490782));
#27793=CARTESIAN_POINT('Ctrl Pts',(-1.69623414782769,-1.,1.03384646003587));
#27794=CARTESIAN_POINT('Ctrl Pts',(-1.69231840863471,-1.,1.02919977579155));
#27795=CARTESIAN_POINT('Ctrl Pts',(-1.68836910178475,-1.,1.02460180535272));
#27796=CARTESIAN_POINT('Ctrl Pts',(-1.68440578021739,-1.,1.02006795074222));
#27797=CARTESIAN_POINT('Ctrl Pts',(-1.6804428989482,-1.,1.01561026162787));
#27798=CARTESIAN_POINT('Ctrl Pts',(-1.67648246776457,-1.,1.01123236493507));
#27799=CARTESIAN_POINT('Ctrl Pts',(-1.67250335383248,-1.,1.00692206696387));
#27800=CARTESIAN_POINT('Ctrl Pts',(-1.66846059277231,-1.,1.00265091003682));
#27801=CARTESIAN_POINT('Ctrl Pts',(-1.66430758030304,-1.,0.998389654952317));
#27802=CARTESIAN_POINT('Ctrl Pts',(-1.66001553809916,-1.,0.994121836661116));
#27803=CARTESIAN_POINT('Ctrl Pts',(-1.65559044289746,-1.,0.98985562785445));
#27804=CARTESIAN_POINT('Ctrl Pts',(-1.6511001661277,-1.,0.985642622921626));
#27805=CARTESIAN_POINT('Ctrl Pts',(-1.64665139190834,-1.,0.981562530940574));
#27806=CARTESIAN_POINT('Ctrl Pts',(-1.64233990826831,-1.,0.977689794120297));
#27807=CARTESIAN_POINT('Ctrl Pts',(-1.63820952658157,-1.,0.974066058287501));
#27808=CARTESIAN_POINT('Ctrl Pts',(-1.63420665729609,-1.,0.970669715996356));
#27809=CARTESIAN_POINT('Ctrl Pts',(-1.63013849959083,-1.,0.967387853228041));
#27810=CARTESIAN_POINT('Ctrl Pts',(-1.6257193066974,-1.,0.964046107037821));
#27811=CARTESIAN_POINT('Ctrl Pts',(-1.62061638139929,-1.,0.960438326099958));
#27812=CARTESIAN_POINT('Ctrl Pts',(-1.61449324337233,-1.,0.956354422921573));
#27813=CARTESIAN_POINT('Ctrl Pts',(-1.60706069897794,-1.,0.951613284361248));
#27814=CARTESIAN_POINT('Ctrl Pts',(-1.59810042045408,-1.,0.946078063325796));
#27815=CARTESIAN_POINT('Ctrl Pts',(-1.58744937489796,-1.,0.939646377909319));
#27816=CARTESIAN_POINT('Ctrl Pts',(-1.57499388385561,-1.,0.932246680128849));
#27817=CARTESIAN_POINT('Ctrl Pts',(-1.56065988582509,-1.,0.923832188966322));
#27818=CARTESIAN_POINT('Ctrl Pts',(-1.54440491152808,-1.,0.91437591904658));
#27819=CARTESIAN_POINT('Ctrl Pts',(-1.52984849890434,-1.,0.905967409640499));
#27820=CARTESIAN_POINT('Ctrl Pts',(-1.51805569591479,-1.,0.89918504749193));
#27821=CARTESIAN_POINT('Ctrl Pts',(-1.50980486807181,-1.,0.894452006967538));
#27822=CARTESIAN_POINT('Ctrl Pts',(-1.5055822144029,-1.,0.892032620296855));
#27823=CARTESIAN_POINT('',(-1.60662857109684,-1.,0.693717979106305));
#27824=CARTESIAN_POINT('Origin',(0.,-1.,0.));
#27825=CARTESIAN_POINT('',(-2.0698113262342,-1.,0.7455743247944));
#27826=CARTESIAN_POINT('Ctrl Pts',(-1.60662857109684,-1.,0.693717979106305));
#27827=CARTESIAN_POINT('Ctrl Pts',(-1.61106790957619,-1.,0.69571209787897));
#27828=CARTESIAN_POINT('Ctrl Pts',(-1.61974673471117,-1.,0.699605146398837));
#27829=CARTESIAN_POINT('Ctrl Pts',(-1.6321654166204,-1.,0.705159151977294));
#27830=CARTESIAN_POINT('Ctrl Pts',(-1.64752408828442,-1.,0.711993139340447));
#27831=CARTESIAN_POINT('Ctrl Pts',(-1.66472880551777,-1.,0.71958543378795));
#27832=CARTESIAN_POINT('Ctrl Pts',(-1.67996158451922,-1.,0.726235967982445));
#27833=CARTESIAN_POINT('Ctrl Pts',(-1.69326921972915,-1.,0.731963238685357));
#27834=CARTESIAN_POINT('Ctrl Pts',(-1.70473309004249,-1.,0.736799665716932));
#27835=CARTESIAN_POINT('Ctrl Pts',(-1.71447789751001,-1.,0.74079516202821));
#27836=CARTESIAN_POINT('Ctrl Pts',(-1.72268229916769,-1.,0.744021445433093));
#27837=CARTESIAN_POINT('Ctrl Pts',(-1.72958533647714,-1.,0.746574710097752));
#27838=CARTESIAN_POINT('Ctrl Pts',(-1.7355035168033,-1.,0.74858246295687));
#27839=CARTESIAN_POINT('Ctrl Pts',(-1.74080458267114,-1.,0.750193435981249));
#27840=CARTESIAN_POINT('Ctrl Pts',(-1.74585086852502,-1.,0.751555614164482));
#27841=CARTESIAN_POINT('Ctrl Pts',(-1.75095139468794,-1.,0.752797683531314));
#27842=CARTESIAN_POINT('Ctrl Pts',(-1.75631083600019,-1.,0.754009254027829));
#27843=CARTESIAN_POINT('Ctrl Pts',(-1.76197817240128,-1.,0.755220979974461));
#27844=CARTESIAN_POINT('Ctrl Pts',(-1.76789396002998,-1.,0.75642189602781));
#27845=CARTESIAN_POINT('Ctrl Pts',(-1.77394167108292,-1.,0.757578264077029));
#27846=CARTESIAN_POINT('Ctrl Pts',(-1.77999411220945,-1.,0.758650626677518));
#27847=CARTESIAN_POINT('Ctrl Pts',(-1.78596964884604,-1.,0.759614401110189));
#27848=CARTESIAN_POINT('Ctrl Pts',(-1.7918581561088,-1.,0.760469555880749));
#27849=CARTESIAN_POINT('Ctrl Pts',(-1.79768986997783,-1.,0.761229695230558));
#27850=CARTESIAN_POINT('Ctrl Pts',(-1.80351583877342,-1.,0.761915336443547));
#27851=CARTESIAN_POINT('Ctrl Pts',(-1.80938551463965,-1.,0.762546129463938));
#27852=CARTESIAN_POINT('Ctrl Pts',(-1.8153211840553,-1.,0.763132003836634));
#27853=CARTESIAN_POINT('Ctrl Pts',(-1.82131873145266,-1.,0.763673465462726));
#27854=CARTESIAN_POINT('Ctrl Pts',(-1.82735991200065,-1.,0.764165902605995));
#27855=CARTESIAN_POINT('Ctrl Pts',(-1.83342077227142,-1.,0.764602549687853));
#27856=CARTESIAN_POINT('Ctrl Pts',(-1.83948181064835,-1.,0.764978057881737));
#27857=CARTESIAN_POINT('Ctrl Pts',(-1.84553698875924,-1.,0.765291664862029));
#27858=CARTESIAN_POINT('Ctrl Pts',(-1.85158945130063,-1.,0.765545710619062));
#27859=CARTESIAN_POINT('Ctrl Pts',(-1.85764741390394,-1.,0.765744212909318));
#27860=CARTESIAN_POINT('Ctrl Pts',(-1.86372027063312,-1.,0.765891519092547));
#27861=CARTESIAN_POINT('Ctrl Pts',(-1.86981398314341,-1.,0.765990708546091));
#27862=CARTESIAN_POINT('Ctrl Pts',(-1.87592888967883,-1.,0.766042837036744));
#27863=CARTESIAN_POINT('Ctrl Pts',(-1.88206215302561,-1.,0.766047794851864));
#27864=CARTESIAN_POINT('Ctrl Pts',(-1.88820926433409,-1.,0.766004837062091));
#27865=CARTESIAN_POINT('Ctrl Pts',(-1.89436577771388,-1.,0.765913193856978));
#27866=CARTESIAN_POINT('Ctrl Pts',(-1.90052930393596,-1.,0.765772772593386));
#27867=CARTESIAN_POINT('Ctrl Pts',(-1.90669961402356,-1.,0.765584196937919));
#27868=CARTESIAN_POINT('Ctrl Pts',(-1.91287765805169,-1.,0.765348465884722));
#27869=CARTESIAN_POINT('Ctrl Pts',(-1.91906491634196,-1.,0.765066729667088));
#27870=CARTESIAN_POINT('Ctrl Pts',(-1.92526263537048,-1.,0.764740025488211));
#27871=CARTESIAN_POINT('Ctrl Pts',(-1.93147105496382,-1.,0.76436901067394));
#27872=CARTESIAN_POINT('Ctrl Pts',(-1.93768964875886,-1.,0.763954049121458));
#27873=CARTESIAN_POINT('Ctrl Pts',(-1.9439174661764,-1.,0.763495333538629));
#27874=CARTESIAN_POINT('Ctrl Pts',(-1.95015342590024,-1.,0.762992990878769));
#27875=CARTESIAN_POINT('Ctrl Pts',(-1.95639665309869,-1.,0.762447203806179));
#27876=CARTESIAN_POINT('Ctrl Pts',(-1.96264672744186,-1.,0.761858300014423));
#27877=CARTESIAN_POINT('Ctrl Pts',(-1.96890351582499,-1.,0.76122669048382));
#27878=CARTESIAN_POINT('Ctrl Pts',(-1.97516705321494,-1.,0.760552825409757));
#27879=CARTESIAN_POINT('Ctrl Pts',(-1.98143741418172,-1.,0.75983714745219));
#27880=CARTESIAN_POINT('Ctrl Pts',(-1.98771456680874,-1.,0.759080037802488));
#27881=CARTESIAN_POINT('Ctrl Pts',(-1.99399831098817,-1.,0.758281796766761));
#27882=CARTESIAN_POINT('Ctrl Pts',(-2.00028834739178,-1.,0.757442676862724));
#27883=CARTESIAN_POINT('Ctrl Pts',(-2.0065843158773,-1.,0.75656290464667));
#27884=CARTESIAN_POINT('Ctrl Pts',(-2.01288584328084,-1.,0.755642704957865));
#27885=CARTESIAN_POINT('Ctrl Pts',(-2.01919259405809,-1.,0.754682330722816));
#27886=CARTESIAN_POINT('Ctrl Pts',(-2.02550428623313,-1.,0.753682061112768));
#27887=CARTESIAN_POINT('Ctrl Pts',(-2.03182068456221,-1.,0.752642180487211));
#27888=CARTESIAN_POINT('Ctrl Pts',(-2.03814160092099,-1.,0.751562963361115));
#27889=CARTESIAN_POINT('Ctrl Pts',(-2.04446689147979,-1.,0.750444657875576));
#27890=CARTESIAN_POINT('Ctrl Pts',(-2.05079645592154,-1.,0.749287468665046));
#27891=CARTESIAN_POINT('Ctrl Pts',(-2.05713023031006,-1.,0.748091554183802));
#27892=CARTESIAN_POINT('Ctrl Pts',(-2.06220058927826,-1.,0.747103932787919));
#27893=CARTESIAN_POINT('Ctrl Pts',(-2.06600523016815,-1.,0.7463458715442));
#27894=CARTESIAN_POINT('Ctrl Pts',(-2.06854248895728,-1.,0.745832791378367));
#27895=CARTESIAN_POINT('Ctrl Pts',(-2.0698113262342,-1.,0.7455743247944));
#27896=CARTESIAN_POINT('',(-2.11275013067528,-1.,0.61342227326009));
#27897=CARTESIAN_POINT('',(-2.0698113262342,-1.,0.7455743247944));
#27898=CARTESIAN_POINT('',(-1.7075470150345,-1.,0.383122945602004));
#27899=CARTESIAN_POINT('Ctrl Pts',(-2.11275013067528,-1.,0.61342227326009));
#27900=CARTESIAN_POINT('Ctrl Pts',(-2.11187554259986,-1.,0.6124673655618));
#27901=CARTESIAN_POINT('Ctrl Pts',(-2.11012443807238,-1.,0.610560911689899));
#27902=CARTESIAN_POINT('Ctrl Pts',(-2.1074919961518,-1.,0.607711315454876));
#27903=CARTESIAN_POINT('Ctrl Pts',(-2.10397049886949,-1.,0.60393203073603));
#27904=CARTESIAN_POINT('Ctrl Pts',(-2.0995493086477,-1.,0.599241616420533));
#27905=CARTESIAN_POINT('Ctrl Pts',(-2.0951087622027,-1.,0.594585006052162));
#27906=CARTESIAN_POINT('Ctrl Pts',(-2.09064881812129,-1.,0.589962365403406));
#27907=CARTESIAN_POINT('Ctrl Pts',(-2.08616943727951,-1.,0.585373918991617));
#27908=CARTESIAN_POINT('Ctrl Pts',(-2.08167059018418,-1.,0.580819952108063));
#27909=CARTESIAN_POINT('Ctrl Pts',(-2.07715226767559,-1.,0.576300797416844));
#27910=CARTESIAN_POINT('Ctrl Pts',(-2.07261449292824,-1.,0.571816823242603));
#27911=CARTESIAN_POINT('Ctrl Pts',(-2.06805732997334,-1.,0.567368421181087));
#27912=CARTESIAN_POINT('Ctrl Pts',(-2.06348090160589,-1.,0.562955993082261));
#27913=CARTESIAN_POINT('Ctrl Pts',(-2.05888537756462,-1.,0.558579940185151));
#27914=CARTESIAN_POINT('Ctrl Pts',(-2.05427091604413,-1.,0.554240657463906));
#27915=CARTESIAN_POINT('Ctrl Pts',(-2.04963761077958,-1.,0.549938525150295));
#27916=CARTESIAN_POINT('Ctrl Pts',(-2.04498544714588,-1.,0.54567390381743));
#27917=CARTESIAN_POINT('Ctrl Pts',(-2.04031422690527,-1.,0.541447120615659));
#27918=CARTESIAN_POINT('Ctrl Pts',(-2.03562362954037,-1.,0.537258489833262));
#27919=CARTESIAN_POINT('Ctrl Pts',(-2.03091336214426,-1.,0.533108355132976));
#27920=CARTESIAN_POINT('Ctrl Pts',(-2.0261832908329,-1.,0.528997127241914));
#27921=CARTESIAN_POINT('Ctrl Pts',(-2.02143356304698,-1.,0.524925318333476));
#27922=CARTESIAN_POINT('Ctrl Pts',(-2.01666477917286,-1.,0.52089359039937));
#27923=CARTESIAN_POINT('Ctrl Pts',(-2.01187773939242,-1.,0.516902681728687));
#27924=CARTESIAN_POINT('Ctrl Pts',(-2.00707309946949,-1.,0.512953306961792));
#27925=CARTESIAN_POINT('Ctrl Pts',(-2.00225107134734,-1.,0.509046069886157));
#27926=CARTESIAN_POINT('Ctrl Pts',(-1.99741107463572,-1.,0.505181361323026));
#27927=CARTESIAN_POINT('Ctrl Pts',(-1.99255149126155,-1.,0.501359287727146));
#27928=CARTESIAN_POINT('Ctrl Pts',(-1.98767044752932,-1.,0.497579909545574));
#27929=CARTESIAN_POINT('Ctrl Pts',(-1.98276658761821,-1.,0.493843476541494));
#27930=CARTESIAN_POINT('Ctrl Pts',(-1.97783973019229,-1.,0.490150627860952));
#27931=CARTESIAN_POINT('Ctrl Pts',(-1.97289186263272,-1.,0.486502692907659));
#27932=CARTESIAN_POINT('Ctrl Pts',(-1.96792703422362,-1.,0.48290166212069));
#27933=CARTESIAN_POINT('Ctrl Pts',(-1.96294933055943,-1.,0.479349583074855));
#27934=CARTESIAN_POINT('Ctrl Pts',(-1.95796111148177,-1.,0.475848034683176));
#27935=CARTESIAN_POINT('Ctrl Pts',(-1.95296148278133,-1.,0.472397672264072));
#27936=CARTESIAN_POINT('Ctrl Pts',(-1.94794381136514,-1.,0.468997482913135));
#27937=CARTESIAN_POINT('Ctrl Pts',(-1.9428979419619,-1.,0.46564546202603));
#27938=CARTESIAN_POINT('Ctrl Pts',(-1.93781486640821,-1.,0.462340031009056));
#27939=CARTESIAN_POINT('Ctrl Pts',(-1.93269066517934,-1.,0.459081234547926));
#27940=CARTESIAN_POINT('Ctrl Pts',(-1.92753067150476,-1.,0.455872005174371));
#27941=CARTESIAN_POINT('Ctrl Pts',(-1.92235380648502,-1.,0.452719478359432));
#27942=CARTESIAN_POINT('Ctrl Pts',(-1.91718342555755,-1.,0.449632260106662));
#27943=CARTESIAN_POINT('Ctrl Pts',(-1.9120369998112,-1.,0.446617343485711));
#27944=CARTESIAN_POINT('Ctrl Pts',(-1.90691756144898,-1.,0.44367755684915));
#27945=CARTESIAN_POINT('Ctrl Pts',(-1.90180124389086,-1.,0.440807833704038));
#27946=CARTESIAN_POINT('Ctrl Pts',(-1.89663648956466,-1.,0.437995003948244));
#27947=CARTESIAN_POINT('Ctrl Pts',(-1.89136993975504,-1.,0.435225660963383));
#27948=CARTESIAN_POINT('Ctrl Pts',(-1.88596913666793,-1.,0.432493038548748));
#27949=CARTESIAN_POINT('Ctrl Pts',(-1.88044229001832,-1.,0.429803062482344));
#27950=CARTESIAN_POINT('Ctrl Pts',(-1.87486989291484,-1.,0.427183828519102));
#27951=CARTESIAN_POINT('Ctrl Pts',(-1.86937803944323,-1.,0.424678177291359));
#27952=CARTESIAN_POINT('Ctrl Pts',(-1.86408083334028,-1.,0.422327307418275));
#27953=CARTESIAN_POINT('Ctrl Pts',(-1.85903281096686,-1.,0.420157287975619));
#27954=CARTESIAN_POINT('Ctrl Pts',(-1.85417632856234,-1.,0.418164129143534));
#27955=CARTESIAN_POINT('Ctrl Pts',(-1.84929312929882,-1.,0.416300022038864));
#27956=CARTESIAN_POINT('Ctrl Pts',(-1.8440575707371,-1.,0.41448743825434));
#27957=CARTESIAN_POINT('Ctrl Pts',(-1.83808953475839,-1.,0.412633125322161));
#27958=CARTESIAN_POINT('Ctrl Pts',(-1.83100408895216,-1.,0.410641256301675));
#27959=CARTESIAN_POINT('Ctrl Pts',(-1.8224702267854,-1.,0.408428948108533));
#27960=CARTESIAN_POINT('Ctrl Pts',(-1.81223801813988,-1.,0.405933518411838));
#27961=CARTESIAN_POINT('Ctrl Pts',(-1.80012077176221,-1.,0.403107976170441));
#27962=CARTESIAN_POINT('Ctrl Pts',(-1.78598826347533,-1.,0.39991940378308));
#27963=CARTESIAN_POINT('Ctrl Pts',(-1.7697556004756,-1.,0.39634619612042));
#27964=CARTESIAN_POINT('Ctrl Pts',(-1.75137405313962,-1.,0.392375812294307));
#27965=CARTESIAN_POINT('Ctrl Pts',(-1.7349317097561,-1.,0.388877023509191));
#27966=CARTESIAN_POINT('Ctrl Pts',(-1.72162022246158,-1.,0.38607079032701));
#27967=CARTESIAN_POINT('Ctrl Pts',(-1.71231062891958,-1.,0.384119047315542));
#27968=CARTESIAN_POINT('Ctrl Pts',(-1.7075470150345,-1.,0.383122945602004));
#27969=CARTESIAN_POINT('',(-1.74236521665491,-1.,0.163289472382896));
#27970=CARTESIAN_POINT('Origin',(0.,-1.,0.));
#27971=CARTESIAN_POINT('',(-2.19890268624765,-1.,0.069476445021958));
#27972=CARTESIAN_POINT('Ctrl Pts',(-1.74236521665491,-1.,0.163289472382896));
#27973=CARTESIAN_POINT('Ctrl Pts',(-1.7472034950333,-1.,0.163814161002002));
#27974=CARTESIAN_POINT('Ctrl Pts',(-1.75666056638427,-1.,0.164834765707158));
#27975=CARTESIAN_POINT('Ctrl Pts',(-1.77018771684844,-1.,0.1662793551464));
#27976=CARTESIAN_POINT('Ctrl Pts',(-1.7869064998507,-1.,0.168032772805197));
#27977=CARTESIAN_POINT('Ctrl Pts',(-1.80561530629706,-1.,0.169936923904608));
#27978=CARTESIAN_POINT('Ctrl Pts',(-1.82215766811545,-1.,0.171554770204119));
#27979=CARTESIAN_POINT('Ctrl Pts',(-1.83658380527692,-1.,0.1728894428919));
#27980=CARTESIAN_POINT('Ctrl Pts',(-1.8489811319852,-1.,0.173946627587731));
#27981=CARTESIAN_POINT('Ctrl Pts',(-1.85948367088837,-1.,0.17473525927603));
#27982=CARTESIAN_POINT('Ctrl Pts',(-1.86828349694799,-1.,0.175268337590758));
#27983=CARTESIAN_POINT('Ctrl Pts',(-1.87563767773588,-1.,0.175563480746485));
#27984=CARTESIAN_POINT('Ctrl Pts',(-1.88188663145367,-1.,0.175644148889698));
#27985=CARTESIAN_POINT('Ctrl Pts',(-1.88742606273259,-1.,0.175538155840648));
#27986=CARTESIAN_POINT('Ctrl Pts',(-1.892646301985,-1.,0.175274276190844));
#27987=CARTESIAN_POINT('Ctrl Pts',(-1.89788101117132,-1.,0.174879405091263));
#27988=CARTESIAN_POINT('Ctrl Pts',(-1.90335253862834,-1.,0.174375518661085));
#27989=CARTESIAN_POINT('Ctrl Pts',(-1.90911693975267,-1.,0.173776635257817));
#27990=CARTESIAN_POINT('Ctrl Pts',(-1.91511429159527,-1.,0.173090695383496));
#27991=CARTESIAN_POINT('Ctrl Pts',(-1.9212233439798,-1.,0.172321621259514));
#27992=CARTESIAN_POINT('Ctrl Pts',(-1.92731093582036,-1.,0.171471191532988));
#27993=CARTESIAN_POINT('Ctrl Pts',(-1.93329183155539,-1.,0.170541253116201));
#27994=CARTESIAN_POINT('Ctrl Pts',(-1.93915639211581,-1.,0.169534904817491));
#27995=CARTESIAN_POINT('Ctrl Pts',(-1.94493757756931,-1.,0.168455741607556));
#27996=CARTESIAN_POINT('Ctrl Pts',(-1.95069027794294,-1.,0.167307501784475));
#27997=CARTESIAN_POINT('Ctrl Pts',(-1.9564675971873,-1.,0.166093592002812));
#27998=CARTESIAN_POINT('Ctrl Pts',(-1.96229379940136,-1.,0.164816568920269));
#27999=CARTESIAN_POINT('Ctrl Pts',(-1.96816512677967,-1.,0.163478185457734));
#28000=CARTESIAN_POINT('Ctrl Pts',(-1.97406280235188,-1.,0.162079693556288));
#28001=CARTESIAN_POINT('Ctrl Pts',(-1.97996195437559,-1.,0.160622060784611));
#28002=CARTESIAN_POINT('Ctrl Pts',(-1.98584238283292,-1.,0.159106226437299));
#28003=CARTESIAN_POINT('Ctrl Pts',(-1.99169810931908,-1.,0.157533331459227));
#28004=CARTESIAN_POINT('Ctrl Pts',(-1.99753284771497,-1.,0.155904629548783));
#28005=CARTESIAN_POINT('Ctrl Pts',(-2.00335565310543,-1.,0.154221403049722));
#28006=CARTESIAN_POINT('Ctrl Pts',(-2.00917680318424,-1.,0.15248488362145));
#28007=CARTESIAN_POINT('Ctrl Pts',(-2.01500291940238,-1.,0.150696157673078));
#28008=CARTESIAN_POINT('Ctrl Pts',(-2.02083464969894,-1.,0.148856124775337));
#28009=CARTESIAN_POINT('Ctrl Pts',(-2.02666926182017,-1.,0.146965557332583));
#28010=CARTESIAN_POINT('Ctrl Pts',(-2.03250223739942,-1.,0.145025140186057));
#28011=CARTESIAN_POINT('Ctrl Pts',(-2.03832911025912,-1.,0.143035515058209));
#28012=CARTESIAN_POINT('Ctrl Pts',(-2.04414757947916,-1.,0.140997332152546));
#28013=CARTESIAN_POINT('Ctrl Pts',(-2.04995762001328,-1.,0.138911255368966));
#28014=CARTESIAN_POINT('Ctrl Pts',(-2.05576044414264,-1.,0.136777941218043));
#28015=CARTESIAN_POINT('Ctrl Pts',(-2.06155781517842,-1.,0.134598026192106));
#28016=CARTESIAN_POINT('Ctrl Pts',(-2.06735123910326,-1.,0.13237211154771));
#28017=CARTESIAN_POINT('Ctrl Pts',(-2.07314114713063,-1.,0.130100748328403));
#28018=CARTESIAN_POINT('Ctrl Pts',(-2.07892715110987,-1.,0.12778444527612));
#28019=CARTESIAN_POINT('Ctrl Pts',(-2.08470840653643,-1.,0.125423679412061));
#28020=CARTESIAN_POINT('Ctrl Pts',(-2.09048392424825,-1.,0.123018905621083));
#28021=CARTESIAN_POINT('Ctrl Pts',(-2.0962529286773,-1.,0.120570567965122));
#28022=CARTESIAN_POINT('Ctrl Pts',(-2.102015121329,-1.,0.118079107988355));
#28023=CARTESIAN_POINT('Ctrl Pts',(-2.10777050261309,-1.,0.115544957687926));
#28024=CARTESIAN_POINT('Ctrl Pts',(-2.11351924490306,-1.,0.112968534419737));
#28025=CARTESIAN_POINT('Ctrl Pts',(-2.11926155590865,-1.,0.110350236135025));
#28026=CARTESIAN_POINT('Ctrl Pts',(-2.12499752307,-1.,0.10769043523109));
#28027=CARTESIAN_POINT('Ctrl Pts',(-2.13072704887293,-1.,0.104989479152739));
#28028=CARTESIAN_POINT('Ctrl Pts',(-2.13644992667165,-1.,0.1022477005561));
#28029=CARTESIAN_POINT('Ctrl Pts',(-2.14216588396025,-1.,0.0994654261990914));
#28030=CARTESIAN_POINT('Ctrl Pts',(-2.14787463531795,-1.,0.0966429852305457));
#28031=CARTESIAN_POINT('Ctrl Pts',(-2.1535759397817,-1.,0.0937807218867642));
#28032=CARTESIAN_POINT('Ctrl Pts',(-2.15926961544516,-1.,0.0908789888107264));
#28033=CARTESIAN_POINT('Ctrl Pts',(-2.16495552645014,-1.,0.0879381291386921));
#28034=CARTESIAN_POINT('Ctrl Pts',(-2.17063357870952,-1.,0.0849584620835371));
#28035=CARTESIAN_POINT('Ctrl Pts',(-2.176303712113,-1.,0.0819402680872764));
#28036=CARTESIAN_POINT('Ctrl Pts',(-2.18196589448887,-1.,0.0788837727685241));
#28037=CARTESIAN_POINT('Ctrl Pts',(-2.1876201139953,-1.,0.0757891465836146));
#28038=CARTESIAN_POINT('Ctrl Pts',(-2.19213712013662,-1.,0.0732830357306724));
#28039=CARTESIAN_POINT('Ctrl Pts',(-2.19552129484002,-1.,0.0713863779526153));
#28040=CARTESIAN_POINT('Ctrl Pts',(-2.19777582085423,-1.,0.0701143536325489));
#28041=CARTESIAN_POINT('Ctrl Pts',(-2.19890268624765,-1.,0.069476445021958));
#28042=CARTESIAN_POINT('',(-2.19890268624765,-1.,-0.0694764450219585));
#28043=CARTESIAN_POINT('',(-2.19890268624765,-1.,0.069476445021958));
#28044=CARTESIAN_POINT('',(-1.74236521665491,-1.,-0.163289472382896));
#28045=CARTESIAN_POINT('Ctrl Pts',(-2.19890268624765,-1.,-0.0694764450219585));
#28046=CARTESIAN_POINT('Ctrl Pts',(-2.19777582085261,-1.,-0.0701143536324927));
#28047=CARTESIAN_POINT('Ctrl Pts',(-2.19552129483562,-1.,-0.0713863779524629));
#28048=CARTESIAN_POINT('Ctrl Pts',(-2.19213712012956,-1.,-0.0732830357304277));
#28049=CARTESIAN_POINT('Ctrl Pts',(-2.1876201139874,-1.,-0.0757891465833413));
#28050=CARTESIAN_POINT('Ctrl Pts',(-2.18196589448304,-1.,-0.0788837727683229));
#28051=CARTESIAN_POINT('Ctrl Pts',(-2.1763037121106,-1.,-0.0819402680871941));
#28052=CARTESIAN_POINT('Ctrl Pts',(-2.17063357871031,-1.,-0.0849584620835644));
#28053=CARTESIAN_POINT('Ctrl Pts',(-2.16495552645275,-1.,-0.0879381291387824));
#28054=CARTESIAN_POINT('Ctrl Pts',(-2.15926961544808,-1.,-0.0908789888108267));
#28055=CARTESIAN_POINT('Ctrl Pts',(-2.15357593978377,-1.,-0.0937807218868346));
#28056=CARTESIAN_POINT('Ctrl Pts',(-2.14787463531864,-1.,-0.096642985230569));
#28057=CARTESIAN_POINT('Ctrl Pts',(-2.14216588395974,-1.,-0.0994654261990744));
#28058=CARTESIAN_POINT('Ctrl Pts',(-2.13644992667052,-1.,-0.102247700556064));
#28059=CARTESIAN_POINT('Ctrl Pts',(-2.1307270488718,-1.,-0.104989479152703));
#28060=CARTESIAN_POINT('Ctrl Pts',(-2.12499752306927,-1.,-0.107690435231068));
#28061=CARTESIAN_POINT('Ctrl Pts',(-2.11926155590849,-1.,-0.11035023613502));
#28062=CARTESIAN_POINT('Ctrl Pts',(-2.11351924490335,-1.,-0.112968534419746));
#28063=CARTESIAN_POINT('Ctrl Pts',(-2.10777050261359,-1.,-0.11554495768794));
#28064=CARTESIAN_POINT('Ctrl Pts',(-2.10201512132945,-1.,-0.118079107988368));
#28065=CARTESIAN_POINT('Ctrl Pts',(-2.09625292867756,-1.,-0.120570567965129));
#28066=CARTESIAN_POINT('Ctrl Pts',(-2.09048392424826,-1.,-0.123018905621083));
#28067=CARTESIAN_POINT('Ctrl Pts',(-2.08470840653628,-1.,-0.125423679412058));
#28068=CARTESIAN_POINT('Ctrl Pts',(-2.07892715110967,-1.,-0.127784445276116));
#28069=CARTESIAN_POINT('Ctrl Pts',(-2.07314114713047,-1.,-0.130100748328401));
#28070=CARTESIAN_POINT('Ctrl Pts',(-2.06735123910319,-1.,-0.13237211154771));
#28071=CARTESIAN_POINT('Ctrl Pts',(-2.06155781517844,-1.,-0.134598026192107));
#28072=CARTESIAN_POINT('Ctrl Pts',(-2.0557604441427,-1.,-0.136777941218044));
#28073=CARTESIAN_POINT('Ctrl Pts',(-2.04995762001333,-1.,-0.138911255368966));
#28074=CARTESIAN_POINT('Ctrl Pts',(-2.04414757947919,-1.,-0.140997332152545));
#28075=CARTESIAN_POINT('Ctrl Pts',(-2.03832911025913,-1.,-0.143035515058208));
#28076=CARTESIAN_POINT('Ctrl Pts',(-2.03250223739941,-1.,-0.145025140186058));
#28077=CARTESIAN_POINT('Ctrl Pts',(-2.02666926182017,-1.,-0.146965557332586));
#28078=CARTESIAN_POINT('Ctrl Pts',(-2.02083464969897,-1.,-0.148856124775343));
#28079=CARTESIAN_POINT('Ctrl Pts',(-2.01500291940243,-1.,-0.150696157673084));
#28080=CARTESIAN_POINT('Ctrl Pts',(-2.00917680318426,-1.,-0.152484883621452));
#28081=CARTESIAN_POINT('Ctrl Pts',(-2.00335565310539,-1.,-0.154221403049719));
#28082=CARTESIAN_POINT('Ctrl Pts',(-1.99753284771487,-1.,-0.155904629548775));
#28083=CARTESIAN_POINT('Ctrl Pts',(-1.99169810931893,-1.,-0.157533331459215));
#28084=CARTESIAN_POINT('Ctrl Pts',(-1.98584238283279,-1.,-0.159106226437289));
#28085=CARTESIAN_POINT('Ctrl Pts',(-1.97996195437557,-1.,-0.16062206078461));
#28086=CARTESIAN_POINT('Ctrl Pts',(-1.97406280235204,-1.,-0.162079693556302));
#28087=CARTESIAN_POINT('Ctrl Pts',(-1.96816512678,-1.,-0.16347818545776));
#28088=CARTESIAN_POINT('Ctrl Pts',(-1.96229379940174,-1.,-0.1648165689203));
#28089=CARTESIAN_POINT('Ctrl Pts',(-1.95646759718755,-1.,-0.166093592002833));
#28090=CARTESIAN_POINT('Ctrl Pts',(-1.95069027794286,-1.,-0.167307501784469));
#28091=CARTESIAN_POINT('Ctrl Pts',(-1.94493757756879,-1.,-0.168455741607516));
#28092=CARTESIAN_POINT('Ctrl Pts',(-1.93915639211497,-1.,-0.169534904817425));
#28093=CARTESIAN_POINT('Ctrl Pts',(-1.93329183155455,-1.,-0.170541253116136));
#28094=CARTESIAN_POINT('Ctrl Pts',(-1.92731093582,-1.,-0.17147119153296));
#28095=CARTESIAN_POINT('Ctrl Pts',(-1.92122334398034,-1.,-0.172321621259557));
#28096=CARTESIAN_POINT('Ctrl Pts',(-1.91511429159681,-1.,-0.173090695383619));
#28097=CARTESIAN_POINT('Ctrl Pts',(-1.90911693975475,-1.,-0.173776635257984));
#28098=CARTESIAN_POINT('Ctrl Pts',(-1.90335253863003,-1.,-0.174375518661222));
#28099=CARTESIAN_POINT('Ctrl Pts',(-1.89788101117148,-1.,-0.174879405091277));
#28100=CARTESIAN_POINT('Ctrl Pts',(-1.89264630198279,-1.,-0.175274276190664));
#28101=CARTESIAN_POINT('Ctrl Pts',(-1.88742606272818,-1.,-0.175538155840286));
#28102=CARTESIAN_POINT('Ctrl Pts',(-1.88188663144846,-1.,-0.175644148889271));
#28103=CARTESIAN_POINT('Ctrl Pts',(-1.87563767773249,-1.,-0.175563480746205));
#28104=CARTESIAN_POINT('Ctrl Pts',(-1.86828349694972,-1.,-0.175268337590901));
#28105=CARTESIAN_POINT('Ctrl Pts',(-1.85948367089838,-1.,-0.174735259276856));
#28106=CARTESIAN_POINT('Ctrl Pts',(-1.84898113200543,-1.,-0.173946627589401));
#28107=CARTESIAN_POINT('Ctrl Pts',(-1.83658380530747,-1.,-0.17288944289442));
#28108=CARTESIAN_POINT('Ctrl Pts',(-1.82215766815414,-1.,-0.171554770207306));
#28109=CARTESIAN_POINT('Ctrl Pts',(-1.80561530633924,-1.,-0.169936923908078));
#28110=CARTESIAN_POINT('Ctrl Pts',(-1.78690649988931,-1.,-0.16803277280837));
#28111=CARTESIAN_POINT('Ctrl Pts',(-1.77018771687692,-1.,-0.166279355148738));
#28112=CARTESIAN_POINT('Ctrl Pts',(-1.75666056640041,-1.,-0.164834765708484));
#28113=CARTESIAN_POINT('Ctrl Pts',(-1.74720349503904,-1.,-0.163814161002474));
#28114=CARTESIAN_POINT('Ctrl Pts',(-1.74236521665491,-1.,-0.163289472382896));
#28115=CARTESIAN_POINT('',(-1.7075470150345,-1.,-0.383122945602004));
#28116=CARTESIAN_POINT('Origin',(0.,-1.,0.));
#28117=CARTESIAN_POINT('',(-2.11275013067528,-1.,-0.61342227326009));
#28118=CARTESIAN_POINT('Ctrl Pts',(-1.7075470150345,-1.,-0.383122945602004));
#28119=CARTESIAN_POINT('Ctrl Pts',(-1.71231062891398,-1.,-0.384119047314215));
#28120=CARTESIAN_POINT('Ctrl Pts',(-1.72162022244582,-1.,-0.386070790323281));
#28121=CARTESIAN_POINT('Ctrl Pts',(-1.73493170972829,-1.,-0.388877023502615));
#28122=CARTESIAN_POINT('Ctrl Pts',(-1.75137405310193,-1.,-0.392375812285395));
#28123=CARTESIAN_POINT('Ctrl Pts',(-1.76975560043442,-1.,-0.396346196110688));
#28124=CARTESIAN_POINT('Ctrl Pts',(-1.78598826343754,-1.,-0.399919403774155));
#28125=CARTESIAN_POINT('Ctrl Pts',(-1.80012077173238,-1.,-0.403107976163396));
#28126=CARTESIAN_POINT('Ctrl Pts',(-1.81223801812013,-1.,-0.405933518407175));
#28127=CARTESIAN_POINT('Ctrl Pts',(-1.82247022677562,-1.,-0.408428948106227));
#28128=CARTESIAN_POINT('Ctrl Pts',(-1.83100408895047,-1.,-0.410641256301276));
#28129=CARTESIAN_POINT('Ctrl Pts',(-1.8380895347617,-1.,-0.412633125322945));
#28130=CARTESIAN_POINT('Ctrl Pts',(-1.84405757074218,-1.,-0.414487438255542));
#28131=CARTESIAN_POINT('Ctrl Pts',(-1.84929312930314,-1.,-0.416300022039885));
#28132=CARTESIAN_POINT('Ctrl Pts',(-1.8541763285645,-1.,-0.418164129144045));
#28133=CARTESIAN_POINT('Ctrl Pts',(-1.8590328109667,-1.,-0.420157287975583));
#28134=CARTESIAN_POINT('Ctrl Pts',(-1.86408083333863,-1.,-0.422327307417884));
#28135=CARTESIAN_POINT('Ctrl Pts',(-1.8693780394412,-1.,-0.424678177290876));
#28136=CARTESIAN_POINT('Ctrl Pts',(-1.87486989291333,-1.,-0.427183828518743));
#28137=CARTESIAN_POINT('Ctrl Pts',(-1.88044229001778,-1.,-0.429803062482217));
#28138=CARTESIAN_POINT('Ctrl Pts',(-1.88596913666828,-1.,-0.432493038548833));
#28139=CARTESIAN_POINT('Ctrl Pts',(-1.89136993975585,-1.,-0.43522566096358));
#28140=CARTESIAN_POINT('Ctrl Pts',(-1.89663648956549,-1.,-0.437995003948443));
#28141=CARTESIAN_POINT('Ctrl Pts',(-1.90180124389137,-1.,-0.44080783370416));
#28142=CARTESIAN_POINT('Ctrl Pts',(-1.90691756144906,-1.,-0.44367755684917));
#28143=CARTESIAN_POINT('Ctrl Pts',(-1.91203699981095,-1.,-0.446617343485651));
#28144=CARTESIAN_POINT('Ctrl Pts',(-1.91718342555717,-1.,-0.449632260106572));
#28145=CARTESIAN_POINT('Ctrl Pts',(-1.9223538064847,-1.,-0.452719478359356));
#28146=CARTESIAN_POINT('Ctrl Pts',(-1.92753067150461,-1.,-0.455872005174335));
#28147=CARTESIAN_POINT('Ctrl Pts',(-1.93269066517936,-1.,-0.459081234547931));
#28148=CARTESIAN_POINT('Ctrl Pts',(-1.93781486640834,-1.,-0.462340031009087));
#28149=CARTESIAN_POINT('Ctrl Pts',(-1.94289794196205,-1.,-0.465645462026064));
#28150=CARTESIAN_POINT('Ctrl Pts',(-1.94794381136524,-1.,-0.468997482913158));
#28151=CARTESIAN_POINT('Ctrl Pts',(-1.95296148278136,-1.,-0.472397672264079));
#28152=CARTESIAN_POINT('Ctrl Pts',(-1.95796111148175,-1.,-0.475848034683171));
#28153=CARTESIAN_POINT('Ctrl Pts',(-1.96294933055938,-1.,-0.479349583074846));
#28154=CARTESIAN_POINT('Ctrl Pts',(-1.96792703422358,-1.,-0.482901662120686));
#28155=CARTESIAN_POINT('Ctrl Pts',(-1.97289186263272,-1.,-0.486502692907661));
#28156=CARTESIAN_POINT('Ctrl Pts',(-1.97783973019229,-1.,-0.490150627860955));
#28157=CARTESIAN_POINT('Ctrl Pts',(-1.9827665876182,-1.,-0.493843476541492));
#28158=CARTESIAN_POINT('Ctrl Pts',(-1.98767044752929,-1.,-0.497579909545564));
#28159=CARTESIAN_POINT('Ctrl Pts',(-1.9925514912615,-1.,-0.501359287727129));
#28160=CARTESIAN_POINT('Ctrl Pts',(-1.99741107463567,-1.,-0.505181361323011));
#28161=CARTESIAN_POINT('Ctrl Pts',(-2.00225107134733,-1.,-0.509046069886152));
#28162=CARTESIAN_POINT('Ctrl Pts',(-2.00707309946955,-1.,-0.512953306961813));
#28163=CARTESIAN_POINT('Ctrl Pts',(-2.01187773939257,-1.,-0.516902681728733));
#28164=CARTESIAN_POINT('Ctrl Pts',(-2.01666477917305,-1.,-0.520893590399428));
#28165=CARTESIAN_POINT('Ctrl Pts',(-2.02143356304712,-1.,-0.524925318333518));
#28166=CARTESIAN_POINT('Ctrl Pts',(-2.02618329083289,-1.,-0.52899712724191));
#28167=CARTESIAN_POINT('Ctrl Pts',(-2.03091336214401,-1.,-0.533108355132905));
#28168=CARTESIAN_POINT('Ctrl Pts',(-2.03562362953993,-1.,-0.537258489833134));
#28169=CARTESIAN_POINT('Ctrl Pts',(-2.0403142269048,-1.,-0.54144712061552));
#28170=CARTESIAN_POINT('Ctrl Pts',(-2.0449854471456,-1.,-0.545673903817348));
#28171=CARTESIAN_POINT('Ctrl Pts',(-2.04963761077974,-1.,-0.549938525150342));
#28172=CARTESIAN_POINT('Ctrl Pts',(-2.05427091604482,-1.,-0.554240657464109));
#28173=CARTESIAN_POINT('Ctrl Pts',(-2.05888537756571,-1.,-0.558579940185467));
#28174=CARTESIAN_POINT('Ctrl Pts',(-2.06348090160697,-1.,-0.562955993082574));
#28175=CARTESIAN_POINT('Ctrl Pts',(-2.06805732997383,-1.,-0.567368421181229));
#28176=CARTESIAN_POINT('Ctrl Pts',(-2.07261449292757,-1.,-0.571816823242411));
#28177=CARTESIAN_POINT('Ctrl Pts',(-2.07715226767361,-1.,-0.576300797416274));
#28178=CARTESIAN_POINT('Ctrl Pts',(-2.08167059018138,-1.,-0.580819952107257));
#28179=CARTESIAN_POINT('Ctrl Pts',(-2.086169437277,-1.,-0.585373918990895));
#28180=CARTESIAN_POINT('Ctrl Pts',(-2.09064881812053,-1.,-0.589962365403189));
#28181=CARTESIAN_POINT('Ctrl Pts',(-2.09510876220501,-1.,-0.594585006052823));
#28182=CARTESIAN_POINT('Ctrl Pts',(-2.09954930865331,-1.,-0.599241616422144));
#28183=CARTESIAN_POINT('Ctrl Pts',(-2.10397049887709,-1.,-0.603932030738212));
#28184=CARTESIAN_POINT('Ctrl Pts',(-2.10749199615859,-1.,-0.607711315456826));
#28185=CARTESIAN_POINT('Ctrl Pts',(-2.11012443807661,-1.,-0.610560911691113));
#28186=CARTESIAN_POINT('Ctrl Pts',(-2.11187554260142,-1.,-0.61246736556225));
#28187=CARTESIAN_POINT('Ctrl Pts',(-2.11275013067528,-1.,-0.61342227326009));
#28188=CARTESIAN_POINT('',(-2.0698113262342,-1.,-0.745574324794401));
#28189=CARTESIAN_POINT('',(-2.11275013067528,-1.,-0.61342227326009));
#28190=CARTESIAN_POINT('',(-1.60662857109684,-1.,-0.693717979106306));
#28191=CARTESIAN_POINT('Ctrl Pts',(-2.0698113262342,-1.,-0.745574324794401));
#28192=CARTESIAN_POINT('Ctrl Pts',(-2.06854248895575,-1.,-0.74583279137781));
#28193=CARTESIAN_POINT('Ctrl Pts',(-2.06600523016401,-1.,-0.746345871542695));
#28194=CARTESIAN_POINT('Ctrl Pts',(-2.06220058927162,-1.,-0.747103932785504));
#28195=CARTESIAN_POINT('Ctrl Pts',(-2.05713023030263,-1.,-0.748091554181101));
#28196=CARTESIAN_POINT('Ctrl Pts',(-2.05079645591606,-1.,-0.749287468663053));
#28197=CARTESIAN_POINT('Ctrl Pts',(-2.04446689147754,-1.,-0.750444657874758));
#28198=CARTESIAN_POINT('Ctrl Pts',(-2.03814160092173,-1.,-0.751562963361383));
#28199=CARTESIAN_POINT('Ctrl Pts',(-2.03182068456467,-1.,-0.752642180488104));
#28200=CARTESIAN_POINT('Ctrl Pts',(-2.02550428623587,-1.,-0.753682061113765));
#28201=CARTESIAN_POINT('Ctrl Pts',(-2.01919259406003,-1.,-0.75468233072352));
#28202=CARTESIAN_POINT('Ctrl Pts',(-2.01288584328149,-1.,-0.7556427049581));
#28203=CARTESIAN_POINT('Ctrl Pts',(-2.00658431587682,-1.,-0.756562904646496));
#28204=CARTESIAN_POINT('Ctrl Pts',(-2.00028834739072,-1.,-0.757442676862341));
#28205=CARTESIAN_POINT('Ctrl Pts',(-1.9939983109871,-1.,-0.758281796766377));
#28206=CARTESIAN_POINT('Ctrl Pts',(-1.98771456680806,-1.,-0.759080037802242));
#28207=CARTESIAN_POINT('Ctrl Pts',(-1.98143741418156,-1.,-0.759837147452135));
#28208=CARTESIAN_POINT('Ctrl Pts',(-1.97516705321521,-1.,-0.760552825409855));
#28209=CARTESIAN_POINT('Ctrl Pts',(-1.96890351582545,-1.,-0.761226690483986));
#28210=CARTESIAN_POINT('Ctrl Pts',(-1.96264672744229,-1.,-0.761858300014575));
#28211=CARTESIAN_POINT('Ctrl Pts',(-1.95639665309893,-1.,-0.762447203806263));
#28212=CARTESIAN_POINT('Ctrl Pts',(-1.95015342590025,-1.,-0.762992990878774));
#28213=CARTESIAN_POINT('Ctrl Pts',(-1.94391746617626,-1.,-0.76349533353858));
#28214=CARTESIAN_POINT('Ctrl Pts',(-1.93768964875867,-1.,-0.763954049121393));
#28215=CARTESIAN_POINT('Ctrl Pts',(-1.93147105496367,-1.,-0.764369010673889));
#28216=CARTESIAN_POINT('Ctrl Pts',(-1.92526263537041,-1.,-0.764740025488189));
#28217=CARTESIAN_POINT('Ctrl Pts',(-1.91906491634197,-1.,-0.765066729667095));
#28218=CARTESIAN_POINT('Ctrl Pts',(-1.91287765805174,-1.,-0.765348465884739));
#28219=CARTESIAN_POINT('Ctrl Pts',(-1.90669961402362,-1.,-0.765584196937936));
#28220=CARTESIAN_POINT('Ctrl Pts',(-1.90052930393599,-1.,-0.765772772593395));
#28221=CARTESIAN_POINT('Ctrl Pts',(-1.89436577771389,-1.,-0.765913193856979));
#28222=CARTESIAN_POINT('Ctrl Pts',(-1.88820926433409,-1.,-0.76600483706209));
#28223=CARTESIAN_POINT('Ctrl Pts',(-1.88206215302561,-1.,-0.766047794851868));
#28224=CARTESIAN_POINT('Ctrl Pts',(-1.87592888967886,-1.,-0.766042837036759));
#28225=CARTESIAN_POINT('Ctrl Pts',(-1.86981398314345,-1.,-0.765990708546111));
#28226=CARTESIAN_POINT('Ctrl Pts',(-1.86372027063314,-1.,-0.765891519092557));
#28227=CARTESIAN_POINT('Ctrl Pts',(-1.85764741390391,-1.,-0.765744212909305));
#28228=CARTESIAN_POINT('Ctrl Pts',(-1.85158945130054,-1.,-0.765545710619023));
#28229=CARTESIAN_POINT('Ctrl Pts',(-1.8455369887591,-1.,-0.765291664861971));
#28230=CARTESIAN_POINT('Ctrl Pts',(-1.83948181064823,-1.,-0.764978057881687));
#28231=CARTESIAN_POINT('Ctrl Pts',(-1.8334207722714,-1.,-0.764602549687845));
#28232=CARTESIAN_POINT('Ctrl Pts',(-1.8273599120008,-1.,-0.764165902606055));
#28233=CARTESIAN_POINT('Ctrl Pts',(-1.82131873145297,-1.,-0.763673465462854));
#28234=CARTESIAN_POINT('Ctrl Pts',(-1.81532118405566,-1.,-0.763132003836783));
#28235=CARTESIAN_POINT('Ctrl Pts',(-1.80938551463989,-1.,-0.762546129464036));
#28236=CARTESIAN_POINT('Ctrl Pts',(-1.80351583877334,-1.,-0.761915336443515));
#28237=CARTESIAN_POINT('Ctrl Pts',(-1.79768986997735,-1.,-0.761229695230359));
#28238=CARTESIAN_POINT('Ctrl Pts',(-1.79185815610802,-1.,-0.760469555880425));
#28239=CARTESIAN_POINT('Ctrl Pts',(-1.78596964884526,-1.,-0.759614401109868));
#28240=CARTESIAN_POINT('Ctrl Pts',(-1.77999411220912,-1.,-0.75865062667738));
#28241=CARTESIAN_POINT('Ctrl Pts',(-1.77394167108342,-1.,-0.757578264077238));
#28242=CARTESIAN_POINT('Ctrl Pts',(-1.76789396003141,-1.,-0.756421896028403));
#28243=CARTESIAN_POINT('Ctrl Pts',(-1.7619781724032,-1.,-0.755220979975262));
#28244=CARTESIAN_POINT('Ctrl Pts',(-1.75631083600175,-1.,-0.75400925402848));
#28245=CARTESIAN_POINT('Ctrl Pts',(-1.75095139468809,-1.,-0.752797683531377));
#28246=CARTESIAN_POINT('Ctrl Pts',(-1.74585086852298,-1.,-0.751555614163629));
#28247=CARTESIAN_POINT('Ctrl Pts',(-1.74080458266705,-1.,-0.75019343597954));
#28248=CARTESIAN_POINT('Ctrl Pts',(-1.73550351679848,-1.,-0.748582462954854));
#28249=CARTESIAN_POINT('Ctrl Pts',(-1.72958533647399,-1.,-0.746574710096436));
#28250=CARTESIAN_POINT('Ctrl Pts',(-1.7226822991693,-1.,-0.744021445433764));
#28251=CARTESIAN_POINT('Ctrl Pts',(-1.71447789751927,-1.,-0.740795162032087));
#28252=CARTESIAN_POINT('Ctrl Pts',(-1.70473309006121,-1.,-0.736799665724771));
#28253=CARTESIAN_POINT('Ctrl Pts',(-1.69326921975743,-1.,-0.731963238697195));
#28254=CARTESIAN_POINT('Ctrl Pts',(-1.67996158455503,-1.,-0.726235967997433));
#28255=CARTESIAN_POINT('Ctrl Pts',(-1.6647288055568,-1.,-0.719585433804282));
#28256=CARTESIAN_POINT('Ctrl Pts',(-1.64752408832016,-1.,-0.711993139355394));
#28257=CARTESIAN_POINT('Ctrl Pts',(-1.63216541664676,-1.,-0.705159151988319));
#28258=CARTESIAN_POINT('Ctrl Pts',(-1.61974673472612,-1.,-0.699605146405088));
#28259=CARTESIAN_POINT('Ctrl Pts',(-1.61106790958151,-1.,-0.695712097881194));
#28260=CARTESIAN_POINT('Ctrl Pts',(-1.60662857109684,-1.,-0.693717979106306));
#28261=CARTESIAN_POINT('',(-1.5055822144029,-1.,-0.892032620296855));
#28262=CARTESIAN_POINT('Origin',(0.,-1.,0.));
#28263=CARTESIAN_POINT('',(-1.81978687191668,-1.,-1.23627494547115));
#28264=CARTESIAN_POINT('Ctrl Pts',(-1.5055822144029,-1.,-0.892032620296855));
#28265=CARTESIAN_POINT('Ctrl Pts',(-1.50980486806688,-1.,-0.894452006964543));
#28266=CARTESIAN_POINT('Ctrl Pts',(-1.51805569590094,-1.,-0.899185047483511));
#28267=CARTESIAN_POINT('Ctrl Pts',(-1.52984849887993,-1.,-0.905967409625651));
#28268=CARTESIAN_POINT('Ctrl Pts',(-1.54440491149498,-1.,-0.914375919026456));
#28269=CARTESIAN_POINT('Ctrl Pts',(-1.56065988578893,-1.,-0.923832188944341));
#28270=CARTESIAN_POINT('Ctrl Pts',(-1.57499388382243,-1.,-0.932246680108685));
#28271=CARTESIAN_POINT('Ctrl Pts',(-1.58744937487176,-1.,-0.939646377893399));
#28272=CARTESIAN_POINT('Ctrl Pts',(-1.59810042043673,-1.,-0.946078063315257));
#28273=CARTESIAN_POINT('Ctrl Pts',(-1.60706069896936,-1.,-0.951613284356035));
#28274=CARTESIAN_POINT('Ctrl Pts',(-1.61449324337085,-1.,-0.956354422920671));
#28275=CARTESIAN_POINT('Ctrl Pts',(-1.62061638140221,-1.,-0.960438326101729));
#28276=CARTESIAN_POINT('Ctrl Pts',(-1.62571930670187,-1.,-0.964046107040536));
#28277=CARTESIAN_POINT('Ctrl Pts',(-1.63013849959461,-1.,-0.967387853230345));
#28278=CARTESIAN_POINT('Ctrl Pts',(-1.63420665729798,-1.,-0.970669715997509));
#28279=CARTESIAN_POINT('Ctrl Pts',(-1.63820952658144,-1.,-0.974066058287418));
#28280=CARTESIAN_POINT('Ctrl Pts',(-1.64233990826687,-1.,-0.977689794119416));
#28281=CARTESIAN_POINT('Ctrl Pts',(-1.64665139190656,-1.,-0.981562530939489));
#28282=CARTESIAN_POINT('Ctrl Pts',(-1.65110016612638,-1.,-0.985642622920821));
#28283=CARTESIAN_POINT('Ctrl Pts',(-1.65559044289699,-1.,-0.989855627854165));
#28284=CARTESIAN_POINT('Ctrl Pts',(-1.66001553809947,-1.,-0.994121836661306));
#28285=CARTESIAN_POINT('Ctrl Pts',(-1.66430758030376,-1.,-0.998389654952758));
#28286=CARTESIAN_POINT('Ctrl Pts',(-1.66846059277303,-1.,-1.00265091003727));
#28287=CARTESIAN_POINT('Ctrl Pts',(-1.67250335383293,-1.,-1.00692206696414));
#28288=CARTESIAN_POINT('Ctrl Pts',(-1.67648246776464,-1.,-1.01123236493511));
#28289=CARTESIAN_POINT('Ctrl Pts',(-1.68044289894798,-1.,-1.01561026162773));
#28290=CARTESIAN_POINT('Ctrl Pts',(-1.68440578021706,-1.,-1.02006795074201));
#28291=CARTESIAN_POINT('Ctrl Pts',(-1.68836910178447,-1.,-1.02460180535255));
#28292=CARTESIAN_POINT('Ctrl Pts',(-1.69231840863458,-1.,-1.02919977579147));
#28293=CARTESIAN_POINT('Ctrl Pts',(-1.69623414782771,-1.,-1.03384646003588));
#28294=CARTESIAN_POINT('Ctrl Pts',(-1.70010052930962,-1.,-1.03852922490789));
#28295=CARTESIAN_POINT('Ctrl Pts',(-1.70391338707982,-1.,-1.04324363334554));
#28296=CARTESIAN_POINT('Ctrl Pts',(-1.70767646263649,-1.,-1.04799085404995));
#28297=CARTESIAN_POINT('Ctrl Pts',(-1.71139783543989,-1.,-1.05277517202855));
#28298=CARTESIAN_POINT('Ctrl Pts',(-1.7150865442702,-1.,-1.05760163192479));
#28299=CARTESIAN_POINT('Ctrl Pts',(-1.71874858456904,-1.,-1.06247324680647));
#28300=CARTESIAN_POINT('Ctrl Pts',(-1.72238500928453,-1.,-1.06738966975462));
#28301=CARTESIAN_POINT('Ctrl Pts',(-1.72599406198488,-1.,-1.07234866990252));
#28302=CARTESIAN_POINT('Ctrl Pts',(-1.72957248977424,-1.,-1.0773470373727));
#28303=CARTESIAN_POINT('Ctrl Pts',(-1.73311705663407,-1.,-1.08238162784749));
#28304=CARTESIAN_POINT('Ctrl Pts',(-1.73662628326091,-1.,-1.08745056285427));
#28305=CARTESIAN_POINT('Ctrl Pts',(-1.74010053962247,-1.,-1.09255329056493));
#28306=CARTESIAN_POINT('Ctrl Pts',(-1.74354119236208,-1.,-1.09768999241225));
#28307=CARTESIAN_POINT('Ctrl Pts',(-1.74695004214923,-1.,-1.10286118991143));
#28308=CARTESIAN_POINT('Ctrl Pts',(-1.7503286607592,-1.,-1.10806728183007));
#28309=CARTESIAN_POINT('Ctrl Pts',(-1.7536777209463,-1.,-1.11330807582551));
#28310=CARTESIAN_POINT('Ctrl Pts',(-1.75699720772105,-1.,-1.11858293216763));
#28311=CARTESIAN_POINT('Ctrl Pts',(-1.76028671825096,-1.,-1.12389096855086));
#28312=CARTESIAN_POINT('Ctrl Pts',(-1.7635457196617,-1.,-1.12923123555075));
#28313=CARTESIAN_POINT('Ctrl Pts',(-1.76677384551862,-1.,-1.1346029180462));
#28314=CARTESIAN_POINT('Ctrl Pts',(-1.76997111386769,-1.,-1.14000548336975));
#28315=CARTESIAN_POINT('Ctrl Pts',(-1.77313777896194,-1.,-1.1454385822692));
#28316=CARTESIAN_POINT('Ctrl Pts',(-1.7762742255701,-1.,-1.15090197841515));
#28317=CARTESIAN_POINT('Ctrl Pts',(-1.77938085564275,-1.,-1.15639547194698));
#28318=CARTESIAN_POINT('Ctrl Pts',(-1.78245795881009,-1.,-1.16191881298499));
#28319=CARTESIAN_POINT('Ctrl Pts',(-1.78550566040443,-1.,-1.16747166312303));
#28320=CARTESIAN_POINT('Ctrl Pts',(-1.78852398877616,-1.,-1.17305363177328));
#28321=CARTESIAN_POINT('Ctrl Pts',(-1.79151291552689,-1.,-1.17866429440809));
#28322=CARTESIAN_POINT('Ctrl Pts',(-1.79447240321515,-1.,-1.18430321697432));
#28323=CARTESIAN_POINT('Ctrl Pts',(-1.79740245923478,-1.,-1.18996997934445));
#28324=CARTESIAN_POINT('Ctrl Pts',(-1.80030314369879,-1.,-1.19566418930242));
#28325=CARTESIAN_POINT('Ctrl Pts',(-1.80317454838603,-1.,-1.20138548938974));
#28326=CARTESIAN_POINT('Ctrl Pts',(-1.80601678480707,-1.,-1.20713356605475));
#28327=CARTESIAN_POINT('Ctrl Pts',(-1.80882996917129,-1.,-1.21290815708314));
#28328=CARTESIAN_POINT('Ctrl Pts',(-1.81161420806656,-1.,-1.21870906103557));
#28329=CARTESIAN_POINT('Ctrl Pts',(-1.81436959210434,-1.,-1.2245361330495));
#28330=CARTESIAN_POINT('Ctrl Pts',(-1.8165508718364,-1.,-1.2292186489137));
#28331=CARTESIAN_POINT('Ctrl Pts',(-1.81817389921279,-1.,-1.2327422452705));
#28332=CARTESIAN_POINT('Ctrl Pts',(-1.81925017193666,-1.,-1.23509651170476));
#28333=CARTESIAN_POINT('Ctrl Pts',(-1.81978687191668,-1.,-1.23627494547115));
#28334=CARTESIAN_POINT('',(-1.73811241238545,-1.,-1.34869019493419));
#28335=CARTESIAN_POINT('',(-1.81978687191668,-1.,-1.23627494547115));
#28336=CARTESIAN_POINT('',(-1.31362392696032,-1.,-1.15624053661742));
#28337=CARTESIAN_POINT('Ctrl Pts',(-1.73811241238545,-1.,-1.34869019493419));
#28338=CARTESIAN_POINT('Ctrl Pts',(-1.73682580585691,-1.,-1.34854391898045));
#28339=CARTESIAN_POINT('Ctrl Pts',(-1.73425417885907,-1.,-1.34824783112887));
#28340=CARTESIAN_POINT('Ctrl Pts',(-1.7304014965394,-1.,-1.34779309152035));
#28341=CARTESIAN_POINT('Ctrl Pts',(-1.72527410680674,-1.,-1.34716554819527));
#28342=CARTESIAN_POINT('Ctrl Pts',(-1.7188807715049,-1.,-1.34634568653227));
#28343=CARTESIAN_POINT('Ctrl Pts',(-1.71250340686822,-1.,-1.34549029589416));
#28344=CARTESIAN_POINT('Ctrl Pts',(-1.70614212266738,-1.,-1.34459924533831));
#28345=CARTESIAN_POINT('Ctrl Pts',(-1.69979707754427,-1.,-1.34367237124483));
#28346=CARTESIAN_POINT('Ctrl Pts',(-1.6934684849687,-1.,-1.34270948206319));
#28347=CARTESIAN_POINT('Ctrl Pts',(-1.68715660868764,-1.,-1.341710374848));
#28348=CARTESIAN_POINT('Ctrl Pts',(-1.68086176030362,-1.,-1.34067485185203));
#28349=CARTESIAN_POINT('Ctrl Pts',(-1.67458429426086,-1.,-1.3396027347034));
#28350=CARTESIAN_POINT('Ctrl Pts',(-1.66832460783989,-1.,-1.33849388654388));
#28351=CARTESIAN_POINT('Ctrl Pts',(-1.66208312541983,-1.,-1.33734820885262));
#28352=CARTESIAN_POINT('Ctrl Pts',(-1.65586025952593,-1.,-1.33616559745172));
#28353=CARTESIAN_POINT('Ctrl Pts',(-1.6496563728683,-1.,-1.33494590467993));
#28354=CARTESIAN_POINT('Ctrl Pts',(-1.6434717485603,-1.,-1.33368890676572));
#28355=CARTESIAN_POINT('Ctrl Pts',(-1.63730653475089,-1.,-1.33239425103724));
#28356=CARTESIAN_POINT('Ctrl Pts',(-1.63116079730923,-1.,-1.33106149345645));
#28357=CARTESIAN_POINT('Ctrl Pts',(-1.62503464209797,-1.,-1.3296901950568));
#28358=CARTESIAN_POINT('Ctrl Pts',(-1.61892832270724,-1.,-1.32828000610449));
#28359=CARTESIAN_POINT('Ctrl Pts',(-1.6128423401575,-1.,-1.32683074483356));
#28360=CARTESIAN_POINT('Ctrl Pts',(-1.60677758290954,-1.,-1.32534250785782));
#28361=CARTESIAN_POINT('Ctrl Pts',(-1.60073511858687,-1.,-1.32381550858256));
#28362=CARTESIAN_POINT('Ctrl Pts',(-1.59471591079403,-1.,-1.32224985747682));
#28363=CARTESIAN_POINT('Ctrl Pts',(-1.58872057258245,-1.,-1.32064537110892));
#28364=CARTESIAN_POINT('Ctrl Pts',(-1.58274907898834,-1.,-1.31900135021432));
#28365=CARTESIAN_POINT('Ctrl Pts',(-1.5768005650559,-1.,-1.31731642317187));
#28366=CARTESIAN_POINT('Ctrl Pts',(-1.57087397835723,-1.,-1.31558903860016));
#28367=CARTESIAN_POINT('Ctrl Pts',(-1.56496872402353,-1.,-1.31381795281002));
#28368=CARTESIAN_POINT('Ctrl Pts',(-1.55908521254821,-1.,-1.31200264341696));
#28369=CARTESIAN_POINT('Ctrl Pts',(-1.55322568759481,-1.,-1.31014393684222));
#28370=CARTESIAN_POINT('Ctrl Pts',(-1.54739413957185,-1.,-1.30824393907473));
#28371=CARTESIAN_POINT('Ctrl Pts',(-1.54159462645432,-1.,-1.30630475189556));
#28372=CARTESIAN_POINT('Ctrl Pts',(-1.53582981268977,-1.,-1.30432735639489));
#28373=CARTESIAN_POINT('Ctrl Pts',(-1.53009970283891,-1.,-1.30231064395568));
#28374=CARTESIAN_POINT('Ctrl Pts',(-1.52439957861062,-1.,-1.30024984366328));
#28375=CARTESIAN_POINT('Ctrl Pts',(-1.51872184912724,-1.,-1.29813791800747));
#28376=CARTESIAN_POINT('Ctrl Pts',(-1.51305994241402,-1.,-1.29596850710509));
#28377=CARTESIAN_POINT('Ctrl Pts',(-1.50741159078365,-1.,-1.29373841372842));
#28378=CARTESIAN_POINT('Ctrl Pts',(-1.50178230149776,-1.,-1.29145022885181));
#28379=CARTESIAN_POINT('Ctrl Pts',(-1.49618896881754,-1.,-1.28911506584254));
#28380=CARTESIAN_POINT('Ctrl Pts',(-1.4906522831278,-1.,-1.2867467611644));
#28381=CARTESIAN_POINT('Ctrl Pts',(-1.4851881711891,-1.,-1.28435533880201));
#28382=CARTESIAN_POINT('Ctrl Pts',(-1.47980070347095,-1.,-1.28194158939517));
#28383=CARTESIAN_POINT('Ctrl Pts',(-1.4744717526707,-1.,-1.2794891824849));
#28384=CARTESIAN_POINT('Ctrl Pts',(-1.46916035917133,-1.,-1.27696414831089));
#28385=CARTESIAN_POINT('Ctrl Pts',(-1.46382431332476,-1.,-1.27433119897822));
#28386=CARTESIAN_POINT('Ctrl Pts',(-1.45843906294697,-1.,-1.27156805265289));
#28387=CARTESIAN_POINT('Ctrl Pts',(-1.45301422764247,-1.,-1.2686778680489));
#28388=CARTESIAN_POINT('Ctrl Pts',(-1.44761985001662,-1.,-1.26570925118868));
#28389=CARTESIAN_POINT('Ctrl Pts',(-1.44236470511303,-1.,-1.26273903323859));
#28390=CARTESIAN_POINT('Ctrl Pts',(-1.43734919180848,-1.,-1.25983531012005));
#28391=CARTESIAN_POINT('Ctrl Pts',(-1.43262645609691,-1.,-1.25702687965755));
#28392=CARTESIAN_POINT('Ctrl Pts',(-1.42815938799387,-1.,-1.25426945222639));
#28393=CARTESIAN_POINT('Ctrl Pts',(-1.42378102115575,-1.,-1.2514145557001));
#28394=CARTESIAN_POINT('Ctrl Pts',(-1.41923722596025,-1.,-1.24824430986571));
#28395=CARTESIAN_POINT('Ctrl Pts',(-1.41422913175179,-1.,-1.24450600513056));
#28396=CARTESIAN_POINT('Ctrl Pts',(-1.40845295531283,-1.,-1.23994455029534));
#28397=CARTESIAN_POINT('Ctrl Pts',(-1.40164708206106,-1.,-1.23434087290423));
#28398=CARTESIAN_POINT('Ctrl Pts',(-1.39361389568796,-1.,-1.22752961899387));
#28399=CARTESIAN_POINT('Ctrl Pts',(-1.38420564527715,-1.,-1.21938737280852));
#28400=CARTESIAN_POINT('Ctrl Pts',(-1.37331915607905,-1.,-1.20982812925645));
#28401=CARTESIAN_POINT('Ctrl Pts',(-1.36088705043885,-1.,-1.1987959077932));
#28402=CARTESIAN_POINT('Ctrl Pts',(-1.34687054001093,-1.,-1.18625865667441));
#28403=CARTESIAN_POINT('Ctrl Pts',(-1.33437539347008,-1.,-1.17501305789857));
#28404=CARTESIAN_POINT('Ctrl Pts',(-1.32428080721772,-1.,-1.16589330093588));
#28405=CARTESIAN_POINT('Ctrl Pts',(-1.31722977216397,-1.,-1.15950888730809));
#28406=CARTESIAN_POINT('Ctrl Pts',(-1.31362392696032,-1.,-1.15624053661742));
#28407=CARTESIAN_POINT('',(-1.15624053661742,-1.,-1.31362392696033));
#28408=CARTESIAN_POINT('Origin',(0.,-1.,0.));
#28409=CARTESIAN_POINT('',(-1.34869019493419,-1.,-1.73811241238545));
#28410=CARTESIAN_POINT('Ctrl Pts',(-1.15624053661742,-1.,-1.31362392696033));
#28411=CARTESIAN_POINT('Ctrl Pts',(-1.15950888730433,-1.,-1.3172297721596));
#28412=CARTESIAN_POINT('Ctrl Pts',(-1.16589330092532,-1.,-1.32428080720544));
#28413=CARTESIAN_POINT('Ctrl Pts',(-1.17501305787994,-1.,-1.33437539344842));
#28414=CARTESIAN_POINT('Ctrl Pts',(-1.18625865664915,-1.,-1.34687053998157));
#28415=CARTESIAN_POINT('Ctrl Pts',(-1.1987959077656,-1.,-1.36088705040677));
#28416=CARTESIAN_POINT('Ctrl Pts',(-1.20982812923113,-1.,-1.37331915604962));
#28417=CARTESIAN_POINT('Ctrl Pts',(-1.21938737278853,-1.,-1.38420564525391));
#28418=CARTESIAN_POINT('Ctrl Pts',(-1.22752961898063,-1.,-1.39361389567257));
#28419=CARTESIAN_POINT('Ctrl Pts',(-1.23434087289768,-1.,-1.40164708205345));
#28420=CARTESIAN_POINT('Ctrl Pts',(-1.23994455029421,-1.,-1.40845295531151));
#28421=CARTESIAN_POINT('Ctrl Pts',(-1.24450600513278,-1.,-1.41422913175437));
#28422=CARTESIAN_POINT('Ctrl Pts',(-1.24824430986911,-1.,-1.41923722596421));
#28423=CARTESIAN_POINT('Ctrl Pts',(-1.25141455570299,-1.,-1.42378102115911));
#28424=CARTESIAN_POINT('Ctrl Pts',(-1.25426945222783,-1.,-1.42815938799555));
#28425=CARTESIAN_POINT('Ctrl Pts',(-1.25702687965744,-1.,-1.43262645609679));
#28426=CARTESIAN_POINT('Ctrl Pts',(-1.25983531011894,-1.,-1.43734919180719));
#28427=CARTESIAN_POINT('Ctrl Pts',(-1.26273903323723,-1.,-1.44236470511145));
#28428=CARTESIAN_POINT('Ctrl Pts',(-1.26570925118767,-1.,-1.44761985001544));
#28429=CARTESIAN_POINT('Ctrl Pts',(-1.26867786804854,-1.,-1.45301422764205));
#28430=CARTESIAN_POINT('Ctrl Pts',(-1.27156805265312,-1.,-1.45843906294725));
#28431=CARTESIAN_POINT('Ctrl Pts',(-1.27433119897877,-1.,-1.4638243133254));
#28432=CARTESIAN_POINT('Ctrl Pts',(-1.27696414831144,-1.,-1.46916035917197));
#28433=CARTESIAN_POINT('Ctrl Pts',(-1.27948918248524,-1.,-1.4744717526711));
#28434=CARTESIAN_POINT('Ctrl Pts',(-1.28194158939522,-1.,-1.47980070347102));
#28435=CARTESIAN_POINT('Ctrl Pts',(-1.28435533880184,-1.,-1.48518817118891));
#28436=CARTESIAN_POINT('Ctrl Pts',(-1.28674676116415,-1.,-1.4906522831275));
#28437=CARTESIAN_POINT('Ctrl Pts',(-1.28911506584232,-1.,-1.49618896881729));
#28438=CARTESIAN_POINT('Ctrl Pts',(-1.29145022885171,-1.,-1.50178230149764));
#28439=CARTESIAN_POINT('Ctrl Pts',(-1.29373841372843,-1.,-1.50741159078367));
#28440=CARTESIAN_POINT('Ctrl Pts',(-1.29596850710518,-1.,-1.51305994241412));
#28441=CARTESIAN_POINT('Ctrl Pts',(-1.29813791800757,-1.,-1.51872184912735));
#28442=CARTESIAN_POINT('Ctrl Pts',(-1.30024984366334,-1.,-1.5243995786107));
#28443=CARTESIAN_POINT('Ctrl Pts',(-1.3023106439557,-1.,-1.53009970283893));
#28444=CARTESIAN_POINT('Ctrl Pts',(-1.30432735639487,-1.,-1.53582981268976));
#28445=CARTESIAN_POINT('Ctrl Pts',(-1.30630475189553,-1.,-1.54159462645428));
#28446=CARTESIAN_POINT('Ctrl Pts',(-1.30824393907471,-1.,-1.54739413957183));
#28447=CARTESIAN_POINT('Ctrl Pts',(-1.31014393684221,-1.,-1.55322568759481));
#28448=CARTESIAN_POINT('Ctrl Pts',(-1.31200264341696,-1.,-1.55908521254822));
#28449=CARTESIAN_POINT('Ctrl Pts',(-1.31381795281002,-1.,-1.56496872402352));
#28450=CARTESIAN_POINT('Ctrl Pts',(-1.31558903860015,-1.,-1.57087397835721));
#28451=CARTESIAN_POINT('Ctrl Pts',(-1.31731642317183,-1.,-1.57680056505585));
#28452=CARTESIAN_POINT('Ctrl Pts',(-1.31900135021428,-1.,-1.58274907898829));
#28453=CARTESIAN_POINT('Ctrl Pts',(-1.32064537110891,-1.,-1.58872057258244));
#28454=CARTESIAN_POINT('Ctrl Pts',(-1.32224985747686,-1.,-1.59471591079408));
#28455=CARTESIAN_POINT('Ctrl Pts',(-1.32381550858266,-1.,-1.600735118587));
#28456=CARTESIAN_POINT('Ctrl Pts',(-1.32534250785794,-1.,-1.6067775829097));
#28457=CARTESIAN_POINT('Ctrl Pts',(-1.32683074483365,-1.,-1.61284234015762));
#28458=CARTESIAN_POINT('Ctrl Pts',(-1.32828000610448,-1.,-1.61892832270723));
#28459=CARTESIAN_POINT('Ctrl Pts',(-1.32969019505665,-1.,-1.62503464209777));
#28460=CARTESIAN_POINT('Ctrl Pts',(-1.33106149345618,-1.,-1.63116079730887));
#28461=CARTESIAN_POINT('Ctrl Pts',(-1.33239425103694,-1.,-1.6373065347505));
#28462=CARTESIAN_POINT('Ctrl Pts',(-1.33368890676554,-1.,-1.64347174856007));
#28463=CARTESIAN_POINT('Ctrl Pts',(-1.33494590468003,-1.,-1.64965637286843));
#28464=CARTESIAN_POINT('Ctrl Pts',(-1.33616559745217,-1.,-1.65586025952651));
#28465=CARTESIAN_POINT('Ctrl Pts',(-1.33734820885331,-1.,-1.66208312542073));
#28466=CARTESIAN_POINT('Ctrl Pts',(-1.33849388654458,-1.,-1.66832460784078));
#28467=CARTESIAN_POINT('Ctrl Pts',(-1.33960273470372,-1.,-1.67458429426126));
#28468=CARTESIAN_POINT('Ctrl Pts',(-1.3406748518516,-1.,-1.68086176030308));
#28469=CARTESIAN_POINT('Ctrl Pts',(-1.34171037484673,-1.,-1.68715660868602));
#28470=CARTESIAN_POINT('Ctrl Pts',(-1.34270948206139,-1.,-1.6934684849664));
#28471=CARTESIAN_POINT('Ctrl Pts',(-1.34367237124322,-1.,-1.69979707754221));
#28472=CARTESIAN_POINT('Ctrl Pts',(-1.34459924533783,-1.,-1.70614212266676));
#28473=CARTESIAN_POINT('Ctrl Pts',(-1.34549029589563,-1.,-1.71250340687011));
#28474=CARTESIAN_POINT('Ctrl Pts',(-1.34634568653586,-1.,-1.7188807715095));
#28475=CARTESIAN_POINT('Ctrl Pts',(-1.34716554820013,-1.,-1.72527410681298));
#28476=CARTESIAN_POINT('Ctrl Pts',(-1.3477930915247,-1.,-1.73040149654497));
#28477=CARTESIAN_POINT('Ctrl Pts',(-1.34824783113158,-1.,-1.73425417886255));
#28478=CARTESIAN_POINT('Ctrl Pts',(-1.34854391898145,-1.,-1.73682580585819));
#28479=CARTESIAN_POINT('Ctrl Pts',(-1.34869019493419,-1.,-1.73811241238545));
#28480=CARTESIAN_POINT('',(-1.23627494547115,-1.,-1.81978687191668));
#28481=CARTESIAN_POINT('',(-1.34869019493419,-1.,-1.73811241238545));
#28482=CARTESIAN_POINT('',(-0.892032620296855,-1.,-1.5055822144029));
#28483=CARTESIAN_POINT('Ctrl Pts',(-1.23627494547115,-1.,-1.81978687191668));
#28484=CARTESIAN_POINT('Ctrl Pts',(-1.23509651170384,-1.,-1.81925017193531));
#28485=CARTESIAN_POINT('Ctrl Pts',(-1.23274224526804,-1.,-1.81817389920914));
#28486=CARTESIAN_POINT('Ctrl Pts',(-1.22921864890975,-1.,-1.81655087183054));
#28487=CARTESIAN_POINT('Ctrl Pts',(-1.22453613304507,-1.,-1.81436959209778));
#28488=CARTESIAN_POINT('Ctrl Pts',(-1.2187090610323,-1.,-1.81161420806172));
#28489=CARTESIAN_POINT('Ctrl Pts',(-1.2129081570818,-1.,-1.80882996916931));
#28490=CARTESIAN_POINT('Ctrl Pts',(-1.20713356605519,-1.,-1.80601678480772));
#28491=CARTESIAN_POINT('Ctrl Pts',(-1.2013854893912,-1.,-1.8031745483882));
#28492=CARTESIAN_POINT('Ctrl Pts',(-1.19566418930405,-1.,-1.80030314370121));
#28493=CARTESIAN_POINT('Ctrl Pts',(-1.1899699793456,-1.,-1.79740245923649));
#28494=CARTESIAN_POINT('Ctrl Pts',(-1.18430321697471,-1.,-1.79447240321572));
#28495=CARTESIAN_POINT('Ctrl Pts',(-1.17866429440781,-1.,-1.79151291552646));
#28496=CARTESIAN_POINT('Ctrl Pts',(-1.17305363177265,-1.,-1.78852398877523));
#28497=CARTESIAN_POINT('Ctrl Pts',(-1.16747166312239,-1.,-1.78550566040349));
#28498=CARTESIAN_POINT('Ctrl Pts',(-1.16191881298458,-1.,-1.78245795880949));
#28499=CARTESIAN_POINT('Ctrl Pts',(-1.15639547194689,-1.,-1.77938085564261));
#28500=CARTESIAN_POINT('Ctrl Pts',(-1.15090197841531,-1.,-1.77627422557034));
#28501=CARTESIAN_POINT('Ctrl Pts',(-1.14543858226948,-1.,-1.77313777896234));
#28502=CARTESIAN_POINT('Ctrl Pts',(-1.14000548337,-1.,-1.76997111386806));
#28503=CARTESIAN_POINT('Ctrl Pts',(-1.13460291804635,-1.,-1.76677384551883));
#28504=CARTESIAN_POINT('Ctrl Pts',(-1.12923123555076,-1.,-1.76354571966171));
#28505=CARTESIAN_POINT('Ctrl Pts',(-1.12389096855078,-1.,-1.76028671825084));
#28506=CARTESIAN_POINT('Ctrl Pts',(-1.11858293216752,-1.,-1.75699720772089));
#28507=CARTESIAN_POINT('Ctrl Pts',(-1.11330807582542,-1.,-1.75367772094617));
#28508=CARTESIAN_POINT('Ctrl Pts',(-1.10806728183003,-1.,-1.75032866075914));
#28509=CARTESIAN_POINT('Ctrl Pts',(-1.10286118991144,-1.,-1.74695004214924));
#28510=CARTESIAN_POINT('Ctrl Pts',(-1.09768999241229,-1.,-1.74354119236212));
#28511=CARTESIAN_POINT('Ctrl Pts',(-1.09255329056496,-1.,-1.74010053962252));
#28512=CARTESIAN_POINT('Ctrl Pts',(-1.08745056285429,-1.,-1.73662628326093));
#28513=CARTESIAN_POINT('Ctrl Pts',(-1.08238162784749,-1.,-1.73311705663407));
#28514=CARTESIAN_POINT('Ctrl Pts',(-1.0773470373727,-1.,-1.72957248977424));
#28515=CARTESIAN_POINT('Ctrl Pts',(-1.07234866990252,-1.,-1.72599406198489));
#28516=CARTESIAN_POINT('Ctrl Pts',(-1.06738966975463,-1.,-1.72238500928456));
#28517=CARTESIAN_POINT('Ctrl Pts',(-1.0624732468065,-1.,-1.71874858456908));
#28518=CARTESIAN_POINT('Ctrl Pts',(-1.05760163192481,-1.,-1.71508654427022));
#28519=CARTESIAN_POINT('Ctrl Pts',(-1.05277517202854,-1.,-1.71139783543986));
#28520=CARTESIAN_POINT('Ctrl Pts',(-1.0479908540499,-1.,-1.70767646263641));
#28521=CARTESIAN_POINT('Ctrl Pts',(-1.04324363334546,-1.,-1.70391338707969));
#28522=CARTESIAN_POINT('Ctrl Pts',(-1.03852922490782,-1.,-1.70010052930951));
#28523=CARTESIAN_POINT('Ctrl Pts',(-1.03384646003587,-1.,-1.69623414782769));
#28524=CARTESIAN_POINT('Ctrl Pts',(-1.02919977579155,-1.,-1.69231840863471));
#28525=CARTESIAN_POINT('Ctrl Pts',(-1.02460180535272,-1.,-1.68836910178475));
#28526=CARTESIAN_POINT('Ctrl Pts',(-1.02006795074222,-1.,-1.68440578021739));
#28527=CARTESIAN_POINT('Ctrl Pts',(-1.01561026162787,-1.,-1.6804428989482));
#28528=CARTESIAN_POINT('Ctrl Pts',(-1.01123236493507,-1.,-1.67648246776457));
#28529=CARTESIAN_POINT('Ctrl Pts',(-1.00692206696387,-1.,-1.67250335383248));
#28530=CARTESIAN_POINT('Ctrl Pts',(-1.00265091003682,-1.,-1.66846059277231));
#28531=CARTESIAN_POINT('Ctrl Pts',(-0.998389654952317,-1.,-1.66430758030304));
#28532=CARTESIAN_POINT('Ctrl Pts',(-0.994121836661116,-1.,-1.66001553809916));
#28533=CARTESIAN_POINT('Ctrl Pts',(-0.98985562785445,-1.,-1.65559044289746));
#28534=CARTESIAN_POINT('Ctrl Pts',(-0.985642622921626,-1.,-1.6511001661277));
#28535=CARTESIAN_POINT('Ctrl Pts',(-0.981562530940574,-1.,-1.64665139190834));
#28536=CARTESIAN_POINT('Ctrl Pts',(-0.977689794120297,-1.,-1.64233990826831));
#28537=CARTESIAN_POINT('Ctrl Pts',(-0.974066058287501,-1.,-1.63820952658157));
#28538=CARTESIAN_POINT('Ctrl Pts',(-0.970669715996356,-1.,-1.63420665729609));
#28539=CARTESIAN_POINT('Ctrl Pts',(-0.967387853228041,-1.,-1.63013849959083));
#28540=CARTESIAN_POINT('Ctrl Pts',(-0.964046107037821,-1.,-1.6257193066974));
#28541=CARTESIAN_POINT('Ctrl Pts',(-0.960438326099958,-1.,-1.62061638139929));
#28542=CARTESIAN_POINT('Ctrl Pts',(-0.956354422921573,-1.,-1.61449324337233));
#28543=CARTESIAN_POINT('Ctrl Pts',(-0.951613284361248,-1.,-1.60706069897794));
#28544=CARTESIAN_POINT('Ctrl Pts',(-0.946078063325796,-1.,-1.59810042045408));
#28545=CARTESIAN_POINT('Ctrl Pts',(-0.939646377909319,-1.,-1.58744937489796));
#28546=CARTESIAN_POINT('Ctrl Pts',(-0.932246680128849,-1.,-1.57499388385561));
#28547=CARTESIAN_POINT('Ctrl Pts',(-0.923832188966322,-1.,-1.56065988582509));
#28548=CARTESIAN_POINT('Ctrl Pts',(-0.91437591904658,-1.,-1.54440491152808));
#28549=CARTESIAN_POINT('Ctrl Pts',(-0.905967409640499,-1.,-1.52984849890434));
#28550=CARTESIAN_POINT('Ctrl Pts',(-0.89918504749193,-1.,-1.51805569591479));
#28551=CARTESIAN_POINT('Ctrl Pts',(-0.894452006967538,-1.,-1.50980486807181));
#28552=CARTESIAN_POINT('Ctrl Pts',(-0.892032620296855,-1.,-1.5055822144029));
#28553=CARTESIAN_POINT('',(-0.693717979106305,-1.,-1.60662857109684));
#28554=CARTESIAN_POINT('Origin',(0.,-1.,0.));
#28555=CARTESIAN_POINT('',(-0.745574324794401,-1.,-2.0698113262342));
#28556=CARTESIAN_POINT('Ctrl Pts',(-0.693717979106305,-1.,-1.60662857109684));
#28557=CARTESIAN_POINT('Ctrl Pts',(-0.69571209787897,-1.,-1.61106790957619));
#28558=CARTESIAN_POINT('Ctrl Pts',(-0.699605146398837,-1.,-1.61974673471117));
#28559=CARTESIAN_POINT('Ctrl Pts',(-0.705159151977294,-1.,-1.6321654166204));
#28560=CARTESIAN_POINT('Ctrl Pts',(-0.711993139340447,-1.,-1.64752408828442));
#28561=CARTESIAN_POINT('Ctrl Pts',(-0.71958543378795,-1.,-1.66472880551777));
#28562=CARTESIAN_POINT('Ctrl Pts',(-0.726235967982445,-1.,-1.67996158451922));
#28563=CARTESIAN_POINT('Ctrl Pts',(-0.731963238685357,-1.,-1.69326921972915));
#28564=CARTESIAN_POINT('Ctrl Pts',(-0.736799665716932,-1.,-1.70473309004249));
#28565=CARTESIAN_POINT('Ctrl Pts',(-0.74079516202821,-1.,-1.71447789751001));
#28566=CARTESIAN_POINT('Ctrl Pts',(-0.744021445433093,-1.,-1.72268229916769));
#28567=CARTESIAN_POINT('Ctrl Pts',(-0.746574710097752,-1.,-1.72958533647714));
#28568=CARTESIAN_POINT('Ctrl Pts',(-0.74858246295687,-1.,-1.7355035168033));
#28569=CARTESIAN_POINT('Ctrl Pts',(-0.750193435981249,-1.,-1.74080458267114));
#28570=CARTESIAN_POINT('Ctrl Pts',(-0.751555614164482,-1.,-1.74585086852502));
#28571=CARTESIAN_POINT('Ctrl Pts',(-0.752797683531314,-1.,-1.75095139468794));
#28572=CARTESIAN_POINT('Ctrl Pts',(-0.754009254027829,-1.,-1.75631083600019));
#28573=CARTESIAN_POINT('Ctrl Pts',(-0.755220979974461,-1.,-1.76197817240128));
#28574=CARTESIAN_POINT('Ctrl Pts',(-0.75642189602781,-1.,-1.76789396002998));
#28575=CARTESIAN_POINT('Ctrl Pts',(-0.757578264077029,-1.,-1.77394167108292));
#28576=CARTESIAN_POINT('Ctrl Pts',(-0.758650626677518,-1.,-1.77999411220945));
#28577=CARTESIAN_POINT('Ctrl Pts',(-0.759614401110189,-1.,-1.78596964884604));
#28578=CARTESIAN_POINT('Ctrl Pts',(-0.760469555880749,-1.,-1.7918581561088));
#28579=CARTESIAN_POINT('Ctrl Pts',(-0.761229695230558,-1.,-1.79768986997783));
#28580=CARTESIAN_POINT('Ctrl Pts',(-0.761915336443547,-1.,-1.80351583877342));
#28581=CARTESIAN_POINT('Ctrl Pts',(-0.762546129463938,-1.,-1.80938551463965));
#28582=CARTESIAN_POINT('Ctrl Pts',(-0.763132003836634,-1.,-1.8153211840553));
#28583=CARTESIAN_POINT('Ctrl Pts',(-0.763673465462726,-1.,-1.82131873145266));
#28584=CARTESIAN_POINT('Ctrl Pts',(-0.764165902605995,-1.,-1.82735991200065));
#28585=CARTESIAN_POINT('Ctrl Pts',(-0.764602549687853,-1.,-1.83342077227142));
#28586=CARTESIAN_POINT('Ctrl Pts',(-0.764978057881737,-1.,-1.83948181064835));
#28587=CARTESIAN_POINT('Ctrl Pts',(-0.765291664862029,-1.,-1.84553698875924));
#28588=CARTESIAN_POINT('Ctrl Pts',(-0.765545710619062,-1.,-1.85158945130063));
#28589=CARTESIAN_POINT('Ctrl Pts',(-0.765744212909318,-1.,-1.85764741390394));
#28590=CARTESIAN_POINT('Ctrl Pts',(-0.765891519092547,-1.,-1.86372027063312));
#28591=CARTESIAN_POINT('Ctrl Pts',(-0.765990708546091,-1.,-1.86981398314341));
#28592=CARTESIAN_POINT('Ctrl Pts',(-0.766042837036744,-1.,-1.87592888967883));
#28593=CARTESIAN_POINT('Ctrl Pts',(-0.766047794851865,-1.,-1.88206215302561));
#28594=CARTESIAN_POINT('Ctrl Pts',(-0.766004837062091,-1.,-1.88820926433409));
#28595=CARTESIAN_POINT('Ctrl Pts',(-0.765913193856978,-1.,-1.89436577771388));
#28596=CARTESIAN_POINT('Ctrl Pts',(-0.765772772593386,-1.,-1.90052930393596));
#28597=CARTESIAN_POINT('Ctrl Pts',(-0.765584196937919,-1.,-1.90669961402356));
#28598=CARTESIAN_POINT('Ctrl Pts',(-0.765348465884722,-1.,-1.91287765805169));
#28599=CARTESIAN_POINT('Ctrl Pts',(-0.765066729667088,-1.,-1.91906491634196));
#28600=CARTESIAN_POINT('Ctrl Pts',(-0.764740025488211,-1.,-1.92526263537048));
#28601=CARTESIAN_POINT('Ctrl Pts',(-0.764369010673941,-1.,-1.93147105496382));
#28602=CARTESIAN_POINT('Ctrl Pts',(-0.763954049121458,-1.,-1.93768964875886));
#28603=CARTESIAN_POINT('Ctrl Pts',(-0.763495333538629,-1.,-1.9439174661764));
#28604=CARTESIAN_POINT('Ctrl Pts',(-0.762992990878769,-1.,-1.95015342590024));
#28605=CARTESIAN_POINT('Ctrl Pts',(-0.762447203806179,-1.,-1.95639665309869));
#28606=CARTESIAN_POINT('Ctrl Pts',(-0.761858300014423,-1.,-1.96264672744186));
#28607=CARTESIAN_POINT('Ctrl Pts',(-0.76122669048382,-1.,-1.96890351582499));
#28608=CARTESIAN_POINT('Ctrl Pts',(-0.760552825409757,-1.,-1.97516705321494));
#28609=CARTESIAN_POINT('Ctrl Pts',(-0.75983714745219,-1.,-1.98143741418172));
#28610=CARTESIAN_POINT('Ctrl Pts',(-0.759080037802488,-1.,-1.98771456680874));
#28611=CARTESIAN_POINT('Ctrl Pts',(-0.758281796766761,-1.,-1.99399831098817));
#28612=CARTESIAN_POINT('Ctrl Pts',(-0.757442676862724,-1.,-2.00028834739178));
#28613=CARTESIAN_POINT('Ctrl Pts',(-0.75656290464667,-1.,-2.0065843158773));
#28614=CARTESIAN_POINT('Ctrl Pts',(-0.755642704957865,-1.,-2.01288584328084));
#28615=CARTESIAN_POINT('Ctrl Pts',(-0.754682330722816,-1.,-2.01919259405809));
#28616=CARTESIAN_POINT('Ctrl Pts',(-0.753682061112768,-1.,-2.02550428623313));
#28617=CARTESIAN_POINT('Ctrl Pts',(-0.752642180487211,-1.,-2.03182068456221));
#28618=CARTESIAN_POINT('Ctrl Pts',(-0.751562963361115,-1.,-2.03814160092099));
#28619=CARTESIAN_POINT('Ctrl Pts',(-0.750444657875576,-1.,-2.04446689147979));
#28620=CARTESIAN_POINT('Ctrl Pts',(-0.749287468665046,-1.,-2.05079645592154));
#28621=CARTESIAN_POINT('Ctrl Pts',(-0.748091554183802,-1.,-2.05713023031006));
#28622=CARTESIAN_POINT('Ctrl Pts',(-0.747103932787919,-1.,-2.06220058927826));
#28623=CARTESIAN_POINT('Ctrl Pts',(-0.7463458715442,-1.,-2.06600523016815));
#28624=CARTESIAN_POINT('Ctrl Pts',(-0.745832791378367,-1.,-2.06854248895728));
#28625=CARTESIAN_POINT('Ctrl Pts',(-0.745574324794401,-1.,-2.0698113262342));
#28626=CARTESIAN_POINT('',(-0.61342227326009,-1.,-2.11275013067528));
#28627=CARTESIAN_POINT('',(-0.745574324794401,-1.,-2.0698113262342));
#28628=CARTESIAN_POINT('',(-0.383122945602004,-1.,-1.7075470150345));
#28629=CARTESIAN_POINT('Ctrl Pts',(-0.61342227326009,-1.,-2.11275013067528));
#28630=CARTESIAN_POINT('Ctrl Pts',(-0.6124673655618,-1.,-2.11187554259986));
#28631=CARTESIAN_POINT('Ctrl Pts',(-0.610560911689899,-1.,-2.11012443807238));
#28632=CARTESIAN_POINT('Ctrl Pts',(-0.607711315454876,-1.,-2.1074919961518));
#28633=CARTESIAN_POINT('Ctrl Pts',(-0.60393203073603,-1.,-2.10397049886949));
#28634=CARTESIAN_POINT('Ctrl Pts',(-0.599241616420533,-1.,-2.0995493086477));
#28635=CARTESIAN_POINT('Ctrl Pts',(-0.594585006052162,-1.,-2.0951087622027));
#28636=CARTESIAN_POINT('Ctrl Pts',(-0.589962365403406,-1.,-2.09064881812129));
#28637=CARTESIAN_POINT('Ctrl Pts',(-0.585373918991617,-1.,-2.08616943727951));
#28638=CARTESIAN_POINT('Ctrl Pts',(-0.580819952108063,-1.,-2.08167059018418));
#28639=CARTESIAN_POINT('Ctrl Pts',(-0.576300797416844,-1.,-2.07715226767559));
#28640=CARTESIAN_POINT('Ctrl Pts',(-0.571816823242603,-1.,-2.07261449292824));
#28641=CARTESIAN_POINT('Ctrl Pts',(-0.567368421181087,-1.,-2.06805732997334));
#28642=CARTESIAN_POINT('Ctrl Pts',(-0.562955993082261,-1.,-2.06348090160589));
#28643=CARTESIAN_POINT('Ctrl Pts',(-0.558579940185151,-1.,-2.05888537756462));
#28644=CARTESIAN_POINT('Ctrl Pts',(-0.554240657463906,-1.,-2.05427091604413));
#28645=CARTESIAN_POINT('Ctrl Pts',(-0.549938525150295,-1.,-2.04963761077958));
#28646=CARTESIAN_POINT('Ctrl Pts',(-0.54567390381743,-1.,-2.04498544714588));
#28647=CARTESIAN_POINT('Ctrl Pts',(-0.541447120615659,-1.,-2.04031422690527));
#28648=CARTESIAN_POINT('Ctrl Pts',(-0.537258489833262,-1.,-2.03562362954037));
#28649=CARTESIAN_POINT('Ctrl Pts',(-0.533108355132977,-1.,-2.03091336214426));
#28650=CARTESIAN_POINT('Ctrl Pts',(-0.528997127241914,-1.,-2.0261832908329));
#28651=CARTESIAN_POINT('Ctrl Pts',(-0.524925318333476,-1.,-2.02143356304698));
#28652=CARTESIAN_POINT('Ctrl Pts',(-0.52089359039937,-1.,-2.01666477917286));
#28653=CARTESIAN_POINT('Ctrl Pts',(-0.516902681728687,-1.,-2.01187773939242));
#28654=CARTESIAN_POINT('Ctrl Pts',(-0.512953306961792,-1.,-2.00707309946949));
#28655=CARTESIAN_POINT('Ctrl Pts',(-0.509046069886157,-1.,-2.00225107134734));
#28656=CARTESIAN_POINT('Ctrl Pts',(-0.505181361323026,-1.,-1.99741107463572));
#28657=CARTESIAN_POINT('Ctrl Pts',(-0.501359287727146,-1.,-1.99255149126155));
#28658=CARTESIAN_POINT('Ctrl Pts',(-0.497579909545574,-1.,-1.98767044752932));
#28659=CARTESIAN_POINT('Ctrl Pts',(-0.493843476541495,-1.,-1.98276658761821));
#28660=CARTESIAN_POINT('Ctrl Pts',(-0.490150627860952,-1.,-1.97783973019229));
#28661=CARTESIAN_POINT('Ctrl Pts',(-0.486502692907659,-1.,-1.97289186263272));
#28662=CARTESIAN_POINT('Ctrl Pts',(-0.482901662120691,-1.,-1.96792703422362));
#28663=CARTESIAN_POINT('Ctrl Pts',(-0.479349583074855,-1.,-1.96294933055943));
#28664=CARTESIAN_POINT('Ctrl Pts',(-0.475848034683176,-1.,-1.95796111148177));
#28665=CARTESIAN_POINT('Ctrl Pts',(-0.472397672264072,-1.,-1.95296148278133));
#28666=CARTESIAN_POINT('Ctrl Pts',(-0.468997482913135,-1.,-1.94794381136514));
#28667=CARTESIAN_POINT('Ctrl Pts',(-0.46564546202603,-1.,-1.9428979419619));
#28668=CARTESIAN_POINT('Ctrl Pts',(-0.462340031009056,-1.,-1.93781486640821));
#28669=CARTESIAN_POINT('Ctrl Pts',(-0.459081234547926,-1.,-1.93269066517934));
#28670=CARTESIAN_POINT('Ctrl Pts',(-0.455872005174371,-1.,-1.92753067150476));
#28671=CARTESIAN_POINT('Ctrl Pts',(-0.452719478359432,-1.,-1.92235380648502));
#28672=CARTESIAN_POINT('Ctrl Pts',(-0.449632260106662,-1.,-1.91718342555755));
#28673=CARTESIAN_POINT('Ctrl Pts',(-0.446617343485711,-1.,-1.9120369998112));
#28674=CARTESIAN_POINT('Ctrl Pts',(-0.443677556849151,-1.,-1.90691756144898));
#28675=CARTESIAN_POINT('Ctrl Pts',(-0.440807833704038,-1.,-1.90180124389086));
#28676=CARTESIAN_POINT('Ctrl Pts',(-0.437995003948244,-1.,-1.89663648956466));
#28677=CARTESIAN_POINT('Ctrl Pts',(-0.435225660963383,-1.,-1.89136993975504));
#28678=CARTESIAN_POINT('Ctrl Pts',(-0.432493038548748,-1.,-1.88596913666793));
#28679=CARTESIAN_POINT('Ctrl Pts',(-0.429803062482344,-1.,-1.88044229001832));
#28680=CARTESIAN_POINT('Ctrl Pts',(-0.427183828519102,-1.,-1.87486989291484));
#28681=CARTESIAN_POINT('Ctrl Pts',(-0.424678177291359,-1.,-1.86937803944323));
#28682=CARTESIAN_POINT('Ctrl Pts',(-0.422327307418275,-1.,-1.86408083334028));
#28683=CARTESIAN_POINT('Ctrl Pts',(-0.420157287975619,-1.,-1.85903281096686));
#28684=CARTESIAN_POINT('Ctrl Pts',(-0.418164129143534,-1.,-1.85417632856234));
#28685=CARTESIAN_POINT('Ctrl Pts',(-0.416300022038864,-1.,-1.84929312929882));
#28686=CARTESIAN_POINT('Ctrl Pts',(-0.41448743825434,-1.,-1.8440575707371));
#28687=CARTESIAN_POINT('Ctrl Pts',(-0.412633125322162,-1.,-1.83808953475839));
#28688=CARTESIAN_POINT('Ctrl Pts',(-0.410641256301675,-1.,-1.83100408895216));
#28689=CARTESIAN_POINT('Ctrl Pts',(-0.408428948108533,-1.,-1.8224702267854));
#28690=CARTESIAN_POINT('Ctrl Pts',(-0.405933518411838,-1.,-1.81223801813988));
#28691=CARTESIAN_POINT('Ctrl Pts',(-0.403107976170441,-1.,-1.80012077176221));
#28692=CARTESIAN_POINT('Ctrl Pts',(-0.39991940378308,-1.,-1.78598826347533));
#28693=CARTESIAN_POINT('Ctrl Pts',(-0.39634619612042,-1.,-1.7697556004756));
#28694=CARTESIAN_POINT('Ctrl Pts',(-0.392375812294307,-1.,-1.75137405313962));
#28695=CARTESIAN_POINT('Ctrl Pts',(-0.388877023509191,-1.,-1.7349317097561));
#28696=CARTESIAN_POINT('Ctrl Pts',(-0.38607079032701,-1.,-1.72162022246158));
#28697=CARTESIAN_POINT('Ctrl Pts',(-0.384119047315542,-1.,-1.71231062891958));
#28698=CARTESIAN_POINT('Ctrl Pts',(-0.383122945602004,-1.,-1.7075470150345));
#28699=CARTESIAN_POINT('',(-0.163289472382896,-1.,-1.74236521665491));
#28700=CARTESIAN_POINT('Origin',(0.,-1.,0.));
#28701=CARTESIAN_POINT('',(-0.0694764450219581,-1.,-2.19890268624765));
#28702=CARTESIAN_POINT('Ctrl Pts',(-0.163289472382896,-1.,-1.74236521665491));
#28703=CARTESIAN_POINT('Ctrl Pts',(-0.163814161002002,-1.,-1.7472034950333));
#28704=CARTESIAN_POINT('Ctrl Pts',(-0.164834765707158,-1.,-1.75666056638427));
#28705=CARTESIAN_POINT('Ctrl Pts',(-0.1662793551464,-1.,-1.77018771684844));
#28706=CARTESIAN_POINT('Ctrl Pts',(-0.168032772805197,-1.,-1.7869064998507));
#28707=CARTESIAN_POINT('Ctrl Pts',(-0.169936923904608,-1.,-1.80561530629706));
#28708=CARTESIAN_POINT('Ctrl Pts',(-0.171554770204119,-1.,-1.82215766811545));
#28709=CARTESIAN_POINT('Ctrl Pts',(-0.1728894428919,-1.,-1.83658380527692));
#28710=CARTESIAN_POINT('Ctrl Pts',(-0.173946627587731,-1.,-1.8489811319852));
#28711=CARTESIAN_POINT('Ctrl Pts',(-0.17473525927603,-1.,-1.85948367088837));
#28712=CARTESIAN_POINT('Ctrl Pts',(-0.175268337590758,-1.,-1.86828349694799));
#28713=CARTESIAN_POINT('Ctrl Pts',(-0.175563480746485,-1.,-1.87563767773588));
#28714=CARTESIAN_POINT('Ctrl Pts',(-0.175644148889699,-1.,-1.88188663145367));
#28715=CARTESIAN_POINT('Ctrl Pts',(-0.175538155840648,-1.,-1.88742606273259));
#28716=CARTESIAN_POINT('Ctrl Pts',(-0.175274276190844,-1.,-1.892646301985));
#28717=CARTESIAN_POINT('Ctrl Pts',(-0.174879405091263,-1.,-1.89788101117132));
#28718=CARTESIAN_POINT('Ctrl Pts',(-0.174375518661085,-1.,-1.90335253862834));
#28719=CARTESIAN_POINT('Ctrl Pts',(-0.173776635257817,-1.,-1.90911693975267));
#28720=CARTESIAN_POINT('Ctrl Pts',(-0.173090695383496,-1.,-1.91511429159527));
#28721=CARTESIAN_POINT('Ctrl Pts',(-0.172321621259514,-1.,-1.9212233439798));
#28722=CARTESIAN_POINT('Ctrl Pts',(-0.171471191532988,-1.,-1.92731093582036));
#28723=CARTESIAN_POINT('Ctrl Pts',(-0.170541253116202,-1.,-1.93329183155539));
#28724=CARTESIAN_POINT('Ctrl Pts',(-0.169534904817491,-1.,-1.93915639211581));
#28725=CARTESIAN_POINT('Ctrl Pts',(-0.168455741607556,-1.,-1.94493757756931));
#28726=CARTESIAN_POINT('Ctrl Pts',(-0.167307501784475,-1.,-1.95069027794294));
#28727=CARTESIAN_POINT('Ctrl Pts',(-0.166093592002812,-1.,-1.9564675971873));
#28728=CARTESIAN_POINT('Ctrl Pts',(-0.164816568920269,-1.,-1.96229379940136));
#28729=CARTESIAN_POINT('Ctrl Pts',(-0.163478185457734,-1.,-1.96816512677967));
#28730=CARTESIAN_POINT('Ctrl Pts',(-0.162079693556289,-1.,-1.97406280235188));
#28731=CARTESIAN_POINT('Ctrl Pts',(-0.160622060784611,-1.,-1.97996195437559));
#28732=CARTESIAN_POINT('Ctrl Pts',(-0.159106226437299,-1.,-1.98584238283292));
#28733=CARTESIAN_POINT('Ctrl Pts',(-0.157533331459227,-1.,-1.99169810931908));
#28734=CARTESIAN_POINT('Ctrl Pts',(-0.155904629548783,-1.,-1.99753284771497));
#28735=CARTESIAN_POINT('Ctrl Pts',(-0.154221403049722,-1.,-2.00335565310543));
#28736=CARTESIAN_POINT('Ctrl Pts',(-0.15248488362145,-1.,-2.00917680318424));
#28737=CARTESIAN_POINT('Ctrl Pts',(-0.150696157673078,-1.,-2.01500291940238));
#28738=CARTESIAN_POINT('Ctrl Pts',(-0.148856124775337,-1.,-2.02083464969894));
#28739=CARTESIAN_POINT('Ctrl Pts',(-0.146965557332583,-1.,-2.02666926182017));
#28740=CARTESIAN_POINT('Ctrl Pts',(-0.145025140186057,-1.,-2.03250223739942));
#28741=CARTESIAN_POINT('Ctrl Pts',(-0.143035515058209,-1.,-2.03832911025912));
#28742=CARTESIAN_POINT('Ctrl Pts',(-0.140997332152546,-1.,-2.04414757947916));
#28743=CARTESIAN_POINT('Ctrl Pts',(-0.138911255368966,-1.,-2.04995762001328));
#28744=CARTESIAN_POINT('Ctrl Pts',(-0.136777941218044,-1.,-2.05576044414264));
#28745=CARTESIAN_POINT('Ctrl Pts',(-0.134598026192106,-1.,-2.06155781517842));
#28746=CARTESIAN_POINT('Ctrl Pts',(-0.13237211154771,-1.,-2.06735123910326));
#28747=CARTESIAN_POINT('Ctrl Pts',(-0.130100748328403,-1.,-2.07314114713063));
#28748=CARTESIAN_POINT('Ctrl Pts',(-0.12778444527612,-1.,-2.07892715110987));
#28749=CARTESIAN_POINT('Ctrl Pts',(-0.125423679412061,-1.,-2.08470840653643));
#28750=CARTESIAN_POINT('Ctrl Pts',(-0.123018905621083,-1.,-2.09048392424825));
#28751=CARTESIAN_POINT('Ctrl Pts',(-0.120570567965122,-1.,-2.0962529286773));
#28752=CARTESIAN_POINT('Ctrl Pts',(-0.118079107988355,-1.,-2.102015121329));
#28753=CARTESIAN_POINT('Ctrl Pts',(-0.115544957687926,-1.,-2.10777050261309));
#28754=CARTESIAN_POINT('Ctrl Pts',(-0.112968534419737,-1.,-2.11351924490306));
#28755=CARTESIAN_POINT('Ctrl Pts',(-0.110350236135025,-1.,-2.11926155590865));
#28756=CARTESIAN_POINT('Ctrl Pts',(-0.10769043523109,-1.,-2.12499752307));
#28757=CARTESIAN_POINT('Ctrl Pts',(-0.104989479152739,-1.,-2.13072704887293));
#28758=CARTESIAN_POINT('Ctrl Pts',(-0.1022477005561,-1.,-2.13644992667165));
#28759=CARTESIAN_POINT('Ctrl Pts',(-0.0994654261990915,-1.,-2.14216588396025));
#28760=CARTESIAN_POINT('Ctrl Pts',(-0.0966429852305459,-1.,-2.14787463531795));
#28761=CARTESIAN_POINT('Ctrl Pts',(-0.0937807218867643,-1.,-2.1535759397817));
#28762=CARTESIAN_POINT('Ctrl Pts',(-0.0908789888107265,-1.,-2.15926961544516));
#28763=CARTESIAN_POINT('Ctrl Pts',(-0.0879381291386923,-1.,-2.16495552645014));
#28764=CARTESIAN_POINT('Ctrl Pts',(-0.0849584620835372,-1.,-2.17063357870952));
#28765=CARTESIAN_POINT('Ctrl Pts',(-0.0819402680872765,-1.,-2.176303712113));
#28766=CARTESIAN_POINT('Ctrl Pts',(-0.0788837727685243,-1.,-2.18196589448887));
#28767=CARTESIAN_POINT('Ctrl Pts',(-0.0757891465836148,-1.,-2.1876201139953));
#28768=CARTESIAN_POINT('Ctrl Pts',(-0.0732830357306725,-1.,-2.19213712013662));
#28769=CARTESIAN_POINT('Ctrl Pts',(-0.0713863779526154,-1.,-2.19552129484002));
#28770=CARTESIAN_POINT('Ctrl Pts',(-0.070114353632549,-1.,-2.19777582085423));
#28771=CARTESIAN_POINT('Ctrl Pts',(-0.0694764450219581,-1.,-2.19890268624765));
#28772=CARTESIAN_POINT('',(0.0694764450219584,-1.,-2.19890268624765));
#28773=CARTESIAN_POINT('',(-0.0694764450219581,-1.,-2.19890268624765));
#28774=CARTESIAN_POINT('',(0.163289472382896,-1.,-1.74236521665491));
#28775=CARTESIAN_POINT('Ctrl Pts',(0.0694764450219584,-1.,-2.19890268624765));
#28776=CARTESIAN_POINT('Ctrl Pts',(0.0701143536324926,-1.,-2.19777582085261));
#28777=CARTESIAN_POINT('Ctrl Pts',(0.0713863779524627,-1.,-2.19552129483562));
#28778=CARTESIAN_POINT('Ctrl Pts',(0.0732830357304276,-1.,-2.19213712012956));
#28779=CARTESIAN_POINT('Ctrl Pts',(0.0757891465833411,-1.,-2.1876201139874));
#28780=CARTESIAN_POINT('Ctrl Pts',(0.0788837727683228,-1.,-2.18196589448304));
#28781=CARTESIAN_POINT('Ctrl Pts',(0.0819402680871939,-1.,-2.1763037121106));
#28782=CARTESIAN_POINT('Ctrl Pts',(0.0849584620835643,-1.,-2.17063357871031));
#28783=CARTESIAN_POINT('Ctrl Pts',(0.0879381291387823,-1.,-2.16495552645275));
#28784=CARTESIAN_POINT('Ctrl Pts',(0.0908789888108266,-1.,-2.15926961544808));
#28785=CARTESIAN_POINT('Ctrl Pts',(0.0937807218868345,-1.,-2.15357593978377));
#28786=CARTESIAN_POINT('Ctrl Pts',(0.0966429852305689,-1.,-2.14787463531864));
#28787=CARTESIAN_POINT('Ctrl Pts',(0.0994654261990743,-1.,-2.14216588395974));
#28788=CARTESIAN_POINT('Ctrl Pts',(0.102247700556064,-1.,-2.13644992667052));
#28789=CARTESIAN_POINT('Ctrl Pts',(0.104989479152703,-1.,-2.1307270488718));
#28790=CARTESIAN_POINT('Ctrl Pts',(0.107690435231068,-1.,-2.12499752306927));
#28791=CARTESIAN_POINT('Ctrl Pts',(0.11035023613502,-1.,-2.11926155590849));
#28792=CARTESIAN_POINT('Ctrl Pts',(0.112968534419746,-1.,-2.11351924490335));
#28793=CARTESIAN_POINT('Ctrl Pts',(0.11554495768794,-1.,-2.10777050261359));
#28794=CARTESIAN_POINT('Ctrl Pts',(0.118079107988368,-1.,-2.10201512132945));
#28795=CARTESIAN_POINT('Ctrl Pts',(0.120570567965129,-1.,-2.09625292867756));
#28796=CARTESIAN_POINT('Ctrl Pts',(0.123018905621083,-1.,-2.09048392424826));
#28797=CARTESIAN_POINT('Ctrl Pts',(0.125423679412058,-1.,-2.08470840653628));
#28798=CARTESIAN_POINT('Ctrl Pts',(0.127784445276116,-1.,-2.07892715110967));
#28799=CARTESIAN_POINT('Ctrl Pts',(0.1301007483284,-1.,-2.07314114713047));
#28800=CARTESIAN_POINT('Ctrl Pts',(0.13237211154771,-1.,-2.06735123910319));
#28801=CARTESIAN_POINT('Ctrl Pts',(0.134598026192107,-1.,-2.06155781517844));
#28802=CARTESIAN_POINT('Ctrl Pts',(0.136777941218044,-1.,-2.0557604441427));
#28803=CARTESIAN_POINT('Ctrl Pts',(0.138911255368966,-1.,-2.04995762001333));
#28804=CARTESIAN_POINT('Ctrl Pts',(0.140997332152545,-1.,-2.04414757947919));
#28805=CARTESIAN_POINT('Ctrl Pts',(0.143035515058208,-1.,-2.03832911025913));
#28806=CARTESIAN_POINT('Ctrl Pts',(0.145025140186058,-1.,-2.03250223739941));
#28807=CARTESIAN_POINT('Ctrl Pts',(0.146965557332586,-1.,-2.02666926182017));
#28808=CARTESIAN_POINT('Ctrl Pts',(0.148856124775343,-1.,-2.02083464969897));
#28809=CARTESIAN_POINT('Ctrl Pts',(0.150696157673084,-1.,-2.01500291940243));
#28810=CARTESIAN_POINT('Ctrl Pts',(0.152484883621452,-1.,-2.00917680318426));
#28811=CARTESIAN_POINT('Ctrl Pts',(0.154221403049719,-1.,-2.00335565310539));
#28812=CARTESIAN_POINT('Ctrl Pts',(0.155904629548774,-1.,-1.99753284771487));
#28813=CARTESIAN_POINT('Ctrl Pts',(0.157533331459215,-1.,-1.99169810931893));
#28814=CARTESIAN_POINT('Ctrl Pts',(0.159106226437288,-1.,-1.98584238283279));
#28815=CARTESIAN_POINT('Ctrl Pts',(0.16062206078461,-1.,-1.97996195437557));
#28816=CARTESIAN_POINT('Ctrl Pts',(0.162079693556302,-1.,-1.97406280235204));
#28817=CARTESIAN_POINT('Ctrl Pts',(0.16347818545776,-1.,-1.96816512678));
#28818=CARTESIAN_POINT('Ctrl Pts',(0.1648165689203,-1.,-1.96229379940174));
#28819=CARTESIAN_POINT('Ctrl Pts',(0.166093592002833,-1.,-1.95646759718755));
#28820=CARTESIAN_POINT('Ctrl Pts',(0.167307501784469,-1.,-1.95069027794286));
#28821=CARTESIAN_POINT('Ctrl Pts',(0.168455741607516,-1.,-1.94493757756879));
#28822=CARTESIAN_POINT('Ctrl Pts',(0.169534904817425,-1.,-1.93915639211497));
#28823=CARTESIAN_POINT('Ctrl Pts',(0.170541253116136,-1.,-1.93329183155455));
#28824=CARTESIAN_POINT('Ctrl Pts',(0.17147119153296,-1.,-1.92731093582));
#28825=CARTESIAN_POINT('Ctrl Pts',(0.172321621259557,-1.,-1.92122334398034));
#28826=CARTESIAN_POINT('Ctrl Pts',(0.173090695383619,-1.,-1.91511429159681));
#28827=CARTESIAN_POINT('Ctrl Pts',(0.173776635257984,-1.,-1.90911693975475));
#28828=CARTESIAN_POINT('Ctrl Pts',(0.174375518661222,-1.,-1.90335253863003));
#28829=CARTESIAN_POINT('Ctrl Pts',(0.174879405091277,-1.,-1.89788101117148));
#28830=CARTESIAN_POINT('Ctrl Pts',(0.175274276190664,-1.,-1.89264630198279));
#28831=CARTESIAN_POINT('Ctrl Pts',(0.175538155840286,-1.,-1.88742606272818));
#28832=CARTESIAN_POINT('Ctrl Pts',(0.175644148889271,-1.,-1.88188663144846));
#28833=CARTESIAN_POINT('Ctrl Pts',(0.175563480746205,-1.,-1.87563767773249));
#28834=CARTESIAN_POINT('Ctrl Pts',(0.175268337590901,-1.,-1.86828349694972));
#28835=CARTESIAN_POINT('Ctrl Pts',(0.174735259276856,-1.,-1.85948367089838));
#28836=CARTESIAN_POINT('Ctrl Pts',(0.173946627589401,-1.,-1.84898113200543));
#28837=CARTESIAN_POINT('Ctrl Pts',(0.17288944289442,-1.,-1.83658380530747));
#28838=CARTESIAN_POINT('Ctrl Pts',(0.171554770207306,-1.,-1.82215766815414));
#28839=CARTESIAN_POINT('Ctrl Pts',(0.169936923908078,-1.,-1.80561530633924));
#28840=CARTESIAN_POINT('Ctrl Pts',(0.16803277280837,-1.,-1.78690649988931));
#28841=CARTESIAN_POINT('Ctrl Pts',(0.166279355148738,-1.,-1.77018771687692));
#28842=CARTESIAN_POINT('Ctrl Pts',(0.164834765708484,-1.,-1.75666056640041));
#28843=CARTESIAN_POINT('Ctrl Pts',(0.163814161002474,-1.,-1.74720349503904));
#28844=CARTESIAN_POINT('Ctrl Pts',(0.163289472382896,-1.,-1.74236521665491));
#28845=CARTESIAN_POINT('',(0.383122945602004,-1.,-1.7075470150345));
#28846=CARTESIAN_POINT('Origin',(0.,-1.,0.));
#28847=CARTESIAN_POINT('',(0.61342227326009,-1.,-2.11275013067528));
#28848=CARTESIAN_POINT('Ctrl Pts',(0.383122945602004,-1.,-1.7075470150345));
#28849=CARTESIAN_POINT('Ctrl Pts',(0.384119047314215,-1.,-1.71231062891398));
#28850=CARTESIAN_POINT('Ctrl Pts',(0.386070790323281,-1.,-1.72162022244582));
#28851=CARTESIAN_POINT('Ctrl Pts',(0.388877023502615,-1.,-1.73493170972829));
#28852=CARTESIAN_POINT('Ctrl Pts',(0.392375812285395,-1.,-1.75137405310193));
#28853=CARTESIAN_POINT('Ctrl Pts',(0.396346196110688,-1.,-1.76975560043442));
#28854=CARTESIAN_POINT('Ctrl Pts',(0.399919403774155,-1.,-1.78598826343754));
#28855=CARTESIAN_POINT('Ctrl Pts',(0.403107976163396,-1.,-1.80012077173238));
#28856=CARTESIAN_POINT('Ctrl Pts',(0.405933518407175,-1.,-1.81223801812013));
#28857=CARTESIAN_POINT('Ctrl Pts',(0.408428948106227,-1.,-1.82247022677562));
#28858=CARTESIAN_POINT('Ctrl Pts',(0.410641256301276,-1.,-1.83100408895047));
#28859=CARTESIAN_POINT('Ctrl Pts',(0.412633125322945,-1.,-1.8380895347617));
#28860=CARTESIAN_POINT('Ctrl Pts',(0.414487438255542,-1.,-1.84405757074218));
#28861=CARTESIAN_POINT('Ctrl Pts',(0.416300022039885,-1.,-1.84929312930314));
#28862=CARTESIAN_POINT('Ctrl Pts',(0.418164129144045,-1.,-1.8541763285645));
#28863=CARTESIAN_POINT('Ctrl Pts',(0.420157287975583,-1.,-1.8590328109667));
#28864=CARTESIAN_POINT('Ctrl Pts',(0.422327307417884,-1.,-1.86408083333863));
#28865=CARTESIAN_POINT('Ctrl Pts',(0.424678177290876,-1.,-1.8693780394412));
#28866=CARTESIAN_POINT('Ctrl Pts',(0.427183828518743,-1.,-1.87486989291334));
#28867=CARTESIAN_POINT('Ctrl Pts',(0.429803062482217,-1.,-1.88044229001779));
#28868=CARTESIAN_POINT('Ctrl Pts',(0.432493038548833,-1.,-1.88596913666828));
#28869=CARTESIAN_POINT('Ctrl Pts',(0.43522566096358,-1.,-1.89136993975585));
#28870=CARTESIAN_POINT('Ctrl Pts',(0.437995003948443,-1.,-1.89663648956549));
#28871=CARTESIAN_POINT('Ctrl Pts',(0.44080783370416,-1.,-1.90180124389137));
#28872=CARTESIAN_POINT('Ctrl Pts',(0.44367755684917,-1.,-1.90691756144906));
#28873=CARTESIAN_POINT('Ctrl Pts',(0.446617343485651,-1.,-1.91203699981095));
#28874=CARTESIAN_POINT('Ctrl Pts',(0.449632260106572,-1.,-1.91718342555717));
#28875=CARTESIAN_POINT('Ctrl Pts',(0.452719478359356,-1.,-1.9223538064847));
#28876=CARTESIAN_POINT('Ctrl Pts',(0.455872005174335,-1.,-1.92753067150461));
#28877=CARTESIAN_POINT('Ctrl Pts',(0.459081234547931,-1.,-1.93269066517936));
#28878=CARTESIAN_POINT('Ctrl Pts',(0.462340031009087,-1.,-1.93781486640834));
#28879=CARTESIAN_POINT('Ctrl Pts',(0.465645462026064,-1.,-1.94289794196205));
#28880=CARTESIAN_POINT('Ctrl Pts',(0.468997482913158,-1.,-1.94794381136524));
#28881=CARTESIAN_POINT('Ctrl Pts',(0.472397672264079,-1.,-1.95296148278136));
#28882=CARTESIAN_POINT('Ctrl Pts',(0.475848034683171,-1.,-1.95796111148175));
#28883=CARTESIAN_POINT('Ctrl Pts',(0.479349583074846,-1.,-1.96294933055938));
#28884=CARTESIAN_POINT('Ctrl Pts',(0.482901662120686,-1.,-1.96792703422358));
#28885=CARTESIAN_POINT('Ctrl Pts',(0.486502692907661,-1.,-1.97289186263272));
#28886=CARTESIAN_POINT('Ctrl Pts',(0.490150627860955,-1.,-1.97783973019229));
#28887=CARTESIAN_POINT('Ctrl Pts',(0.493843476541492,-1.,-1.9827665876182));
#28888=CARTESIAN_POINT('Ctrl Pts',(0.497579909545564,-1.,-1.98767044752929));
#28889=CARTESIAN_POINT('Ctrl Pts',(0.501359287727129,-1.,-1.9925514912615));
#28890=CARTESIAN_POINT('Ctrl Pts',(0.505181361323011,-1.,-1.99741107463567));
#28891=CARTESIAN_POINT('Ctrl Pts',(0.509046069886152,-1.,-2.00225107134733));
#28892=CARTESIAN_POINT('Ctrl Pts',(0.512953306961813,-1.,-2.00707309946955));
#28893=CARTESIAN_POINT('Ctrl Pts',(0.516902681728733,-1.,-2.01187773939257));
#28894=CARTESIAN_POINT('Ctrl Pts',(0.520893590399428,-1.,-2.01666477917306));
#28895=CARTESIAN_POINT('Ctrl Pts',(0.524925318333518,-1.,-2.02143356304712));
#28896=CARTESIAN_POINT('Ctrl Pts',(0.52899712724191,-1.,-2.02618329083289));
#28897=CARTESIAN_POINT('Ctrl Pts',(0.533108355132905,-1.,-2.03091336214401));
#28898=CARTESIAN_POINT('Ctrl Pts',(0.537258489833134,-1.,-2.03562362953993));
#28899=CARTESIAN_POINT('Ctrl Pts',(0.54144712061552,-1.,-2.0403142269048));
#28900=CARTESIAN_POINT('Ctrl Pts',(0.545673903817348,-1.,-2.0449854471456));
#28901=CARTESIAN_POINT('Ctrl Pts',(0.549938525150342,-1.,-2.04963761077974));
#28902=CARTESIAN_POINT('Ctrl Pts',(0.554240657464109,-1.,-2.05427091604482));
#28903=CARTESIAN_POINT('Ctrl Pts',(0.558579940185467,-1.,-2.05888537756571));
#28904=CARTESIAN_POINT('Ctrl Pts',(0.562955993082574,-1.,-2.06348090160697));
#28905=CARTESIAN_POINT('Ctrl Pts',(0.567368421181229,-1.,-2.06805732997383));
#28906=CARTESIAN_POINT('Ctrl Pts',(0.571816823242411,-1.,-2.07261449292758));
#28907=CARTESIAN_POINT('Ctrl Pts',(0.576300797416274,-1.,-2.07715226767361));
#28908=CARTESIAN_POINT('Ctrl Pts',(0.580819952107256,-1.,-2.08167059018138));
#28909=CARTESIAN_POINT('Ctrl Pts',(0.585373918990895,-1.,-2.086169437277));
#28910=CARTESIAN_POINT('Ctrl Pts',(0.589962365403189,-1.,-2.09064881812053));
#28911=CARTESIAN_POINT('Ctrl Pts',(0.594585006052823,-1.,-2.09510876220501));
#28912=CARTESIAN_POINT('Ctrl Pts',(0.599241616422144,-1.,-2.09954930865331));
#28913=CARTESIAN_POINT('Ctrl Pts',(0.603932030738212,-1.,-2.10397049887709));
#28914=CARTESIAN_POINT('Ctrl Pts',(0.607711315456826,-1.,-2.10749199615859));
#28915=CARTESIAN_POINT('Ctrl Pts',(0.610560911691113,-1.,-2.11012443807661));
#28916=CARTESIAN_POINT('Ctrl Pts',(0.61246736556225,-1.,-2.11187554260142));
#28917=CARTESIAN_POINT('Ctrl Pts',(0.61342227326009,-1.,-2.11275013067528));
#28918=CARTESIAN_POINT('',(0.745574324794401,-1.,-2.0698113262342));
#28919=CARTESIAN_POINT('',(0.61342227326009,-1.,-2.11275013067528));
#28920=CARTESIAN_POINT('',(0.693717979106306,-1.,-1.60662857109684));
#28921=CARTESIAN_POINT('Ctrl Pts',(0.745574324794401,-1.,-2.0698113262342));
#28922=CARTESIAN_POINT('Ctrl Pts',(0.74583279137781,-1.,-2.06854248895575));
#28923=CARTESIAN_POINT('Ctrl Pts',(0.746345871542695,-1.,-2.06600523016401));
#28924=CARTESIAN_POINT('Ctrl Pts',(0.747103932785504,-1.,-2.06220058927162));
#28925=CARTESIAN_POINT('Ctrl Pts',(0.748091554181101,-1.,-2.05713023030263));
#28926=CARTESIAN_POINT('Ctrl Pts',(0.749287468663053,-1.,-2.05079645591606));
#28927=CARTESIAN_POINT('Ctrl Pts',(0.750444657874758,-1.,-2.04446689147754));
#28928=CARTESIAN_POINT('Ctrl Pts',(0.751562963361383,-1.,-2.03814160092173));
#28929=CARTESIAN_POINT('Ctrl Pts',(0.752642180488104,-1.,-2.03182068456467));
#28930=CARTESIAN_POINT('Ctrl Pts',(0.753682061113765,-1.,-2.02550428623587));
#28931=CARTESIAN_POINT('Ctrl Pts',(0.75468233072352,-1.,-2.01919259406003));
#28932=CARTESIAN_POINT('Ctrl Pts',(0.7556427049581,-1.,-2.01288584328149));
#28933=CARTESIAN_POINT('Ctrl Pts',(0.756562904646496,-1.,-2.00658431587682));
#28934=CARTESIAN_POINT('Ctrl Pts',(0.757442676862341,-1.,-2.00028834739072));
#28935=CARTESIAN_POINT('Ctrl Pts',(0.758281796766377,-1.,-1.9939983109871));
#28936=CARTESIAN_POINT('Ctrl Pts',(0.759080037802242,-1.,-1.98771456680806));
#28937=CARTESIAN_POINT('Ctrl Pts',(0.759837147452135,-1.,-1.98143741418156));
#28938=CARTESIAN_POINT('Ctrl Pts',(0.760552825409855,-1.,-1.97516705321521));
#28939=CARTESIAN_POINT('Ctrl Pts',(0.761226690483986,-1.,-1.96890351582545));
#28940=CARTESIAN_POINT('Ctrl Pts',(0.761858300014575,-1.,-1.96264672744229));
#28941=CARTESIAN_POINT('Ctrl Pts',(0.762447203806263,-1.,-1.95639665309893));
#28942=CARTESIAN_POINT('Ctrl Pts',(0.762992990878774,-1.,-1.95015342590025));
#28943=CARTESIAN_POINT('Ctrl Pts',(0.76349533353858,-1.,-1.94391746617626));
#28944=CARTESIAN_POINT('Ctrl Pts',(0.763954049121393,-1.,-1.93768964875867));
#28945=CARTESIAN_POINT('Ctrl Pts',(0.764369010673889,-1.,-1.93147105496367));
#28946=CARTESIAN_POINT('Ctrl Pts',(0.764740025488189,-1.,-1.92526263537041));
#28947=CARTESIAN_POINT('Ctrl Pts',(0.765066729667095,-1.,-1.91906491634197));
#28948=CARTESIAN_POINT('Ctrl Pts',(0.765348465884739,-1.,-1.91287765805174));
#28949=CARTESIAN_POINT('Ctrl Pts',(0.765584196937936,-1.,-1.90669961402362));
#28950=CARTESIAN_POINT('Ctrl Pts',(0.765772772593395,-1.,-1.90052930393599));
#28951=CARTESIAN_POINT('Ctrl Pts',(0.765913193856979,-1.,-1.89436577771389));
#28952=CARTESIAN_POINT('Ctrl Pts',(0.76600483706209,-1.,-1.88820926433409));
#28953=CARTESIAN_POINT('Ctrl Pts',(0.766047794851868,-1.,-1.88206215302561));
#28954=CARTESIAN_POINT('Ctrl Pts',(0.766042837036759,-1.,-1.87592888967886));
#28955=CARTESIAN_POINT('Ctrl Pts',(0.765990708546111,-1.,-1.86981398314345));
#28956=CARTESIAN_POINT('Ctrl Pts',(0.765891519092557,-1.,-1.86372027063315));
#28957=CARTESIAN_POINT('Ctrl Pts',(0.765744212909305,-1.,-1.85764741390391));
#28958=CARTESIAN_POINT('Ctrl Pts',(0.765545710619023,-1.,-1.85158945130054));
#28959=CARTESIAN_POINT('Ctrl Pts',(0.765291664861971,-1.,-1.84553698875911));
#28960=CARTESIAN_POINT('Ctrl Pts',(0.764978057881687,-1.,-1.83948181064823));
#28961=CARTESIAN_POINT('Ctrl Pts',(0.764602549687845,-1.,-1.8334207722714));
#28962=CARTESIAN_POINT('Ctrl Pts',(0.764165902606055,-1.,-1.8273599120008));
#28963=CARTESIAN_POINT('Ctrl Pts',(0.763673465462854,-1.,-1.82131873145297));
#28964=CARTESIAN_POINT('Ctrl Pts',(0.763132003836783,-1.,-1.81532118405566));
#28965=CARTESIAN_POINT('Ctrl Pts',(0.762546129464036,-1.,-1.80938551463989));
#28966=CARTESIAN_POINT('Ctrl Pts',(0.761915336443515,-1.,-1.80351583877334));
#28967=CARTESIAN_POINT('Ctrl Pts',(0.761229695230359,-1.,-1.79768986997735));
#28968=CARTESIAN_POINT('Ctrl Pts',(0.760469555880425,-1.,-1.79185815610802));
#28969=CARTESIAN_POINT('Ctrl Pts',(0.759614401109868,-1.,-1.78596964884527));
#28970=CARTESIAN_POINT('Ctrl Pts',(0.75865062667738,-1.,-1.77999411220912));
#28971=CARTESIAN_POINT('Ctrl Pts',(0.757578264077238,-1.,-1.77394167108342));
#28972=CARTESIAN_POINT('Ctrl Pts',(0.756421896028403,-1.,-1.76789396003141));
#28973=CARTESIAN_POINT('Ctrl Pts',(0.755220979975262,-1.,-1.7619781724032));
#28974=CARTESIAN_POINT('Ctrl Pts',(0.75400925402848,-1.,-1.75631083600175));
#28975=CARTESIAN_POINT('Ctrl Pts',(0.752797683531377,-1.,-1.75095139468809));
#28976=CARTESIAN_POINT('Ctrl Pts',(0.751555614163629,-1.,-1.74585086852298));
#28977=CARTESIAN_POINT('Ctrl Pts',(0.75019343597954,-1.,-1.74080458266705));
#28978=CARTESIAN_POINT('Ctrl Pts',(0.748582462954854,-1.,-1.73550351679848));
#28979=CARTESIAN_POINT('Ctrl Pts',(0.746574710096436,-1.,-1.72958533647399));
#28980=CARTESIAN_POINT('Ctrl Pts',(0.744021445433764,-1.,-1.7226822991693));
#28981=CARTESIAN_POINT('Ctrl Pts',(0.740795162032087,-1.,-1.71447789751927));
#28982=CARTESIAN_POINT('Ctrl Pts',(0.736799665724771,-1.,-1.70473309006121));
#28983=CARTESIAN_POINT('Ctrl Pts',(0.731963238697195,-1.,-1.69326921975743));
#28984=CARTESIAN_POINT('Ctrl Pts',(0.726235967997433,-1.,-1.67996158455503));
#28985=CARTESIAN_POINT('Ctrl Pts',(0.719585433804282,-1.,-1.6647288055568));
#28986=CARTESIAN_POINT('Ctrl Pts',(0.711993139355394,-1.,-1.64752408832016));
#28987=CARTESIAN_POINT('Ctrl Pts',(0.705159151988319,-1.,-1.63216541664676));
#28988=CARTESIAN_POINT('Ctrl Pts',(0.699605146405088,-1.,-1.61974673472612));
#28989=CARTESIAN_POINT('Ctrl Pts',(0.695712097881194,-1.,-1.61106790958151));
#28990=CARTESIAN_POINT('Ctrl Pts',(0.693717979106306,-1.,-1.60662857109684));
#28991=CARTESIAN_POINT('',(0.892032620296855,-1.,-1.5055822144029));
#28992=CARTESIAN_POINT('Origin',(0.,-1.,0.));
#28993=CARTESIAN_POINT('',(1.23627494547115,-1.,-1.81978687191668));
#28994=CARTESIAN_POINT('Ctrl Pts',(0.892032620296855,-1.,-1.5055822144029));
#28995=CARTESIAN_POINT('Ctrl Pts',(0.894452006964543,-1.,-1.50980486806688));
#28996=CARTESIAN_POINT('Ctrl Pts',(0.89918504748351,-1.,-1.51805569590094));
#28997=CARTESIAN_POINT('Ctrl Pts',(0.905967409625651,-1.,-1.52984849887993));
#28998=CARTESIAN_POINT('Ctrl Pts',(0.914375919026456,-1.,-1.54440491149498));
#28999=CARTESIAN_POINT('Ctrl Pts',(0.923832188944341,-1.,-1.56065988578893));
#29000=CARTESIAN_POINT('Ctrl Pts',(0.932246680108685,-1.,-1.57499388382243));
#29001=CARTESIAN_POINT('Ctrl Pts',(0.939646377893399,-1.,-1.58744937487176));
#29002=CARTESIAN_POINT('Ctrl Pts',(0.946078063315257,-1.,-1.59810042043673));
#29003=CARTESIAN_POINT('Ctrl Pts',(0.951613284356035,-1.,-1.60706069896936));
#29004=CARTESIAN_POINT('Ctrl Pts',(0.95635442292067,-1.,-1.61449324337085));
#29005=CARTESIAN_POINT('Ctrl Pts',(0.960438326101728,-1.,-1.62061638140221));
#29006=CARTESIAN_POINT('Ctrl Pts',(0.964046107040535,-1.,-1.62571930670187));
#29007=CARTESIAN_POINT('Ctrl Pts',(0.967387853230345,-1.,-1.63013849959462));
#29008=CARTESIAN_POINT('Ctrl Pts',(0.970669715997509,-1.,-1.63420665729798));
#29009=CARTESIAN_POINT('Ctrl Pts',(0.974066058287418,-1.,-1.63820952658144));
#29010=CARTESIAN_POINT('Ctrl Pts',(0.977689794119416,-1.,-1.64233990826687));
#29011=CARTESIAN_POINT('Ctrl Pts',(0.981562530939489,-1.,-1.64665139190656));
#29012=CARTESIAN_POINT('Ctrl Pts',(0.98564262292082,-1.,-1.65110016612638));
#29013=CARTESIAN_POINT('Ctrl Pts',(0.989855627854164,-1.,-1.65559044289699));
#29014=CARTESIAN_POINT('Ctrl Pts',(0.994121836661305,-1.,-1.66001553809947));
#29015=CARTESIAN_POINT('Ctrl Pts',(0.998389654952757,-1.,-1.66430758030376));
#29016=CARTESIAN_POINT('Ctrl Pts',(1.00265091003727,-1.,-1.66846059277303));
#29017=CARTESIAN_POINT('Ctrl Pts',(1.00692206696414,-1.,-1.67250335383293));
#29018=CARTESIAN_POINT('Ctrl Pts',(1.01123236493511,-1.,-1.67648246776464));
#29019=CARTESIAN_POINT('Ctrl Pts',(1.01561026162773,-1.,-1.68044289894798));
#29020=CARTESIAN_POINT('Ctrl Pts',(1.02006795074201,-1.,-1.68440578021706));
#29021=CARTESIAN_POINT('Ctrl Pts',(1.02460180535255,-1.,-1.68836910178447));
#29022=CARTESIAN_POINT('Ctrl Pts',(1.02919977579147,-1.,-1.69231840863458));
#29023=CARTESIAN_POINT('Ctrl Pts',(1.03384646003588,-1.,-1.69623414782771));
#29024=CARTESIAN_POINT('Ctrl Pts',(1.03852922490789,-1.,-1.70010052930962));
#29025=CARTESIAN_POINT('Ctrl Pts',(1.04324363334554,-1.,-1.70391338707982));
#29026=CARTESIAN_POINT('Ctrl Pts',(1.04799085404995,-1.,-1.70767646263649));
#29027=CARTESIAN_POINT('Ctrl Pts',(1.05277517202855,-1.,-1.71139783543989));
#29028=CARTESIAN_POINT('Ctrl Pts',(1.05760163192479,-1.,-1.7150865442702));
#29029=CARTESIAN_POINT('Ctrl Pts',(1.06247324680647,-1.,-1.71874858456904));
#29030=CARTESIAN_POINT('Ctrl Pts',(1.06738966975462,-1.,-1.72238500928453));
#29031=CARTESIAN_POINT('Ctrl Pts',(1.07234866990252,-1.,-1.72599406198488));
#29032=CARTESIAN_POINT('Ctrl Pts',(1.0773470373727,-1.,-1.72957248977424));
#29033=CARTESIAN_POINT('Ctrl Pts',(1.08238162784749,-1.,-1.73311705663407));
#29034=CARTESIAN_POINT('Ctrl Pts',(1.08745056285427,-1.,-1.73662628326091));
#29035=CARTESIAN_POINT('Ctrl Pts',(1.09255329056493,-1.,-1.74010053962247));
#29036=CARTESIAN_POINT('Ctrl Pts',(1.09768999241225,-1.,-1.74354119236208));
#29037=CARTESIAN_POINT('Ctrl Pts',(1.10286118991143,-1.,-1.74695004214923));
#29038=CARTESIAN_POINT('Ctrl Pts',(1.10806728183007,-1.,-1.7503286607592));
#29039=CARTESIAN_POINT('Ctrl Pts',(1.11330807582551,-1.,-1.7536777209463));
#29040=CARTESIAN_POINT('Ctrl Pts',(1.11858293216763,-1.,-1.75699720772105));
#29041=CARTESIAN_POINT('Ctrl Pts',(1.12389096855086,-1.,-1.76028671825096));
#29042=CARTESIAN_POINT('Ctrl Pts',(1.12923123555075,-1.,-1.7635457196617));
#29043=CARTESIAN_POINT('Ctrl Pts',(1.1346029180462,-1.,-1.76677384551862));
#29044=CARTESIAN_POINT('Ctrl Pts',(1.14000548336975,-1.,-1.76997111386769));
#29045=CARTESIAN_POINT('Ctrl Pts',(1.1454385822692,-1.,-1.77313777896194));
#29046=CARTESIAN_POINT('Ctrl Pts',(1.15090197841514,-1.,-1.7762742255701));
#29047=CARTESIAN_POINT('Ctrl Pts',(1.15639547194698,-1.,-1.77938085564275));
#29048=CARTESIAN_POINT('Ctrl Pts',(1.16191881298499,-1.,-1.78245795881009));
#29049=CARTESIAN_POINT('Ctrl Pts',(1.16747166312303,-1.,-1.78550566040443));
#29050=CARTESIAN_POINT('Ctrl Pts',(1.17305363177328,-1.,-1.78852398877617));
#29051=CARTESIAN_POINT('Ctrl Pts',(1.17866429440809,-1.,-1.79151291552689));
#29052=CARTESIAN_POINT('Ctrl Pts',(1.18430321697432,-1.,-1.79447240321515));
#29053=CARTESIAN_POINT('Ctrl Pts',(1.18996997934445,-1.,-1.79740245923478));
#29054=CARTESIAN_POINT('Ctrl Pts',(1.19566418930242,-1.,-1.80030314369879));
#29055=CARTESIAN_POINT('Ctrl Pts',(1.20138548938974,-1.,-1.80317454838603));
#29056=CARTESIAN_POINT('Ctrl Pts',(1.20713356605475,-1.,-1.80601678480707));
#29057=CARTESIAN_POINT('Ctrl Pts',(1.21290815708314,-1.,-1.80882996917129));
#29058=CARTESIAN_POINT('Ctrl Pts',(1.21870906103557,-1.,-1.81161420806656));
#29059=CARTESIAN_POINT('Ctrl Pts',(1.2245361330495,-1.,-1.81436959210434));
#29060=CARTESIAN_POINT('Ctrl Pts',(1.2292186489137,-1.,-1.8165508718364));
#29061=CARTESIAN_POINT('Ctrl Pts',(1.2327422452705,-1.,-1.81817389921279));
#29062=CARTESIAN_POINT('Ctrl Pts',(1.23509651170476,-1.,-1.81925017193666));
#29063=CARTESIAN_POINT('Ctrl Pts',(1.23627494547115,-1.,-1.81978687191668));
#29064=CARTESIAN_POINT('',(1.34869019493419,-1.,-1.73811241238545));
#29065=CARTESIAN_POINT('',(1.23627494547115,-1.,-1.81978687191668));
#29066=CARTESIAN_POINT('',(1.15624053661742,-1.,-1.31362392696032));
#29067=CARTESIAN_POINT('Ctrl Pts',(1.34869019493419,-1.,-1.73811241238545));
#29068=CARTESIAN_POINT('Ctrl Pts',(1.34854391898045,-1.,-1.73682580585691));
#29069=CARTESIAN_POINT('Ctrl Pts',(1.34824783112887,-1.,-1.73425417885907));
#29070=CARTESIAN_POINT('Ctrl Pts',(1.34779309152035,-1.,-1.7304014965394));
#29071=CARTESIAN_POINT('Ctrl Pts',(1.34716554819527,-1.,-1.72527410680674));
#29072=CARTESIAN_POINT('Ctrl Pts',(1.34634568653227,-1.,-1.7188807715049));
#29073=CARTESIAN_POINT('Ctrl Pts',(1.34549029589416,-1.,-1.71250340686822));
#29074=CARTESIAN_POINT('Ctrl Pts',(1.34459924533831,-1.,-1.70614212266738));
#29075=CARTESIAN_POINT('Ctrl Pts',(1.34367237124483,-1.,-1.69979707754427));
#29076=CARTESIAN_POINT('Ctrl Pts',(1.34270948206319,-1.,-1.6934684849687));
#29077=CARTESIAN_POINT('Ctrl Pts',(1.341710374848,-1.,-1.68715660868764));
#29078=CARTESIAN_POINT('Ctrl Pts',(1.34067485185203,-1.,-1.68086176030362));
#29079=CARTESIAN_POINT('Ctrl Pts',(1.3396027347034,-1.,-1.67458429426086));
#29080=CARTESIAN_POINT('Ctrl Pts',(1.33849388654388,-1.,-1.66832460783989));
#29081=CARTESIAN_POINT('Ctrl Pts',(1.33734820885262,-1.,-1.66208312541983));
#29082=CARTESIAN_POINT('Ctrl Pts',(1.33616559745172,-1.,-1.65586025952593));
#29083=CARTESIAN_POINT('Ctrl Pts',(1.33494590467993,-1.,-1.6496563728683));
#29084=CARTESIAN_POINT('Ctrl Pts',(1.33368890676572,-1.,-1.6434717485603));
#29085=CARTESIAN_POINT('Ctrl Pts',(1.33239425103724,-1.,-1.63730653475089));
#29086=CARTESIAN_POINT('Ctrl Pts',(1.33106149345645,-1.,-1.63116079730923));
#29087=CARTESIAN_POINT('Ctrl Pts',(1.3296901950568,-1.,-1.62503464209797));
#29088=CARTESIAN_POINT('Ctrl Pts',(1.32828000610449,-1.,-1.61892832270724));
#29089=CARTESIAN_POINT('Ctrl Pts',(1.32683074483356,-1.,-1.6128423401575));
#29090=CARTESIAN_POINT('Ctrl Pts',(1.32534250785782,-1.,-1.60677758290954));
#29091=CARTESIAN_POINT('Ctrl Pts',(1.32381550858256,-1.,-1.60073511858687));
#29092=CARTESIAN_POINT('Ctrl Pts',(1.32224985747682,-1.,-1.59471591079403));
#29093=CARTESIAN_POINT('Ctrl Pts',(1.32064537110892,-1.,-1.58872057258245));
#29094=CARTESIAN_POINT('Ctrl Pts',(1.31900135021432,-1.,-1.58274907898834));
#29095=CARTESIAN_POINT('Ctrl Pts',(1.31731642317187,-1.,-1.5768005650559));
#29096=CARTESIAN_POINT('Ctrl Pts',(1.31558903860016,-1.,-1.57087397835723));
#29097=CARTESIAN_POINT('Ctrl Pts',(1.31381795281002,-1.,-1.56496872402353));
#29098=CARTESIAN_POINT('Ctrl Pts',(1.31200264341696,-1.,-1.55908521254821));
#29099=CARTESIAN_POINT('Ctrl Pts',(1.31014393684222,-1.,-1.55322568759481));
#29100=CARTESIAN_POINT('Ctrl Pts',(1.30824393907473,-1.,-1.54739413957185));
#29101=CARTESIAN_POINT('Ctrl Pts',(1.30630475189556,-1.,-1.54159462645432));
#29102=CARTESIAN_POINT('Ctrl Pts',(1.30432735639489,-1.,-1.53582981268977));
#29103=CARTESIAN_POINT('Ctrl Pts',(1.30231064395568,-1.,-1.53009970283891));
#29104=CARTESIAN_POINT('Ctrl Pts',(1.30024984366328,-1.,-1.52439957861062));
#29105=CARTESIAN_POINT('Ctrl Pts',(1.29813791800747,-1.,-1.51872184912724));
#29106=CARTESIAN_POINT('Ctrl Pts',(1.29596850710509,-1.,-1.51305994241402));
#29107=CARTESIAN_POINT('Ctrl Pts',(1.29373841372842,-1.,-1.50741159078365));
#29108=CARTESIAN_POINT('Ctrl Pts',(1.29145022885181,-1.,-1.50178230149776));
#29109=CARTESIAN_POINT('Ctrl Pts',(1.28911506584254,-1.,-1.49618896881754));
#29110=CARTESIAN_POINT('Ctrl Pts',(1.2867467611644,-1.,-1.4906522831278));
#29111=CARTESIAN_POINT('Ctrl Pts',(1.28435533880201,-1.,-1.4851881711891));
#29112=CARTESIAN_POINT('Ctrl Pts',(1.28194158939517,-1.,-1.47980070347096));
#29113=CARTESIAN_POINT('Ctrl Pts',(1.2794891824849,-1.,-1.4744717526707));
#29114=CARTESIAN_POINT('Ctrl Pts',(1.27696414831089,-1.,-1.46916035917133));
#29115=CARTESIAN_POINT('Ctrl Pts',(1.27433119897822,-1.,-1.46382431332476));
#29116=CARTESIAN_POINT('Ctrl Pts',(1.27156805265289,-1.,-1.45843906294697));
#29117=CARTESIAN_POINT('Ctrl Pts',(1.2686778680489,-1.,-1.45301422764247));
#29118=CARTESIAN_POINT('Ctrl Pts',(1.26570925118868,-1.,-1.44761985001662));
#29119=CARTESIAN_POINT('Ctrl Pts',(1.26273903323858,-1.,-1.44236470511303));
#29120=CARTESIAN_POINT('Ctrl Pts',(1.25983531012005,-1.,-1.43734919180848));
#29121=CARTESIAN_POINT('Ctrl Pts',(1.25702687965755,-1.,-1.43262645609691));
#29122=CARTESIAN_POINT('Ctrl Pts',(1.25426945222639,-1.,-1.42815938799387));
#29123=CARTESIAN_POINT('Ctrl Pts',(1.2514145557001,-1.,-1.42378102115575));
#29124=CARTESIAN_POINT('Ctrl Pts',(1.24824430986571,-1.,-1.41923722596025));
#29125=CARTESIAN_POINT('Ctrl Pts',(1.24450600513056,-1.,-1.41422913175179));
#29126=CARTESIAN_POINT('Ctrl Pts',(1.23994455029534,-1.,-1.40845295531283));
#29127=CARTESIAN_POINT('Ctrl Pts',(1.23434087290423,-1.,-1.40164708206106));
#29128=CARTESIAN_POINT('Ctrl Pts',(1.22752961899387,-1.,-1.39361389568796));
#29129=CARTESIAN_POINT('Ctrl Pts',(1.21938737280852,-1.,-1.38420564527715));
#29130=CARTESIAN_POINT('Ctrl Pts',(1.20982812925645,-1.,-1.37331915607905));
#29131=CARTESIAN_POINT('Ctrl Pts',(1.1987959077932,-1.,-1.36088705043885));
#29132=CARTESIAN_POINT('Ctrl Pts',(1.18625865667441,-1.,-1.34687054001093));
#29133=CARTESIAN_POINT('Ctrl Pts',(1.17501305789857,-1.,-1.33437539347008));
#29134=CARTESIAN_POINT('Ctrl Pts',(1.16589330093588,-1.,-1.32428080721772));
#29135=CARTESIAN_POINT('Ctrl Pts',(1.15950888730809,-1.,-1.31722977216397));
#29136=CARTESIAN_POINT('Ctrl Pts',(1.15624053661742,-1.,-1.31362392696032));
#29137=CARTESIAN_POINT('',(1.31362392696032,-1.,-1.15624053661742));
#29138=CARTESIAN_POINT('Origin',(0.,-1.,0.));
#29139=CARTESIAN_POINT('',(1.73811241238545,-1.,-1.34869019493419));
#29140=CARTESIAN_POINT('Ctrl Pts',(1.31362392696032,-1.,-1.15624053661742));
#29141=CARTESIAN_POINT('Ctrl Pts',(1.3172297721596,-1.,-1.15950888730433));
#29142=CARTESIAN_POINT('Ctrl Pts',(1.32428080720544,-1.,-1.16589330092532));
#29143=CARTESIAN_POINT('Ctrl Pts',(1.33437539344842,-1.,-1.17501305787994));
#29144=CARTESIAN_POINT('Ctrl Pts',(1.34687053998157,-1.,-1.18625865664915));
#29145=CARTESIAN_POINT('Ctrl Pts',(1.36088705040677,-1.,-1.1987959077656));
#29146=CARTESIAN_POINT('Ctrl Pts',(1.37331915604962,-1.,-1.20982812923113));
#29147=CARTESIAN_POINT('Ctrl Pts',(1.38420564525391,-1.,-1.21938737278853));
#29148=CARTESIAN_POINT('Ctrl Pts',(1.39361389567257,-1.,-1.22752961898063));
#29149=CARTESIAN_POINT('Ctrl Pts',(1.40164708205345,-1.,-1.23434087289768));
#29150=CARTESIAN_POINT('Ctrl Pts',(1.40845295531151,-1.,-1.23994455029421));
#29151=CARTESIAN_POINT('Ctrl Pts',(1.41422913175437,-1.,-1.24450600513278));
#29152=CARTESIAN_POINT('Ctrl Pts',(1.41923722596421,-1.,-1.24824430986911));
#29153=CARTESIAN_POINT('Ctrl Pts',(1.42378102115911,-1.,-1.25141455570299));
#29154=CARTESIAN_POINT('Ctrl Pts',(1.42815938799555,-1.,-1.25426945222783));
#29155=CARTESIAN_POINT('Ctrl Pts',(1.43262645609679,-1.,-1.25702687965744));
#29156=CARTESIAN_POINT('Ctrl Pts',(1.43734919180719,-1.,-1.25983531011894));
#29157=CARTESIAN_POINT('Ctrl Pts',(1.44236470511145,-1.,-1.26273903323723));
#29158=CARTESIAN_POINT('Ctrl Pts',(1.44761985001544,-1.,-1.26570925118767));
#29159=CARTESIAN_POINT('Ctrl Pts',(1.45301422764205,-1.,-1.26867786804854));
#29160=CARTESIAN_POINT('Ctrl Pts',(1.45843906294725,-1.,-1.27156805265312));
#29161=CARTESIAN_POINT('Ctrl Pts',(1.4638243133254,-1.,-1.27433119897877));
#29162=CARTESIAN_POINT('Ctrl Pts',(1.46916035917197,-1.,-1.27696414831144));
#29163=CARTESIAN_POINT('Ctrl Pts',(1.4744717526711,-1.,-1.27948918248524));
#29164=CARTESIAN_POINT('Ctrl Pts',(1.47980070347102,-1.,-1.28194158939522));
#29165=CARTESIAN_POINT('Ctrl Pts',(1.48518817118891,-1.,-1.28435533880184));
#29166=CARTESIAN_POINT('Ctrl Pts',(1.4906522831275,-1.,-1.28674676116415));
#29167=CARTESIAN_POINT('Ctrl Pts',(1.49618896881729,-1.,-1.28911506584232));
#29168=CARTESIAN_POINT('Ctrl Pts',(1.50178230149764,-1.,-1.29145022885171));
#29169=CARTESIAN_POINT('Ctrl Pts',(1.50741159078367,-1.,-1.29373841372843));
#29170=CARTESIAN_POINT('Ctrl Pts',(1.51305994241412,-1.,-1.29596850710518));
#29171=CARTESIAN_POINT('Ctrl Pts',(1.51872184912735,-1.,-1.29813791800757));
#29172=CARTESIAN_POINT('Ctrl Pts',(1.5243995786107,-1.,-1.30024984366334));
#29173=CARTESIAN_POINT('Ctrl Pts',(1.53009970283893,-1.,-1.3023106439557));
#29174=CARTESIAN_POINT('Ctrl Pts',(1.53582981268976,-1.,-1.30432735639487));
#29175=CARTESIAN_POINT('Ctrl Pts',(1.54159462645428,-1.,-1.30630475189553));
#29176=CARTESIAN_POINT('Ctrl Pts',(1.54739413957183,-1.,-1.30824393907471));
#29177=CARTESIAN_POINT('Ctrl Pts',(1.55322568759481,-1.,-1.31014393684221));
#29178=CARTESIAN_POINT('Ctrl Pts',(1.55908521254822,-1.,-1.31200264341696));
#29179=CARTESIAN_POINT('Ctrl Pts',(1.56496872402352,-1.,-1.31381795281002));
#29180=CARTESIAN_POINT('Ctrl Pts',(1.57087397835721,-1.,-1.31558903860015));
#29181=CARTESIAN_POINT('Ctrl Pts',(1.57680056505585,-1.,-1.31731642317183));
#29182=CARTESIAN_POINT('Ctrl Pts',(1.58274907898829,-1.,-1.31900135021428));
#29183=CARTESIAN_POINT('Ctrl Pts',(1.58872057258244,-1.,-1.32064537110891));
#29184=CARTESIAN_POINT('Ctrl Pts',(1.59471591079408,-1.,-1.32224985747686));
#29185=CARTESIAN_POINT('Ctrl Pts',(1.600735118587,-1.,-1.32381550858266));
#29186=CARTESIAN_POINT('Ctrl Pts',(1.6067775829097,-1.,-1.32534250785794));
#29187=CARTESIAN_POINT('Ctrl Pts',(1.61284234015762,-1.,-1.32683074483365));
#29188=CARTESIAN_POINT('Ctrl Pts',(1.61892832270723,-1.,-1.32828000610448));
#29189=CARTESIAN_POINT('Ctrl Pts',(1.62503464209777,-1.,-1.32969019505665));
#29190=CARTESIAN_POINT('Ctrl Pts',(1.63116079730887,-1.,-1.33106149345618));
#29191=CARTESIAN_POINT('Ctrl Pts',(1.63730653475049,-1.,-1.33239425103694));
#29192=CARTESIAN_POINT('Ctrl Pts',(1.64347174856007,-1.,-1.33368890676554));
#29193=CARTESIAN_POINT('Ctrl Pts',(1.64965637286843,-1.,-1.33494590468003));
#29194=CARTESIAN_POINT('Ctrl Pts',(1.65586025952651,-1.,-1.33616559745217));
#29195=CARTESIAN_POINT('Ctrl Pts',(1.66208312542073,-1.,-1.33734820885331));
#29196=CARTESIAN_POINT('Ctrl Pts',(1.66832460784078,-1.,-1.33849388654458));
#29197=CARTESIAN_POINT('Ctrl Pts',(1.67458429426126,-1.,-1.33960273470372));
#29198=CARTESIAN_POINT('Ctrl Pts',(1.68086176030308,-1.,-1.3406748518516));
#29199=CARTESIAN_POINT('Ctrl Pts',(1.68715660868602,-1.,-1.34171037484673));
#29200=CARTESIAN_POINT('Ctrl Pts',(1.6934684849664,-1.,-1.34270948206139));
#29201=CARTESIAN_POINT('Ctrl Pts',(1.69979707754221,-1.,-1.34367237124322));
#29202=CARTESIAN_POINT('Ctrl Pts',(1.70614212266676,-1.,-1.34459924533783));
#29203=CARTESIAN_POINT('Ctrl Pts',(1.71250340687011,-1.,-1.34549029589563));
#29204=CARTESIAN_POINT('Ctrl Pts',(1.7188807715095,-1.,-1.34634568653586));
#29205=CARTESIAN_POINT('Ctrl Pts',(1.72527410681298,-1.,-1.34716554820013));
#29206=CARTESIAN_POINT('Ctrl Pts',(1.73040149654497,-1.,-1.3477930915247));
#29207=CARTESIAN_POINT('Ctrl Pts',(1.73425417886254,-1.,-1.34824783113158));
#29208=CARTESIAN_POINT('Ctrl Pts',(1.73682580585819,-1.,-1.34854391898145));
#29209=CARTESIAN_POINT('Ctrl Pts',(1.73811241238545,-1.,-1.34869019493419));
#29210=CARTESIAN_POINT('',(1.81978687191668,-1.,-1.23627494547115));
#29211=CARTESIAN_POINT('',(1.73811241238545,-1.,-1.34869019493419));
#29212=CARTESIAN_POINT('',(1.5055822144029,-1.,-0.892032620296855));
#29213=CARTESIAN_POINT('Ctrl Pts',(1.81978687191668,-1.,-1.23627494547115));
#29214=CARTESIAN_POINT('Ctrl Pts',(1.81925017193531,-1.,-1.23509651170384));
#29215=CARTESIAN_POINT('Ctrl Pts',(1.81817389920914,-1.,-1.23274224526804));
#29216=CARTESIAN_POINT('Ctrl Pts',(1.81655087183054,-1.,-1.22921864890975));
#29217=CARTESIAN_POINT('Ctrl Pts',(1.81436959209778,-1.,-1.22453613304507));
#29218=CARTESIAN_POINT('Ctrl Pts',(1.81161420806172,-1.,-1.2187090610323));
#29219=CARTESIAN_POINT('Ctrl Pts',(1.80882996916931,-1.,-1.2129081570818));
#29220=CARTESIAN_POINT('Ctrl Pts',(1.80601678480772,-1.,-1.20713356605519));
#29221=CARTESIAN_POINT('Ctrl Pts',(1.8031745483882,-1.,-1.2013854893912));
#29222=CARTESIAN_POINT('Ctrl Pts',(1.80030314370121,-1.,-1.19566418930405));
#29223=CARTESIAN_POINT('Ctrl Pts',(1.79740245923649,-1.,-1.1899699793456));
#29224=CARTESIAN_POINT('Ctrl Pts',(1.79447240321572,-1.,-1.18430321697471));
#29225=CARTESIAN_POINT('Ctrl Pts',(1.79151291552646,-1.,-1.17866429440781));
#29226=CARTESIAN_POINT('Ctrl Pts',(1.78852398877523,-1.,-1.17305363177265));
#29227=CARTESIAN_POINT('Ctrl Pts',(1.78550566040349,-1.,-1.16747166312239));
#29228=CARTESIAN_POINT('Ctrl Pts',(1.78245795880949,-1.,-1.16191881298458));
#29229=CARTESIAN_POINT('Ctrl Pts',(1.77938085564261,-1.,-1.15639547194689));
#29230=CARTESIAN_POINT('Ctrl Pts',(1.77627422557034,-1.,-1.15090197841531));
#29231=CARTESIAN_POINT('Ctrl Pts',(1.77313777896234,-1.,-1.14543858226948));
#29232=CARTESIAN_POINT('Ctrl Pts',(1.76997111386806,-1.,-1.14000548337));
#29233=CARTESIAN_POINT('Ctrl Pts',(1.76677384551883,-1.,-1.13460291804635));
#29234=CARTESIAN_POINT('Ctrl Pts',(1.76354571966171,-1.,-1.12923123555076));
#29235=CARTESIAN_POINT('Ctrl Pts',(1.76028671825084,-1.,-1.12389096855078));
#29236=CARTESIAN_POINT('Ctrl Pts',(1.75699720772089,-1.,-1.11858293216752));
#29237=CARTESIAN_POINT('Ctrl Pts',(1.75367772094617,-1.,-1.11330807582542));
#29238=CARTESIAN_POINT('Ctrl Pts',(1.75032866075914,-1.,-1.10806728183003));
#29239=CARTESIAN_POINT('Ctrl Pts',(1.74695004214924,-1.,-1.10286118991144));
#29240=CARTESIAN_POINT('Ctrl Pts',(1.74354119236212,-1.,-1.09768999241229));
#29241=CARTESIAN_POINT('Ctrl Pts',(1.74010053962252,-1.,-1.09255329056496));
#29242=CARTESIAN_POINT('Ctrl Pts',(1.73662628326093,-1.,-1.08745056285429));
#29243=CARTESIAN_POINT('Ctrl Pts',(1.73311705663407,-1.,-1.08238162784749));
#29244=CARTESIAN_POINT('Ctrl Pts',(1.72957248977424,-1.,-1.0773470373727));
#29245=CARTESIAN_POINT('Ctrl Pts',(1.72599406198489,-1.,-1.07234866990252));
#29246=CARTESIAN_POINT('Ctrl Pts',(1.72238500928456,-1.,-1.06738966975463));
#29247=CARTESIAN_POINT('Ctrl Pts',(1.71874858456908,-1.,-1.0624732468065));
#29248=CARTESIAN_POINT('Ctrl Pts',(1.71508654427022,-1.,-1.05760163192481));
#29249=CARTESIAN_POINT('Ctrl Pts',(1.71139783543986,-1.,-1.05277517202854));
#29250=CARTESIAN_POINT('Ctrl Pts',(1.70767646263641,-1.,-1.0479908540499));
#29251=CARTESIAN_POINT('Ctrl Pts',(1.70391338707969,-1.,-1.04324363334546));
#29252=CARTESIAN_POINT('Ctrl Pts',(1.70010052930951,-1.,-1.03852922490782));
#29253=CARTESIAN_POINT('Ctrl Pts',(1.69623414782769,-1.,-1.03384646003587));
#29254=CARTESIAN_POINT('Ctrl Pts',(1.69231840863471,-1.,-1.02919977579155));
#29255=CARTESIAN_POINT('Ctrl Pts',(1.68836910178475,-1.,-1.02460180535272));
#29256=CARTESIAN_POINT('Ctrl Pts',(1.68440578021739,-1.,-1.02006795074222));
#29257=CARTESIAN_POINT('Ctrl Pts',(1.6804428989482,-1.,-1.01561026162787));
#29258=CARTESIAN_POINT('Ctrl Pts',(1.67648246776457,-1.,-1.01123236493507));
#29259=CARTESIAN_POINT('Ctrl Pts',(1.67250335383248,-1.,-1.00692206696387));
#29260=CARTESIAN_POINT('Ctrl Pts',(1.66846059277231,-1.,-1.00265091003682));
#29261=CARTESIAN_POINT('Ctrl Pts',(1.66430758030304,-1.,-0.998389654952317));
#29262=CARTESIAN_POINT('Ctrl Pts',(1.66001553809916,-1.,-0.994121836661116));
#29263=CARTESIAN_POINT('Ctrl Pts',(1.65559044289746,-1.,-0.98985562785445));
#29264=CARTESIAN_POINT('Ctrl Pts',(1.6511001661277,-1.,-0.985642622921626));
#29265=CARTESIAN_POINT('Ctrl Pts',(1.64665139190834,-1.,-0.981562530940574));
#29266=CARTESIAN_POINT('Ctrl Pts',(1.64233990826831,-1.,-0.977689794120297));
#29267=CARTESIAN_POINT('Ctrl Pts',(1.63820952658157,-1.,-0.974066058287501));
#29268=CARTESIAN_POINT('Ctrl Pts',(1.63420665729609,-1.,-0.970669715996356));
#29269=CARTESIAN_POINT('Ctrl Pts',(1.63013849959083,-1.,-0.967387853228041));
#29270=CARTESIAN_POINT('Ctrl Pts',(1.6257193066974,-1.,-0.964046107037821));
#29271=CARTESIAN_POINT('Ctrl Pts',(1.62061638139929,-1.,-0.960438326099958));
#29272=CARTESIAN_POINT('Ctrl Pts',(1.61449324337233,-1.,-0.956354422921573));
#29273=CARTESIAN_POINT('Ctrl Pts',(1.60706069897794,-1.,-0.951613284361248));
#29274=CARTESIAN_POINT('Ctrl Pts',(1.59810042045408,-1.,-0.946078063325796));
#29275=CARTESIAN_POINT('Ctrl Pts',(1.58744937489796,-1.,-0.939646377909319));
#29276=CARTESIAN_POINT('Ctrl Pts',(1.57499388385561,-1.,-0.932246680128849));
#29277=CARTESIAN_POINT('Ctrl Pts',(1.56065988582509,-1.,-0.923832188966322));
#29278=CARTESIAN_POINT('Ctrl Pts',(1.54440491152807,-1.,-0.91437591904658));
#29279=CARTESIAN_POINT('Ctrl Pts',(1.52984849890434,-1.,-0.905967409640499));
#29280=CARTESIAN_POINT('Ctrl Pts',(1.51805569591479,-1.,-0.89918504749193));
#29281=CARTESIAN_POINT('Ctrl Pts',(1.50980486807181,-1.,-0.894452006967538));
#29282=CARTESIAN_POINT('Ctrl Pts',(1.5055822144029,-1.,-0.892032620296855));
#29283=CARTESIAN_POINT('',(1.60662857109684,-1.,-0.693717979106306));
#29284=CARTESIAN_POINT('Origin',(0.,-1.,0.));
#29285=CARTESIAN_POINT('',(2.0698113262342,-1.,-0.745574324794401));
#29286=CARTESIAN_POINT('Ctrl Pts',(1.60662857109684,-1.,-0.693717979106306));
#29287=CARTESIAN_POINT('Ctrl Pts',(1.61106790957619,-1.,-0.69571209787897));
#29288=CARTESIAN_POINT('Ctrl Pts',(1.61974673471117,-1.,-0.699605146398837));
#29289=CARTESIAN_POINT('Ctrl Pts',(1.6321654166204,-1.,-0.705159151977294));
#29290=CARTESIAN_POINT('Ctrl Pts',(1.64752408828442,-1.,-0.711993139340448));
#29291=CARTESIAN_POINT('Ctrl Pts',(1.66472880551777,-1.,-0.71958543378795));
#29292=CARTESIAN_POINT('Ctrl Pts',(1.67996158451922,-1.,-0.726235967982445));
#29293=CARTESIAN_POINT('Ctrl Pts',(1.69326921972915,-1.,-0.731963238685357));
#29294=CARTESIAN_POINT('Ctrl Pts',(1.70473309004249,-1.,-0.736799665716932));
#29295=CARTESIAN_POINT('Ctrl Pts',(1.71447789751001,-1.,-0.74079516202821));
#29296=CARTESIAN_POINT('Ctrl Pts',(1.72268229916769,-1.,-0.744021445433094));
#29297=CARTESIAN_POINT('Ctrl Pts',(1.72958533647714,-1.,-0.746574710097752));
#29298=CARTESIAN_POINT('Ctrl Pts',(1.7355035168033,-1.,-0.74858246295687));
#29299=CARTESIAN_POINT('Ctrl Pts',(1.74080458267114,-1.,-0.75019343598125));
#29300=CARTESIAN_POINT('Ctrl Pts',(1.74585086852502,-1.,-0.751555614164483));
#29301=CARTESIAN_POINT('Ctrl Pts',(1.75095139468794,-1.,-0.752797683531314));
#29302=CARTESIAN_POINT('Ctrl Pts',(1.75631083600019,-1.,-0.754009254027829));
#29303=CARTESIAN_POINT('Ctrl Pts',(1.76197817240128,-1.,-0.755220979974462));
#29304=CARTESIAN_POINT('Ctrl Pts',(1.76789396002998,-1.,-0.75642189602781));
#29305=CARTESIAN_POINT('Ctrl Pts',(1.77394167108292,-1.,-0.757578264077029));
#29306=CARTESIAN_POINT('Ctrl Pts',(1.77999411220945,-1.,-0.758650626677519));
#29307=CARTESIAN_POINT('Ctrl Pts',(1.78596964884604,-1.,-0.75961440111019));
#29308=CARTESIAN_POINT('Ctrl Pts',(1.7918581561088,-1.,-0.760469555880749));
#29309=CARTESIAN_POINT('Ctrl Pts',(1.79768986997783,-1.,-0.761229695230558));
#29310=CARTESIAN_POINT('Ctrl Pts',(1.80351583877342,-1.,-0.761915336443547));
#29311=CARTESIAN_POINT('Ctrl Pts',(1.80938551463965,-1.,-0.762546129463938));
#29312=CARTESIAN_POINT('Ctrl Pts',(1.8153211840553,-1.,-0.763132003836634));
#29313=CARTESIAN_POINT('Ctrl Pts',(1.82131873145266,-1.,-0.763673465462727));
#29314=CARTESIAN_POINT('Ctrl Pts',(1.82735991200065,-1.,-0.764165902605995));
#29315=CARTESIAN_POINT('Ctrl Pts',(1.83342077227142,-1.,-0.764602549687853));
#29316=CARTESIAN_POINT('Ctrl Pts',(1.83948181064835,-1.,-0.764978057881738));
#29317=CARTESIAN_POINT('Ctrl Pts',(1.84553698875924,-1.,-0.765291664862029));
#29318=CARTESIAN_POINT('Ctrl Pts',(1.85158945130063,-1.,-0.765545710619063));
#29319=CARTESIAN_POINT('Ctrl Pts',(1.85764741390394,-1.,-0.765744212909319));
#29320=CARTESIAN_POINT('Ctrl Pts',(1.86372027063312,-1.,-0.765891519092547));
#29321=CARTESIAN_POINT('Ctrl Pts',(1.86981398314341,-1.,-0.765990708546091));
#29322=CARTESIAN_POINT('Ctrl Pts',(1.87592888967883,-1.,-0.766042837036744));
#29323=CARTESIAN_POINT('Ctrl Pts',(1.88206215302561,-1.,-0.766047794851865));
#29324=CARTESIAN_POINT('Ctrl Pts',(1.88820926433409,-1.,-0.766004837062091));
#29325=CARTESIAN_POINT('Ctrl Pts',(1.89436577771388,-1.,-0.765913193856978));
#29326=CARTESIAN_POINT('Ctrl Pts',(1.90052930393596,-1.,-0.765772772593386));
#29327=CARTESIAN_POINT('Ctrl Pts',(1.90669961402356,-1.,-0.765584196937919));
#29328=CARTESIAN_POINT('Ctrl Pts',(1.91287765805169,-1.,-0.765348465884722));
#29329=CARTESIAN_POINT('Ctrl Pts',(1.91906491634196,-1.,-0.765066729667089));
#29330=CARTESIAN_POINT('Ctrl Pts',(1.92526263537048,-1.,-0.764740025488212));
#29331=CARTESIAN_POINT('Ctrl Pts',(1.93147105496382,-1.,-0.764369010673941));
#29332=CARTESIAN_POINT('Ctrl Pts',(1.93768964875886,-1.,-0.763954049121459));
#29333=CARTESIAN_POINT('Ctrl Pts',(1.9439174661764,-1.,-0.763495333538629));
#29334=CARTESIAN_POINT('Ctrl Pts',(1.95015342590024,-1.,-0.762992990878769));
#29335=CARTESIAN_POINT('Ctrl Pts',(1.95639665309869,-1.,-0.762447203806179));
#29336=CARTESIAN_POINT('Ctrl Pts',(1.96264672744186,-1.,-0.761858300014424));
#29337=CARTESIAN_POINT('Ctrl Pts',(1.96890351582499,-1.,-0.761226690483821));
#29338=CARTESIAN_POINT('Ctrl Pts',(1.97516705321494,-1.,-0.760552825409757));
#29339=CARTESIAN_POINT('Ctrl Pts',(1.98143741418172,-1.,-0.75983714745219));
#29340=CARTESIAN_POINT('Ctrl Pts',(1.98771456680874,-1.,-0.759080037802488));
#29341=CARTESIAN_POINT('Ctrl Pts',(1.99399831098817,-1.,-0.758281796766761));
#29342=CARTESIAN_POINT('Ctrl Pts',(2.00028834739178,-1.,-0.757442676862724));
#29343=CARTESIAN_POINT('Ctrl Pts',(2.0065843158773,-1.,-0.756562904646671));
#29344=CARTESIAN_POINT('Ctrl Pts',(2.01288584328084,-1.,-0.755642704957865));
#29345=CARTESIAN_POINT('Ctrl Pts',(2.01919259405809,-1.,-0.754682330722816));
#29346=CARTESIAN_POINT('Ctrl Pts',(2.02550428623313,-1.,-0.753682061112768));
#29347=CARTESIAN_POINT('Ctrl Pts',(2.03182068456221,-1.,-0.752642180487211));
#29348=CARTESIAN_POINT('Ctrl Pts',(2.03814160092099,-1.,-0.751562963361115));
#29349=CARTESIAN_POINT('Ctrl Pts',(2.04446689147979,-1.,-0.750444657875576));
#29350=CARTESIAN_POINT('Ctrl Pts',(2.05079645592154,-1.,-0.749287468665046));
#29351=CARTESIAN_POINT('Ctrl Pts',(2.05713023031006,-1.,-0.748091554183803));
#29352=CARTESIAN_POINT('Ctrl Pts',(2.06220058927826,-1.,-0.74710393278792));
#29353=CARTESIAN_POINT('Ctrl Pts',(2.06600523016815,-1.,-0.746345871544201));
#29354=CARTESIAN_POINT('Ctrl Pts',(2.06854248895728,-1.,-0.745832791378367));
#29355=CARTESIAN_POINT('Ctrl Pts',(2.0698113262342,-1.,-0.745574324794401));
#29356=CARTESIAN_POINT('',(2.11275013067528,-1.,-0.61342227326009));
#29357=CARTESIAN_POINT('',(2.0698113262342,-1.,-0.745574324794401));
#29358=CARTESIAN_POINT('',(1.7075470150345,-1.,-0.383122945602004));
#29359=CARTESIAN_POINT('Ctrl Pts',(2.11275013067528,-1.,-0.61342227326009));
#29360=CARTESIAN_POINT('Ctrl Pts',(2.11187554259986,-1.,-0.6124673655618));
#29361=CARTESIAN_POINT('Ctrl Pts',(2.11012443807238,-1.,-0.610560911689899));
#29362=CARTESIAN_POINT('Ctrl Pts',(2.1074919961518,-1.,-0.607711315454876));
#29363=CARTESIAN_POINT('Ctrl Pts',(2.10397049886949,-1.,-0.60393203073603));
#29364=CARTESIAN_POINT('Ctrl Pts',(2.0995493086477,-1.,-0.599241616420534));
#29365=CARTESIAN_POINT('Ctrl Pts',(2.0951087622027,-1.,-0.594585006052162));
#29366=CARTESIAN_POINT('Ctrl Pts',(2.09064881812129,-1.,-0.589962365403406));
#29367=CARTESIAN_POINT('Ctrl Pts',(2.08616943727951,-1.,-0.585373918991617));
#29368=CARTESIAN_POINT('Ctrl Pts',(2.08167059018418,-1.,-0.580819952108064));
#29369=CARTESIAN_POINT('Ctrl Pts',(2.07715226767559,-1.,-0.576300797416845));
#29370=CARTESIAN_POINT('Ctrl Pts',(2.07261449292824,-1.,-0.571816823242603));
#29371=CARTESIAN_POINT('Ctrl Pts',(2.06805732997334,-1.,-0.567368421181087));
#29372=CARTESIAN_POINT('Ctrl Pts',(2.06348090160589,-1.,-0.562955993082262));
#29373=CARTESIAN_POINT('Ctrl Pts',(2.05888537756462,-1.,-0.558579940185152));
#29374=CARTESIAN_POINT('Ctrl Pts',(2.05427091604413,-1.,-0.554240657463906));
#29375=CARTESIAN_POINT('Ctrl Pts',(2.04963761077958,-1.,-0.549938525150295));
#29376=CARTESIAN_POINT('Ctrl Pts',(2.04498544714588,-1.,-0.54567390381743));
#29377=CARTESIAN_POINT('Ctrl Pts',(2.04031422690527,-1.,-0.541447120615659));
#29378=CARTESIAN_POINT('Ctrl Pts',(2.03562362954037,-1.,-0.537258489833262));
#29379=CARTESIAN_POINT('Ctrl Pts',(2.03091336214426,-1.,-0.533108355132977));
#29380=CARTESIAN_POINT('Ctrl Pts',(2.0261832908329,-1.,-0.528997127241914));
#29381=CARTESIAN_POINT('Ctrl Pts',(2.02143356304698,-1.,-0.524925318333476));
#29382=CARTESIAN_POINT('Ctrl Pts',(2.01666477917286,-1.,-0.520893590399371));
#29383=CARTESIAN_POINT('Ctrl Pts',(2.01187773939242,-1.,-0.516902681728687));
#29384=CARTESIAN_POINT('Ctrl Pts',(2.00707309946949,-1.,-0.512953306961793));
#29385=CARTESIAN_POINT('Ctrl Pts',(2.00225107134734,-1.,-0.509046069886157));
#29386=CARTESIAN_POINT('Ctrl Pts',(1.99741107463572,-1.,-0.505181361323026));
#29387=CARTESIAN_POINT('Ctrl Pts',(1.99255149126155,-1.,-0.501359287727146));
#29388=CARTESIAN_POINT('Ctrl Pts',(1.98767044752932,-1.,-0.497579909545574));
#29389=CARTESIAN_POINT('Ctrl Pts',(1.98276658761821,-1.,-0.493843476541495));
#29390=CARTESIAN_POINT('Ctrl Pts',(1.97783973019229,-1.,-0.490150627860953));
#29391=CARTESIAN_POINT('Ctrl Pts',(1.97289186263272,-1.,-0.486502692907659));
#29392=CARTESIAN_POINT('Ctrl Pts',(1.96792703422362,-1.,-0.482901662120691));
#29393=CARTESIAN_POINT('Ctrl Pts',(1.96294933055943,-1.,-0.479349583074855));
#29394=CARTESIAN_POINT('Ctrl Pts',(1.95796111148177,-1.,-0.475848034683176));
#29395=CARTESIAN_POINT('Ctrl Pts',(1.95296148278133,-1.,-0.472397672264072));
#29396=CARTESIAN_POINT('Ctrl Pts',(1.94794381136514,-1.,-0.468997482913135));
#29397=CARTESIAN_POINT('Ctrl Pts',(1.9428979419619,-1.,-0.46564546202603));
#29398=CARTESIAN_POINT('Ctrl Pts',(1.93781486640821,-1.,-0.462340031009057));
#29399=CARTESIAN_POINT('Ctrl Pts',(1.93269066517934,-1.,-0.459081234547926));
#29400=CARTESIAN_POINT('Ctrl Pts',(1.92753067150476,-1.,-0.455872005174371));
#29401=CARTESIAN_POINT('Ctrl Pts',(1.92235380648502,-1.,-0.452719478359433));
#29402=CARTESIAN_POINT('Ctrl Pts',(1.91718342555755,-1.,-0.449632260106662));
#29403=CARTESIAN_POINT('Ctrl Pts',(1.9120369998112,-1.,-0.446617343485711));
#29404=CARTESIAN_POINT('Ctrl Pts',(1.90691756144898,-1.,-0.443677556849151));
#29405=CARTESIAN_POINT('Ctrl Pts',(1.90180124389086,-1.,-0.440807833704038));
#29406=CARTESIAN_POINT('Ctrl Pts',(1.89663648956466,-1.,-0.437995003948244));
#29407=CARTESIAN_POINT('Ctrl Pts',(1.89136993975504,-1.,-0.435225660963383));
#29408=CARTESIAN_POINT('Ctrl Pts',(1.88596913666793,-1.,-0.432493038548748));
#29409=CARTESIAN_POINT('Ctrl Pts',(1.88044229001832,-1.,-0.429803062482345));
#29410=CARTESIAN_POINT('Ctrl Pts',(1.87486989291484,-1.,-0.427183828519102));
#29411=CARTESIAN_POINT('Ctrl Pts',(1.86937803944323,-1.,-0.424678177291359));
#29412=CARTESIAN_POINT('Ctrl Pts',(1.86408083334028,-1.,-0.422327307418275));
#29413=CARTESIAN_POINT('Ctrl Pts',(1.85903281096686,-1.,-0.42015728797562));
#29414=CARTESIAN_POINT('Ctrl Pts',(1.85417632856234,-1.,-0.418164129143534));
#29415=CARTESIAN_POINT('Ctrl Pts',(1.84929312929882,-1.,-0.416300022038864));
#29416=CARTESIAN_POINT('Ctrl Pts',(1.8440575707371,-1.,-0.41448743825434));
#29417=CARTESIAN_POINT('Ctrl Pts',(1.83808953475839,-1.,-0.412633125322162));
#29418=CARTESIAN_POINT('Ctrl Pts',(1.83100408895216,-1.,-0.410641256301675));
#29419=CARTESIAN_POINT('Ctrl Pts',(1.8224702267854,-1.,-0.408428948108534));
#29420=CARTESIAN_POINT('Ctrl Pts',(1.81223801813988,-1.,-0.405933518411838));
#29421=CARTESIAN_POINT('Ctrl Pts',(1.80012077176221,-1.,-0.403107976170441));
#29422=CARTESIAN_POINT('Ctrl Pts',(1.78598826347533,-1.,-0.399919403783081));
#29423=CARTESIAN_POINT('Ctrl Pts',(1.7697556004756,-1.,-0.39634619612042));
#29424=CARTESIAN_POINT('Ctrl Pts',(1.75137405313962,-1.,-0.392375812294307));
#29425=CARTESIAN_POINT('Ctrl Pts',(1.7349317097561,-1.,-0.388877023509192));
#29426=CARTESIAN_POINT('Ctrl Pts',(1.72162022246158,-1.,-0.38607079032701));
#29427=CARTESIAN_POINT('Ctrl Pts',(1.71231062891958,-1.,-0.384119047315542));
#29428=CARTESIAN_POINT('Ctrl Pts',(1.7075470150345,-1.,-0.383122945602004));
#29429=CARTESIAN_POINT('',(1.74236521665491,-1.,-0.163289472382896));
#29430=CARTESIAN_POINT('Origin',(0.,-1.,0.));
#29431=CARTESIAN_POINT('',(2.19890268624765,-1.,-0.0694764450219582));
#29432=CARTESIAN_POINT('Ctrl Pts',(1.74236521665491,-1.,-0.163289472382896));
#29433=CARTESIAN_POINT('Ctrl Pts',(1.7472034950333,-1.,-0.163814161002002));
#29434=CARTESIAN_POINT('Ctrl Pts',(1.75666056638427,-1.,-0.164834765707159));
#29435=CARTESIAN_POINT('Ctrl Pts',(1.77018771684844,-1.,-0.1662793551464));
#29436=CARTESIAN_POINT('Ctrl Pts',(1.7869064998507,-1.,-0.168032772805197));
#29437=CARTESIAN_POINT('Ctrl Pts',(1.80561530629706,-1.,-0.169936923904608));
#29438=CARTESIAN_POINT('Ctrl Pts',(1.82215766811545,-1.,-0.171554770204119));
#29439=CARTESIAN_POINT('Ctrl Pts',(1.83658380527692,-1.,-0.1728894428919));
#29440=CARTESIAN_POINT('Ctrl Pts',(1.8489811319852,-1.,-0.173946627587732));
#29441=CARTESIAN_POINT('Ctrl Pts',(1.85948367088837,-1.,-0.17473525927603));
#29442=CARTESIAN_POINT('Ctrl Pts',(1.86828349694799,-1.,-0.175268337590758));
#29443=CARTESIAN_POINT('Ctrl Pts',(1.87563767773588,-1.,-0.175563480746485));
#29444=CARTESIAN_POINT('Ctrl Pts',(1.88188663145367,-1.,-0.175644148889699));
#29445=CARTESIAN_POINT('Ctrl Pts',(1.88742606273259,-1.,-0.175538155840648));
#29446=CARTESIAN_POINT('Ctrl Pts',(1.892646301985,-1.,-0.175274276190844));
#29447=CARTESIAN_POINT('Ctrl Pts',(1.89788101117132,-1.,-0.174879405091263));
#29448=CARTESIAN_POINT('Ctrl Pts',(1.90335253862834,-1.,-0.174375518661085));
#29449=CARTESIAN_POINT('Ctrl Pts',(1.90911693975267,-1.,-0.173776635257817));
#29450=CARTESIAN_POINT('Ctrl Pts',(1.91511429159527,-1.,-0.173090695383496));
#29451=CARTESIAN_POINT('Ctrl Pts',(1.9212233439798,-1.,-0.172321621259514));
#29452=CARTESIAN_POINT('Ctrl Pts',(1.92731093582036,-1.,-0.171471191532988));
#29453=CARTESIAN_POINT('Ctrl Pts',(1.93329183155539,-1.,-0.170541253116202));
#29454=CARTESIAN_POINT('Ctrl Pts',(1.93915639211581,-1.,-0.169534904817491));
#29455=CARTESIAN_POINT('Ctrl Pts',(1.94493757756931,-1.,-0.168455741607556));
#29456=CARTESIAN_POINT('Ctrl Pts',(1.95069027794294,-1.,-0.167307501784476));
#29457=CARTESIAN_POINT('Ctrl Pts',(1.9564675971873,-1.,-0.166093592002813));
#29458=CARTESIAN_POINT('Ctrl Pts',(1.96229379940136,-1.,-0.164816568920269));
#29459=CARTESIAN_POINT('Ctrl Pts',(1.96816512677967,-1.,-0.163478185457734));
#29460=CARTESIAN_POINT('Ctrl Pts',(1.97406280235188,-1.,-0.162079693556289));
#29461=CARTESIAN_POINT('Ctrl Pts',(1.97996195437559,-1.,-0.160622060784611));
#29462=CARTESIAN_POINT('Ctrl Pts',(1.98584238283292,-1.,-0.159106226437299));
#29463=CARTESIAN_POINT('Ctrl Pts',(1.99169810931908,-1.,-0.157533331459227));
#29464=CARTESIAN_POINT('Ctrl Pts',(1.99753284771497,-1.,-0.155904629548784));
#29465=CARTESIAN_POINT('Ctrl Pts',(2.00335565310543,-1.,-0.154221403049722));
#29466=CARTESIAN_POINT('Ctrl Pts',(2.00917680318424,-1.,-0.15248488362145));
#29467=CARTESIAN_POINT('Ctrl Pts',(2.01500291940238,-1.,-0.150696157673078));
#29468=CARTESIAN_POINT('Ctrl Pts',(2.02083464969894,-1.,-0.148856124775337));
#29469=CARTESIAN_POINT('Ctrl Pts',(2.02666926182017,-1.,-0.146965557332583));
#29470=CARTESIAN_POINT('Ctrl Pts',(2.03250223739942,-1.,-0.145025140186058));
#29471=CARTESIAN_POINT('Ctrl Pts',(2.03832911025912,-1.,-0.143035515058209));
#29472=CARTESIAN_POINT('Ctrl Pts',(2.04414757947916,-1.,-0.140997332152546));
#29473=CARTESIAN_POINT('Ctrl Pts',(2.04995762001328,-1.,-0.138911255368966));
#29474=CARTESIAN_POINT('Ctrl Pts',(2.05576044414264,-1.,-0.136777941218044));
#29475=CARTESIAN_POINT('Ctrl Pts',(2.06155781517842,-1.,-0.134598026192106));
#29476=CARTESIAN_POINT('Ctrl Pts',(2.06735123910326,-1.,-0.132372111547711));
#29477=CARTESIAN_POINT('Ctrl Pts',(2.07314114713063,-1.,-0.130100748328404));
#29478=CARTESIAN_POINT('Ctrl Pts',(2.07892715110987,-1.,-0.12778444527612));
#29479=CARTESIAN_POINT('Ctrl Pts',(2.08470840653643,-1.,-0.125423679412062));
#29480=CARTESIAN_POINT('Ctrl Pts',(2.09048392424825,-1.,-0.123018905621083));
#29481=CARTESIAN_POINT('Ctrl Pts',(2.0962529286773,-1.,-0.120570567965122));
#29482=CARTESIAN_POINT('Ctrl Pts',(2.102015121329,-1.,-0.118079107988356));
#29483=CARTESIAN_POINT('Ctrl Pts',(2.10777050261309,-1.,-0.115544957687927));
#29484=CARTESIAN_POINT('Ctrl Pts',(2.11351924490306,-1.,-0.112968534419737));
#29485=CARTESIAN_POINT('Ctrl Pts',(2.11926155590865,-1.,-0.110350236135025));
#29486=CARTESIAN_POINT('Ctrl Pts',(2.12499752307,-1.,-0.10769043523109));
#29487=CARTESIAN_POINT('Ctrl Pts',(2.13072704887293,-1.,-0.10498947915274));
#29488=CARTESIAN_POINT('Ctrl Pts',(2.13644992667165,-1.,-0.102247700556101));
#29489=CARTESIAN_POINT('Ctrl Pts',(2.14216588396025,-1.,-0.0994654261990917));
#29490=CARTESIAN_POINT('Ctrl Pts',(2.14787463531795,-1.,-0.096642985230546));
#29491=CARTESIAN_POINT('Ctrl Pts',(2.1535759397817,-1.,-0.0937807218867645));
#29492=CARTESIAN_POINT('Ctrl Pts',(2.15926961544516,-1.,-0.0908789888107267));
#29493=CARTESIAN_POINT('Ctrl Pts',(2.16495552645014,-1.,-0.0879381291386924));
#29494=CARTESIAN_POINT('Ctrl Pts',(2.17063357870952,-1.,-0.0849584620835374));
#29495=CARTESIAN_POINT('Ctrl Pts',(2.176303712113,-1.,-0.0819402680872767));
#29496=CARTESIAN_POINT('Ctrl Pts',(2.18196589448887,-1.,-0.0788837727685244));
#29497=CARTESIAN_POINT('Ctrl Pts',(2.1876201139953,-1.,-0.0757891465836149));
#29498=CARTESIAN_POINT('Ctrl Pts',(2.19213712013662,-1.,-0.0732830357306726));
#29499=CARTESIAN_POINT('Ctrl Pts',(2.19552129484002,-1.,-0.0713863779526155));
#29500=CARTESIAN_POINT('Ctrl Pts',(2.19777582085423,-1.,-0.0701143536325491));
#29501=CARTESIAN_POINT('Ctrl Pts',(2.19890268624765,-1.,-0.0694764450219582));
#29502=CARTESIAN_POINT('',(2.19890268624765,-1.,0.0694764450219582));
#29503=CARTESIAN_POINT('',(2.19890268624765,-1.,-0.0694764450219582));
#29504=CARTESIAN_POINT('',(1.74236521665491,-1.,0.163289472382896));
#29505=CARTESIAN_POINT('Ctrl Pts',(2.19890268624765,-1.,0.0694764450219582));
#29506=CARTESIAN_POINT('Ctrl Pts',(2.19777582085261,-1.,0.0701143536324925));
#29507=CARTESIAN_POINT('Ctrl Pts',(2.19552129483562,-1.,0.0713863779524626));
#29508=CARTESIAN_POINT('Ctrl Pts',(2.19213712012956,-1.,0.0732830357304275));
#29509=CARTESIAN_POINT('Ctrl Pts',(2.1876201139874,-1.,0.075789146583341));
#29510=CARTESIAN_POINT('Ctrl Pts',(2.18196589448304,-1.,0.0788837727683226));
#29511=CARTESIAN_POINT('Ctrl Pts',(2.1763037121106,-1.,0.0819402680871938));
#29512=CARTESIAN_POINT('Ctrl Pts',(2.17063357871031,-1.,0.0849584620835642));
#29513=CARTESIAN_POINT('Ctrl Pts',(2.16495552645275,-1.,0.0879381291387821));
#29514=CARTESIAN_POINT('Ctrl Pts',(2.15926961544808,-1.,0.0908789888108265));
#29515=CARTESIAN_POINT('Ctrl Pts',(2.15357593978377,-1.,0.0937807218868344));
#29516=CARTESIAN_POINT('Ctrl Pts',(2.14787463531864,-1.,0.0966429852305688));
#29517=CARTESIAN_POINT('Ctrl Pts',(2.14216588395974,-1.,0.0994654261990741));
#29518=CARTESIAN_POINT('Ctrl Pts',(2.13644992667052,-1.,0.102247700556063));
#29519=CARTESIAN_POINT('Ctrl Pts',(2.1307270488718,-1.,0.104989479152703));
#29520=CARTESIAN_POINT('Ctrl Pts',(2.12499752306927,-1.,0.107690435231068));
#29521=CARTESIAN_POINT('Ctrl Pts',(2.11926155590849,-1.,0.11035023613502));
#29522=CARTESIAN_POINT('Ctrl Pts',(2.11351924490335,-1.,0.112968534419746));
#29523=CARTESIAN_POINT('Ctrl Pts',(2.10777050261359,-1.,0.11554495768794));
#29524=CARTESIAN_POINT('Ctrl Pts',(2.10201512132945,-1.,0.118079107988368));
#29525=CARTESIAN_POINT('Ctrl Pts',(2.09625292867756,-1.,0.120570567965129));
#29526=CARTESIAN_POINT('Ctrl Pts',(2.09048392424826,-1.,0.123018905621083));
#29527=CARTESIAN_POINT('Ctrl Pts',(2.08470840653628,-1.,0.125423679412058));
#29528=CARTESIAN_POINT('Ctrl Pts',(2.07892715110967,-1.,0.127784445276116));
#29529=CARTESIAN_POINT('Ctrl Pts',(2.07314114713047,-1.,0.1301007483284));
#29530=CARTESIAN_POINT('Ctrl Pts',(2.06735123910319,-1.,0.132372111547709));
#29531=CARTESIAN_POINT('Ctrl Pts',(2.06155781517844,-1.,0.134598026192107));
#29532=CARTESIAN_POINT('Ctrl Pts',(2.0557604441427,-1.,0.136777941218044));
#29533=CARTESIAN_POINT('Ctrl Pts',(2.04995762001333,-1.,0.138911255368966));
#29534=CARTESIAN_POINT('Ctrl Pts',(2.04414757947919,-1.,0.140997332152545));
#29535=CARTESIAN_POINT('Ctrl Pts',(2.03832911025913,-1.,0.143035515058208));
#29536=CARTESIAN_POINT('Ctrl Pts',(2.03250223739941,-1.,0.145025140186058));
#29537=CARTESIAN_POINT('Ctrl Pts',(2.02666926182017,-1.,0.146965557332586));
#29538=CARTESIAN_POINT('Ctrl Pts',(2.02083464969897,-1.,0.148856124775342));
#29539=CARTESIAN_POINT('Ctrl Pts',(2.01500291940243,-1.,0.150696157673084));
#29540=CARTESIAN_POINT('Ctrl Pts',(2.00917680318426,-1.,0.152484883621452));
#29541=CARTESIAN_POINT('Ctrl Pts',(2.00335565310539,-1.,0.154221403049719));
#29542=CARTESIAN_POINT('Ctrl Pts',(1.99753284771487,-1.,0.155904629548774));
#29543=CARTESIAN_POINT('Ctrl Pts',(1.99169810931893,-1.,0.157533331459215));
#29544=CARTESIAN_POINT('Ctrl Pts',(1.98584238283279,-1.,0.159106226437288));
#29545=CARTESIAN_POINT('Ctrl Pts',(1.97996195437557,-1.,0.16062206078461));
#29546=CARTESIAN_POINT('Ctrl Pts',(1.97406280235204,-1.,0.162079693556302));
#29547=CARTESIAN_POINT('Ctrl Pts',(1.96816512678,-1.,0.16347818545776));
#29548=CARTESIAN_POINT('Ctrl Pts',(1.96229379940174,-1.,0.1648165689203));
#29549=CARTESIAN_POINT('Ctrl Pts',(1.95646759718755,-1.,0.166093592002832));
#29550=CARTESIAN_POINT('Ctrl Pts',(1.95069027794286,-1.,0.167307501784469));
#29551=CARTESIAN_POINT('Ctrl Pts',(1.94493757756879,-1.,0.168455741607515));
#29552=CARTESIAN_POINT('Ctrl Pts',(1.93915639211497,-1.,0.169534904817425));
#29553=CARTESIAN_POINT('Ctrl Pts',(1.93329183155455,-1.,0.170541253116136));
#29554=CARTESIAN_POINT('Ctrl Pts',(1.92731093582,-1.,0.17147119153296));
#29555=CARTESIAN_POINT('Ctrl Pts',(1.92122334398034,-1.,0.172321621259556));
#29556=CARTESIAN_POINT('Ctrl Pts',(1.91511429159681,-1.,0.173090695383619));
#29557=CARTESIAN_POINT('Ctrl Pts',(1.90911693975475,-1.,0.173776635257983));
#29558=CARTESIAN_POINT('Ctrl Pts',(1.90335253863003,-1.,0.174375518661222));
#29559=CARTESIAN_POINT('Ctrl Pts',(1.89788101117148,-1.,0.174879405091277));
#29560=CARTESIAN_POINT('Ctrl Pts',(1.89264630198279,-1.,0.175274276190664));
#29561=CARTESIAN_POINT('Ctrl Pts',(1.88742606272818,-1.,0.175538155840286));
#29562=CARTESIAN_POINT('Ctrl Pts',(1.88188663144846,-1.,0.175644148889271));
#29563=CARTESIAN_POINT('Ctrl Pts',(1.87563767773249,-1.,0.175563480746205));
#29564=CARTESIAN_POINT('Ctrl Pts',(1.86828349694972,-1.,0.1752683375909));
#29565=CARTESIAN_POINT('Ctrl Pts',(1.85948367089838,-1.,0.174735259276856));
#29566=CARTESIAN_POINT('Ctrl Pts',(1.84898113200543,-1.,0.173946627589401));
#29567=CARTESIAN_POINT('Ctrl Pts',(1.83658380530747,-1.,0.17288944289442));
#29568=CARTESIAN_POINT('Ctrl Pts',(1.82215766815414,-1.,0.171554770207306));
#29569=CARTESIAN_POINT('Ctrl Pts',(1.80561530633924,-1.,0.169936923908078));
#29570=CARTESIAN_POINT('Ctrl Pts',(1.78690649988931,-1.,0.16803277280837));
#29571=CARTESIAN_POINT('Ctrl Pts',(1.77018771687692,-1.,0.166279355148738));
#29572=CARTESIAN_POINT('Ctrl Pts',(1.75666056640041,-1.,0.164834765708484));
#29573=CARTESIAN_POINT('Ctrl Pts',(1.74720349503904,-1.,0.163814161002474));
#29574=CARTESIAN_POINT('Ctrl Pts',(1.74236521665491,-1.,0.163289472382896));
#29575=CARTESIAN_POINT('',(1.7075470150345,-1.,0.383122945602004));
#29576=CARTESIAN_POINT('Origin',(0.,-1.,0.));
#29577=CARTESIAN_POINT('',(2.11275013067528,-1.,0.613422273260091));
#29578=CARTESIAN_POINT('Ctrl Pts',(1.7075470150345,-1.,0.383122945602004));
#29579=CARTESIAN_POINT('Ctrl Pts',(1.71231062891398,-1.,0.384119047314215));
#29580=CARTESIAN_POINT('Ctrl Pts',(1.72162022244582,-1.,0.386070790323281));
#29581=CARTESIAN_POINT('Ctrl Pts',(1.73493170972829,-1.,0.388877023502615));
#29582=CARTESIAN_POINT('Ctrl Pts',(1.75137405310193,-1.,0.392375812285396));
#29583=CARTESIAN_POINT('Ctrl Pts',(1.76975560043442,-1.,0.396346196110688));
#29584=CARTESIAN_POINT('Ctrl Pts',(1.78598826343754,-1.,0.399919403774156));
#29585=CARTESIAN_POINT('Ctrl Pts',(1.80012077173238,-1.,0.403107976163396));
#29586=CARTESIAN_POINT('Ctrl Pts',(1.81223801812013,-1.,0.405933518407176));
#29587=CARTESIAN_POINT('Ctrl Pts',(1.82247022677562,-1.,0.408428948106228));
#29588=CARTESIAN_POINT('Ctrl Pts',(1.83100408895047,-1.,0.410641256301276));
#29589=CARTESIAN_POINT('Ctrl Pts',(1.8380895347617,-1.,0.412633125322945));
#29590=CARTESIAN_POINT('Ctrl Pts',(1.84405757074218,-1.,0.414487438255542));
#29591=CARTESIAN_POINT('Ctrl Pts',(1.84929312930314,-1.,0.416300022039885));
#29592=CARTESIAN_POINT('Ctrl Pts',(1.8541763285645,-1.,0.418164129144046));
#29593=CARTESIAN_POINT('Ctrl Pts',(1.8590328109667,-1.,0.420157287975583));
#29594=CARTESIAN_POINT('Ctrl Pts',(1.86408083333863,-1.,0.422327307417885));
#29595=CARTESIAN_POINT('Ctrl Pts',(1.8693780394412,-1.,0.424678177290876));
#29596=CARTESIAN_POINT('Ctrl Pts',(1.87486989291333,-1.,0.427183828518743));
#29597=CARTESIAN_POINT('Ctrl Pts',(1.88044229001778,-1.,0.429803062482217));
#29598=CARTESIAN_POINT('Ctrl Pts',(1.88596913666828,-1.,0.432493038548833));
#29599=CARTESIAN_POINT('Ctrl Pts',(1.89136993975585,-1.,0.43522566096358));
#29600=CARTESIAN_POINT('Ctrl Pts',(1.89663648956549,-1.,0.437995003948443));
#29601=CARTESIAN_POINT('Ctrl Pts',(1.90180124389137,-1.,0.440807833704161));
#29602=CARTESIAN_POINT('Ctrl Pts',(1.90691756144906,-1.,0.443677556849171));
#29603=CARTESIAN_POINT('Ctrl Pts',(1.91203699981095,-1.,0.446617343485651));
#29604=CARTESIAN_POINT('Ctrl Pts',(1.91718342555717,-1.,0.449632260106572));
#29605=CARTESIAN_POINT('Ctrl Pts',(1.9223538064847,-1.,0.452719478359356));
#29606=CARTESIAN_POINT('Ctrl Pts',(1.92753067150461,-1.,0.455872005174336));
#29607=CARTESIAN_POINT('Ctrl Pts',(1.93269066517936,-1.,0.459081234547932));
#29608=CARTESIAN_POINT('Ctrl Pts',(1.93781486640834,-1.,0.462340031009087));
#29609=CARTESIAN_POINT('Ctrl Pts',(1.94289794196205,-1.,0.465645462026065));
#29610=CARTESIAN_POINT('Ctrl Pts',(1.94794381136524,-1.,0.468997482913158));
#29611=CARTESIAN_POINT('Ctrl Pts',(1.95296148278136,-1.,0.47239767226408));
#29612=CARTESIAN_POINT('Ctrl Pts',(1.95796111148175,-1.,0.475848034683172));
#29613=CARTESIAN_POINT('Ctrl Pts',(1.96294933055938,-1.,0.479349583074846));
#29614=CARTESIAN_POINT('Ctrl Pts',(1.96792703422358,-1.,0.482901662120687));
#29615=CARTESIAN_POINT('Ctrl Pts',(1.97289186263272,-1.,0.486502692907661));
#29616=CARTESIAN_POINT('Ctrl Pts',(1.97783973019229,-1.,0.490150627860955));
#29617=CARTESIAN_POINT('Ctrl Pts',(1.9827665876182,-1.,0.493843476541493));
#29618=CARTESIAN_POINT('Ctrl Pts',(1.98767044752929,-1.,0.497579909545564));
#29619=CARTESIAN_POINT('Ctrl Pts',(1.9925514912615,-1.,0.501359287727129));
#29620=CARTESIAN_POINT('Ctrl Pts',(1.99741107463567,-1.,0.505181361323011));
#29621=CARTESIAN_POINT('Ctrl Pts',(2.00225107134733,-1.,0.509046069886152));
#29622=CARTESIAN_POINT('Ctrl Pts',(2.00707309946955,-1.,0.512953306961814));
#29623=CARTESIAN_POINT('Ctrl Pts',(2.01187773939257,-1.,0.516902681728733));
#29624=CARTESIAN_POINT('Ctrl Pts',(2.01666477917305,-1.,0.520893590399429));
#29625=CARTESIAN_POINT('Ctrl Pts',(2.02143356304712,-1.,0.524925318333519));
#29626=CARTESIAN_POINT('Ctrl Pts',(2.02618329083289,-1.,0.528997127241911));
#29627=CARTESIAN_POINT('Ctrl Pts',(2.03091336214401,-1.,0.533108355132905));
#29628=CARTESIAN_POINT('Ctrl Pts',(2.03562362953993,-1.,0.537258489833135));
#29629=CARTESIAN_POINT('Ctrl Pts',(2.0403142269048,-1.,0.54144712061552));
#29630=CARTESIAN_POINT('Ctrl Pts',(2.0449854471456,-1.,0.545673903817349));
#29631=CARTESIAN_POINT('Ctrl Pts',(2.04963761077974,-1.,0.549938525150342));
#29632=CARTESIAN_POINT('Ctrl Pts',(2.05427091604482,-1.,0.55424065746411));
#29633=CARTESIAN_POINT('Ctrl Pts',(2.05888537756571,-1.,0.558579940185468));
#29634=CARTESIAN_POINT('Ctrl Pts',(2.06348090160697,-1.,0.562955993082574));
#29635=CARTESIAN_POINT('Ctrl Pts',(2.06805732997383,-1.,0.56736842118123));
#29636=CARTESIAN_POINT('Ctrl Pts',(2.07261449292757,-1.,0.571816823242411));
#29637=CARTESIAN_POINT('Ctrl Pts',(2.07715226767361,-1.,0.576300797416275));
#29638=CARTESIAN_POINT('Ctrl Pts',(2.08167059018138,-1.,0.580819952107257));
#29639=CARTESIAN_POINT('Ctrl Pts',(2.086169437277,-1.,0.585373918990895));
#29640=CARTESIAN_POINT('Ctrl Pts',(2.09064881812053,-1.,0.58996236540319));
#29641=CARTESIAN_POINT('Ctrl Pts',(2.09510876220501,-1.,0.594585006052824));
#29642=CARTESIAN_POINT('Ctrl Pts',(2.09954930865331,-1.,0.599241616422144));
#29643=CARTESIAN_POINT('Ctrl Pts',(2.10397049887709,-1.,0.603932030738212));
#29644=CARTESIAN_POINT('Ctrl Pts',(2.10749199615859,-1.,0.607711315456826));
#29645=CARTESIAN_POINT('Ctrl Pts',(2.11012443807661,-1.,0.610560911691114));
#29646=CARTESIAN_POINT('Ctrl Pts',(2.11187554260142,-1.,0.61246736556225));
#29647=CARTESIAN_POINT('Ctrl Pts',(2.11275013067528,-1.,0.613422273260091));
#29648=CARTESIAN_POINT('',(2.0698113262342,-1.,0.745574324794401));
#29649=CARTESIAN_POINT('',(2.11275013067528,-1.,0.613422273260091));
#29650=CARTESIAN_POINT('Ctrl Pts',(2.0698113262342,-1.,0.745574324794401));
#29651=CARTESIAN_POINT('Ctrl Pts',(2.06854248895575,-1.,0.74583279137781));
#29652=CARTESIAN_POINT('Ctrl Pts',(2.06600523016401,-1.,0.746345871542696));
#29653=CARTESIAN_POINT('Ctrl Pts',(2.06220058927162,-1.,0.747103932785504));
#29654=CARTESIAN_POINT('Ctrl Pts',(2.05713023030263,-1.,0.748091554181101));
#29655=CARTESIAN_POINT('Ctrl Pts',(2.05079645591606,-1.,0.749287468663053));
#29656=CARTESIAN_POINT('Ctrl Pts',(2.04446689147754,-1.,0.750444657874758));
#29657=CARTESIAN_POINT('Ctrl Pts',(2.03814160092173,-1.,0.751562963361384));
#29658=CARTESIAN_POINT('Ctrl Pts',(2.03182068456467,-1.,0.752642180488104));
#29659=CARTESIAN_POINT('Ctrl Pts',(2.02550428623587,-1.,0.753682061113766));
#29660=CARTESIAN_POINT('Ctrl Pts',(2.01919259406003,-1.,0.75468233072352));
#29661=CARTESIAN_POINT('Ctrl Pts',(2.01288584328149,-1.,0.755642704958101));
#29662=CARTESIAN_POINT('Ctrl Pts',(2.00658431587682,-1.,0.756562904646496));
#29663=CARTESIAN_POINT('Ctrl Pts',(2.00028834739072,-1.,0.757442676862342));
#29664=CARTESIAN_POINT('Ctrl Pts',(1.9939983109871,-1.,0.758281796766377));
#29665=CARTESIAN_POINT('Ctrl Pts',(1.98771456680806,-1.,0.759080037802243));
#29666=CARTESIAN_POINT('Ctrl Pts',(1.98143741418156,-1.,0.759837147452135));
#29667=CARTESIAN_POINT('Ctrl Pts',(1.97516705321521,-1.,0.760552825409856));
#29668=CARTESIAN_POINT('Ctrl Pts',(1.96890351582545,-1.,0.761226690483986));
#29669=CARTESIAN_POINT('Ctrl Pts',(1.96264672744229,-1.,0.761858300014575));
#29670=CARTESIAN_POINT('Ctrl Pts',(1.95639665309893,-1.,0.762447203806264));
#29671=CARTESIAN_POINT('Ctrl Pts',(1.95015342590025,-1.,0.762992990878774));
#29672=CARTESIAN_POINT('Ctrl Pts',(1.94391746617626,-1.,0.763495333538581));
#29673=CARTESIAN_POINT('Ctrl Pts',(1.93768964875867,-1.,0.763954049121394));
#29674=CARTESIAN_POINT('Ctrl Pts',(1.93147105496367,-1.,0.76436901067389));
#29675=CARTESIAN_POINT('Ctrl Pts',(1.92526263537041,-1.,0.764740025488189));
#29676=CARTESIAN_POINT('Ctrl Pts',(1.91906491634197,-1.,0.765066729667095));
#29677=CARTESIAN_POINT('Ctrl Pts',(1.91287765805174,-1.,0.765348465884739));
#29678=CARTESIAN_POINT('Ctrl Pts',(1.90669961402362,-1.,0.765584196937937));
#29679=CARTESIAN_POINT('Ctrl Pts',(1.90052930393599,-1.,0.765772772593395));
#29680=CARTESIAN_POINT('Ctrl Pts',(1.89436577771389,-1.,0.765913193856979));
#29681=CARTESIAN_POINT('Ctrl Pts',(1.88820926433409,-1.,0.76600483706209));
#29682=CARTESIAN_POINT('Ctrl Pts',(1.88206215302561,-1.,0.766047794851869));
#29683=CARTESIAN_POINT('Ctrl Pts',(1.87592888967886,-1.,0.766042837036759));
#29684=CARTESIAN_POINT('Ctrl Pts',(1.86981398314345,-1.,0.765990708546112));
#29685=CARTESIAN_POINT('Ctrl Pts',(1.86372027063314,-1.,0.765891519092557));
#29686=CARTESIAN_POINT('Ctrl Pts',(1.85764741390391,-1.,0.765744212909305));
#29687=CARTESIAN_POINT('Ctrl Pts',(1.85158945130054,-1.,0.765545710619023));
#29688=CARTESIAN_POINT('Ctrl Pts',(1.8455369887591,-1.,0.765291664861972));
#29689=CARTESIAN_POINT('Ctrl Pts',(1.83948181064823,-1.,0.764978057881688));
#29690=CARTESIAN_POINT('Ctrl Pts',(1.8334207722714,-1.,0.764602549687846));
#29691=CARTESIAN_POINT('Ctrl Pts',(1.8273599120008,-1.,0.764165902606056));
#29692=CARTESIAN_POINT('Ctrl Pts',(1.82131873145297,-1.,0.763673465462854));
#29693=CARTESIAN_POINT('Ctrl Pts',(1.81532118405566,-1.,0.763132003836783));
#29694=CARTESIAN_POINT('Ctrl Pts',(1.80938551463989,-1.,0.762546129464036));
#29695=CARTESIAN_POINT('Ctrl Pts',(1.80351583877334,-1.,0.761915336443516));
#29696=CARTESIAN_POINT('Ctrl Pts',(1.79768986997735,-1.,0.761229695230359));
#29697=CARTESIAN_POINT('Ctrl Pts',(1.79185815610802,-1.,0.760469555880425));
#29698=CARTESIAN_POINT('Ctrl Pts',(1.78596964884526,-1.,0.759614401109868));
#29699=CARTESIAN_POINT('Ctrl Pts',(1.77999411220912,-1.,0.75865062667738));
#29700=CARTESIAN_POINT('Ctrl Pts',(1.77394167108342,-1.,0.757578264077238));
#29701=CARTESIAN_POINT('Ctrl Pts',(1.76789396003141,-1.,0.756421896028403));
#29702=CARTESIAN_POINT('Ctrl Pts',(1.7619781724032,-1.,0.755220979975262));
#29703=CARTESIAN_POINT('Ctrl Pts',(1.75631083600175,-1.,0.75400925402848));
#29704=CARTESIAN_POINT('Ctrl Pts',(1.75095139468809,-1.,0.752797683531377));
#29705=CARTESIAN_POINT('Ctrl Pts',(1.74585086852298,-1.,0.751555614163629));
#29706=CARTESIAN_POINT('Ctrl Pts',(1.74080458266705,-1.,0.750193435979541));
#29707=CARTESIAN_POINT('Ctrl Pts',(1.73550351679848,-1.,0.748582462954855));
#29708=CARTESIAN_POINT('Ctrl Pts',(1.72958533647399,-1.,0.746574710096437));
#29709=CARTESIAN_POINT('Ctrl Pts',(1.7226822991693,-1.,0.744021445433765));
#29710=CARTESIAN_POINT('Ctrl Pts',(1.71447789751927,-1.,0.740795162032088));
#29711=CARTESIAN_POINT('Ctrl Pts',(1.70473309006121,-1.,0.736799665724771));
#29712=CARTESIAN_POINT('Ctrl Pts',(1.69326921975743,-1.,0.731963238697195));
#29713=CARTESIAN_POINT('Ctrl Pts',(1.67996158455503,-1.,0.726235967997433));
#29714=CARTESIAN_POINT('Ctrl Pts',(1.6647288055568,-1.,0.719585433804282));
#29715=CARTESIAN_POINT('Ctrl Pts',(1.64752408832016,-1.,0.711993139355394));
#29716=CARTESIAN_POINT('Ctrl Pts',(1.63216541664676,-1.,0.705159151988319));
#29717=CARTESIAN_POINT('Ctrl Pts',(1.61974673472612,-1.,0.699605146405088));
#29718=CARTESIAN_POINT('Ctrl Pts',(1.61106790958151,-1.,0.695712097881194));
#29719=CARTESIAN_POINT('Ctrl Pts',(1.60662857109684,-1.,0.693717979106306));
#29720=CARTESIAN_POINT('Origin',(0.,-1.,0.));
#29721=CARTESIAN_POINT('Origin',(0.,0.,0.));
#29722=CARTESIAN_POINT('Origin',(0.,2.2,0.));
#29723=CARTESIAN_POINT('Origin',(0.,1.,0.));
#29724=CARTESIAN_POINT('',(-1.4,2.2,1.71450551880629E-16));
#29725=CARTESIAN_POINT('Origin',(0.,2.2,0.));
#29726=CARTESIAN_POINT('',(-1.4,1.,1.71450551880629E-16));
#29727=CARTESIAN_POINT('',(-1.4,1.,1.71450551880629E-16));
#29728=CARTESIAN_POINT('Origin',(0.,1.,0.));
#29729=CARTESIAN_POINT('Origin',(0.,2.2,0.));
#29730=CARTESIAN_POINT('Ctrl Pts',(2.11275013067528,-1.,0.613422273260091));
#29731=CARTESIAN_POINT('Ctrl Pts',(2.11275013067528,1.,0.613422273260091));
#29732=CARTESIAN_POINT('Ctrl Pts',(2.11187554260142,-1.,0.61246736556225));
#29733=CARTESIAN_POINT('Ctrl Pts',(2.11187554260142,1.,0.61246736556225));
#29734=CARTESIAN_POINT('Ctrl Pts',(2.11012443807661,-1.,0.610560911691114));
#29735=CARTESIAN_POINT('Ctrl Pts',(2.11012443807661,1.,0.610560911691114));
#29736=CARTESIAN_POINT('Ctrl Pts',(2.10749199615859,-1.,0.607711315456826));
#29737=CARTESIAN_POINT('Ctrl Pts',(2.10749199615859,1.,0.607711315456826));
#29738=CARTESIAN_POINT('Ctrl Pts',(2.10397049887709,-1.,0.603932030738212));
#29739=CARTESIAN_POINT('Ctrl Pts',(2.10397049887709,1.,0.603932030738212));
#29740=CARTESIAN_POINT('Ctrl Pts',(2.09954930865331,-1.,0.599241616422144));
#29741=CARTESIAN_POINT('Ctrl Pts',(2.09954930865331,1.,0.599241616422144));
#29742=CARTESIAN_POINT('Ctrl Pts',(2.09510876220501,-1.,0.594585006052824));
#29743=CARTESIAN_POINT('Ctrl Pts',(2.09510876220501,1.,0.594585006052824));
#29744=CARTESIAN_POINT('Ctrl Pts',(2.09064881812053,-1.,0.58996236540319));
#29745=CARTESIAN_POINT('Ctrl Pts',(2.09064881812053,1.,0.58996236540319));
#29746=CARTESIAN_POINT('Ctrl Pts',(2.086169437277,-1.,0.585373918990895));
#29747=CARTESIAN_POINT('Ctrl Pts',(2.086169437277,1.,0.585373918990895));
#29748=CARTESIAN_POINT('Ctrl Pts',(2.08167059018138,-1.,0.580819952107257));
#29749=CARTESIAN_POINT('Ctrl Pts',(2.08167059018138,1.,0.580819952107257));
#29750=CARTESIAN_POINT('Ctrl Pts',(2.07715226767361,-1.,0.576300797416275));
#29751=CARTESIAN_POINT('Ctrl Pts',(2.07715226767361,1.,0.576300797416275));
#29752=CARTESIAN_POINT('Ctrl Pts',(2.07261449292757,-1.,0.571816823242411));
#29753=CARTESIAN_POINT('Ctrl Pts',(2.07261449292757,1.,0.571816823242411));
#29754=CARTESIAN_POINT('Ctrl Pts',(2.06805732997383,-1.,0.56736842118123));
#29755=CARTESIAN_POINT('Ctrl Pts',(2.06805732997383,1.,0.56736842118123));
#29756=CARTESIAN_POINT('Ctrl Pts',(2.06348090160697,-1.,0.562955993082574));
#29757=CARTESIAN_POINT('Ctrl Pts',(2.06348090160697,1.,0.562955993082574));
#29758=CARTESIAN_POINT('Ctrl Pts',(2.05888537756571,-1.,0.558579940185468));
#29759=CARTESIAN_POINT('Ctrl Pts',(2.05888537756571,1.,0.558579940185468));
#29760=CARTESIAN_POINT('Ctrl Pts',(2.05427091604482,-1.,0.55424065746411));
#29761=CARTESIAN_POINT('Ctrl Pts',(2.05427091604482,1.,0.55424065746411));
#29762=CARTESIAN_POINT('Ctrl Pts',(2.04963761077974,-1.,0.549938525150342));
#29763=CARTESIAN_POINT('Ctrl Pts',(2.04963761077974,1.,0.549938525150342));
#29764=CARTESIAN_POINT('Ctrl Pts',(2.0449854471456,-1.,0.545673903817349));
#29765=CARTESIAN_POINT('Ctrl Pts',(2.0449854471456,1.,0.545673903817349));
#29766=CARTESIAN_POINT('Ctrl Pts',(2.0403142269048,-1.,0.54144712061552));
#29767=CARTESIAN_POINT('Ctrl Pts',(2.0403142269048,1.,0.54144712061552));
#29768=CARTESIAN_POINT('Ctrl Pts',(2.03562362953993,-1.,0.537258489833135));
#29769=CARTESIAN_POINT('Ctrl Pts',(2.03562362953993,1.,0.537258489833135));
#29770=CARTESIAN_POINT('Ctrl Pts',(2.03091336214401,-1.,0.533108355132905));
#29771=CARTESIAN_POINT('Ctrl Pts',(2.03091336214401,1.,0.533108355132905));
#29772=CARTESIAN_POINT('Ctrl Pts',(2.02618329083289,-1.,0.528997127241911));
#29773=CARTESIAN_POINT('Ctrl Pts',(2.02618329083289,1.,0.528997127241911));
#29774=CARTESIAN_POINT('Ctrl Pts',(2.02143356304712,-1.,0.524925318333519));
#29775=CARTESIAN_POINT('Ctrl Pts',(2.02143356304712,1.,0.524925318333519));
#29776=CARTESIAN_POINT('Ctrl Pts',(2.01666477917305,-1.,0.520893590399429));
#29777=CARTESIAN_POINT('Ctrl Pts',(2.01666477917305,1.,0.520893590399429));
#29778=CARTESIAN_POINT('Ctrl Pts',(2.01187773939257,-1.,0.516902681728733));
#29779=CARTESIAN_POINT('Ctrl Pts',(2.01187773939257,1.,0.516902681728733));
#29780=CARTESIAN_POINT('Ctrl Pts',(2.00707309946955,-1.,0.512953306961814));
#29781=CARTESIAN_POINT('Ctrl Pts',(2.00707309946955,1.,0.512953306961814));
#29782=CARTESIAN_POINT('Ctrl Pts',(2.00225107134733,-1.,0.509046069886152));
#29783=CARTESIAN_POINT('Ctrl Pts',(2.00225107134733,1.,0.509046069886152));
#29784=CARTESIAN_POINT('Ctrl Pts',(1.99741107463567,-1.,0.505181361323011));
#29785=CARTESIAN_POINT('Ctrl Pts',(1.99741107463567,1.,0.505181361323011));
#29786=CARTESIAN_POINT('Ctrl Pts',(1.9925514912615,-1.,0.501359287727129));
#29787=CARTESIAN_POINT('Ctrl Pts',(1.9925514912615,1.,0.501359287727129));
#29788=CARTESIAN_POINT('Ctrl Pts',(1.98767044752929,-1.,0.497579909545564));
#29789=CARTESIAN_POINT('Ctrl Pts',(1.98767044752929,1.,0.497579909545564));
#29790=CARTESIAN_POINT('Ctrl Pts',(1.9827665876182,-1.,0.493843476541493));
#29791=CARTESIAN_POINT('Ctrl Pts',(1.9827665876182,1.,0.493843476541493));
#29792=CARTESIAN_POINT('Ctrl Pts',(1.97783973019229,-1.,0.490150627860955));
#29793=CARTESIAN_POINT('Ctrl Pts',(1.97783973019229,1.,0.490150627860955));
#29794=CARTESIAN_POINT('Ctrl Pts',(1.97289186263272,-1.,0.486502692907661));
#29795=CARTESIAN_POINT('Ctrl Pts',(1.97289186263272,1.,0.486502692907661));
#29796=CARTESIAN_POINT('Ctrl Pts',(1.96792703422358,-1.,0.482901662120687));
#29797=CARTESIAN_POINT('Ctrl Pts',(1.96792703422358,1.,0.482901662120687));
#29798=CARTESIAN_POINT('Ctrl Pts',(1.96294933055938,-1.,0.479349583074846));
#29799=CARTESIAN_POINT('Ctrl Pts',(1.96294933055938,1.,0.479349583074846));
#29800=CARTESIAN_POINT('Ctrl Pts',(1.95796111148175,-1.,0.475848034683172));
#29801=CARTESIAN_POINT('Ctrl Pts',(1.95796111148175,1.,0.475848034683172));
#29802=CARTESIAN_POINT('Ctrl Pts',(1.95296148278136,-1.,0.47239767226408));
#29803=CARTESIAN_POINT('Ctrl Pts',(1.95296148278136,1.,0.47239767226408));
#29804=CARTESIAN_POINT('Ctrl Pts',(1.94794381136524,-1.,0.468997482913158));
#29805=CARTESIAN_POINT('Ctrl Pts',(1.94794381136524,1.,0.468997482913158));
#29806=CARTESIAN_POINT('Ctrl Pts',(1.94289794196205,-1.,0.465645462026065));
#29807=CARTESIAN_POINT('Ctrl Pts',(1.94289794196205,1.,0.465645462026065));
#29808=CARTESIAN_POINT('Ctrl Pts',(1.93781486640834,-1.,0.462340031009087));
#29809=CARTESIAN_POINT('Ctrl Pts',(1.93781486640834,1.,0.462340031009087));
#29810=CARTESIAN_POINT('Ctrl Pts',(1.93269066517936,-1.,0.459081234547932));
#29811=CARTESIAN_POINT('Ctrl Pts',(1.93269066517936,1.,0.459081234547932));
#29812=CARTESIAN_POINT('Ctrl Pts',(1.92753067150461,-1.,0.455872005174336));
#29813=CARTESIAN_POINT('Ctrl Pts',(1.92753067150461,1.,0.455872005174336));
#29814=CARTESIAN_POINT('Ctrl Pts',(1.9223538064847,-1.,0.452719478359356));
#29815=CARTESIAN_POINT('Ctrl Pts',(1.9223538064847,1.,0.452719478359356));
#29816=CARTESIAN_POINT('Ctrl Pts',(1.91718342555717,-1.,0.449632260106572));
#29817=CARTESIAN_POINT('Ctrl Pts',(1.91718342555717,1.,0.449632260106572));
#29818=CARTESIAN_POINT('Ctrl Pts',(1.91203699981095,-1.,0.446617343485651));
#29819=CARTESIAN_POINT('Ctrl Pts',(1.91203699981095,1.,0.446617343485651));
#29820=CARTESIAN_POINT('Ctrl Pts',(1.90691756144906,-1.,0.443677556849171));
#29821=CARTESIAN_POINT('Ctrl Pts',(1.90691756144906,1.,0.443677556849171));
#29822=CARTESIAN_POINT('Ctrl Pts',(1.90180124389137,-1.,0.440807833704161));
#29823=CARTESIAN_POINT('Ctrl Pts',(1.90180124389137,1.,0.440807833704161));
#29824=CARTESIAN_POINT('Ctrl Pts',(1.89663648956549,-1.,0.437995003948443));
#29825=CARTESIAN_POINT('Ctrl Pts',(1.89663648956549,1.,0.437995003948443));
#29826=CARTESIAN_POINT('Ctrl Pts',(1.89136993975585,-1.,0.43522566096358));
#29827=CARTESIAN_POINT('Ctrl Pts',(1.89136993975585,1.,0.43522566096358));
#29828=CARTESIAN_POINT('Ctrl Pts',(1.88596913666828,-1.,0.432493038548833));
#29829=CARTESIAN_POINT('Ctrl Pts',(1.88596913666828,1.,0.432493038548833));
#29830=CARTESIAN_POINT('Ctrl Pts',(1.88044229001778,-1.,0.429803062482217));
#29831=CARTESIAN_POINT('Ctrl Pts',(1.88044229001778,1.,0.429803062482217));
#29832=CARTESIAN_POINT('Ctrl Pts',(1.87486989291333,-1.,0.427183828518743));
#29833=CARTESIAN_POINT('Ctrl Pts',(1.87486989291333,1.,0.427183828518743));
#29834=CARTESIAN_POINT('Ctrl Pts',(1.8693780394412,-1.,0.424678177290876));
#29835=CARTESIAN_POINT('Ctrl Pts',(1.8693780394412,1.,0.424678177290876));
#29836=CARTESIAN_POINT('Ctrl Pts',(1.86408083333863,-1.,0.422327307417885));
#29837=CARTESIAN_POINT('Ctrl Pts',(1.86408083333863,1.,0.422327307417885));
#29838=CARTESIAN_POINT('Ctrl Pts',(1.8590328109667,-1.,0.420157287975583));
#29839=CARTESIAN_POINT('Ctrl Pts',(1.8590328109667,1.,0.420157287975583));
#29840=CARTESIAN_POINT('Ctrl Pts',(1.8541763285645,-1.,0.418164129144046));
#29841=CARTESIAN_POINT('Ctrl Pts',(1.8541763285645,1.,0.418164129144046));
#29842=CARTESIAN_POINT('Ctrl Pts',(1.84929312930314,-1.,0.416300022039885));
#29843=CARTESIAN_POINT('Ctrl Pts',(1.84929312930314,1.,0.416300022039885));
#29844=CARTESIAN_POINT('Ctrl Pts',(1.84405757074218,-1.,0.414487438255542));
#29845=CARTESIAN_POINT('Ctrl Pts',(1.84405757074218,1.,0.414487438255542));
#29846=CARTESIAN_POINT('Ctrl Pts',(1.8380895347617,-1.,0.412633125322945));
#29847=CARTESIAN_POINT('Ctrl Pts',(1.8380895347617,1.,0.412633125322945));
#29848=CARTESIAN_POINT('Ctrl Pts',(1.83100408895047,-1.,0.410641256301276));
#29849=CARTESIAN_POINT('Ctrl Pts',(1.83100408895047,1.,0.410641256301276));
#29850=CARTESIAN_POINT('Ctrl Pts',(1.82247022677562,-1.,0.408428948106228));
#29851=CARTESIAN_POINT('Ctrl Pts',(1.82247022677562,1.,0.408428948106228));
#29852=CARTESIAN_POINT('Ctrl Pts',(1.81223801812013,-1.,0.405933518407176));
#29853=CARTESIAN_POINT('Ctrl Pts',(1.81223801812013,1.,0.405933518407176));
#29854=CARTESIAN_POINT('Ctrl Pts',(1.80012077173238,-1.,0.403107976163396));
#29855=CARTESIAN_POINT('Ctrl Pts',(1.80012077173238,1.,0.403107976163396));
#29856=CARTESIAN_POINT('Ctrl Pts',(1.78598826343754,-1.,0.399919403774156));
#29857=CARTESIAN_POINT('Ctrl Pts',(1.78598826343754,1.,0.399919403774156));
#29858=CARTESIAN_POINT('Ctrl Pts',(1.76975560043442,-1.,0.396346196110688));
#29859=CARTESIAN_POINT('Ctrl Pts',(1.76975560043442,1.,0.396346196110688));
#29860=CARTESIAN_POINT('Ctrl Pts',(1.75137405310193,-1.,0.392375812285396));
#29861=CARTESIAN_POINT('Ctrl Pts',(1.75137405310193,1.,0.392375812285396));
#29862=CARTESIAN_POINT('Ctrl Pts',(1.73493170972829,-1.,0.388877023502615));
#29863=CARTESIAN_POINT('Ctrl Pts',(1.73493170972829,1.,0.388877023502615));
#29864=CARTESIAN_POINT('Ctrl Pts',(1.72162022244582,-1.,0.386070790323281));
#29865=CARTESIAN_POINT('Ctrl Pts',(1.72162022244582,1.,0.386070790323281));
#29866=CARTESIAN_POINT('Ctrl Pts',(1.71231062891398,-1.,0.384119047314215));
#29867=CARTESIAN_POINT('Ctrl Pts',(1.71231062891398,1.,0.384119047314215));
#29868=CARTESIAN_POINT('Ctrl Pts',(1.7075470150345,-1.,0.383122945602004));
#29869=CARTESIAN_POINT('Ctrl Pts',(1.7075470150345,1.,0.383122945602004));
#29870=CARTESIAN_POINT('',(1.7075470150345,1.,0.383122945602004));
#29871=CARTESIAN_POINT('',(1.7075470150345,0.,0.383122945602005));
#29872=CARTESIAN_POINT('',(2.11275013067528,1.,0.613422273260091));
#29873=CARTESIAN_POINT('Ctrl Pts',(2.11275013067528,1.,0.613422273260091));
#29874=CARTESIAN_POINT('Ctrl Pts',(2.11187554260142,1.,0.61246736556225));
#29875=CARTESIAN_POINT('Ctrl Pts',(2.11012443807661,1.,0.610560911691114));
#29876=CARTESIAN_POINT('Ctrl Pts',(2.10749199615859,1.,0.607711315456826));
#29877=CARTESIAN_POINT('Ctrl Pts',(2.10397049887709,1.,0.603932030738212));
#29878=CARTESIAN_POINT('Ctrl Pts',(2.09954930865331,1.,0.599241616422144));
#29879=CARTESIAN_POINT('Ctrl Pts',(2.09510876220501,1.,0.594585006052824));
#29880=CARTESIAN_POINT('Ctrl Pts',(2.09064881812053,1.,0.58996236540319));
#29881=CARTESIAN_POINT('Ctrl Pts',(2.086169437277,1.,0.585373918990895));
#29882=CARTESIAN_POINT('Ctrl Pts',(2.08167059018138,1.,0.580819952107257));
#29883=CARTESIAN_POINT('Ctrl Pts',(2.07715226767361,1.,0.576300797416275));
#29884=CARTESIAN_POINT('Ctrl Pts',(2.07261449292757,1.,0.571816823242411));
#29885=CARTESIAN_POINT('Ctrl Pts',(2.06805732997383,1.,0.56736842118123));
#29886=CARTESIAN_POINT('Ctrl Pts',(2.06348090160697,1.,0.562955993082574));
#29887=CARTESIAN_POINT('Ctrl Pts',(2.05888537756571,1.,0.558579940185468));
#29888=CARTESIAN_POINT('Ctrl Pts',(2.05427091604482,1.,0.55424065746411));
#29889=CARTESIAN_POINT('Ctrl Pts',(2.04963761077974,1.,0.549938525150342));
#29890=CARTESIAN_POINT('Ctrl Pts',(2.0449854471456,1.,0.545673903817349));
#29891=CARTESIAN_POINT('Ctrl Pts',(2.0403142269048,1.,0.54144712061552));
#29892=CARTESIAN_POINT('Ctrl Pts',(2.03562362953993,1.,0.537258489833135));
#29893=CARTESIAN_POINT('Ctrl Pts',(2.03091336214401,1.,0.533108355132905));
#29894=CARTESIAN_POINT('Ctrl Pts',(2.02618329083289,1.,0.528997127241911));
#29895=CARTESIAN_POINT('Ctrl Pts',(2.02143356304712,1.,0.524925318333519));
#29896=CARTESIAN_POINT('Ctrl Pts',(2.01666477917305,1.,0.520893590399429));
#29897=CARTESIAN_POINT('Ctrl Pts',(2.01187773939257,1.,0.516902681728733));
#29898=CARTESIAN_POINT('Ctrl Pts',(2.00707309946955,1.,0.512953306961814));
#29899=CARTESIAN_POINT('Ctrl Pts',(2.00225107134733,1.,0.509046069886152));
#29900=CARTESIAN_POINT('Ctrl Pts',(1.99741107463567,1.,0.505181361323011));
#29901=CARTESIAN_POINT('Ctrl Pts',(1.9925514912615,1.,0.501359287727129));
#29902=CARTESIAN_POINT('Ctrl Pts',(1.98767044752929,1.,0.497579909545564));
#29903=CARTESIAN_POINT('Ctrl Pts',(1.9827665876182,1.,0.493843476541493));
#29904=CARTESIAN_POINT('Ctrl Pts',(1.97783973019229,1.,0.490150627860955));
#29905=CARTESIAN_POINT('Ctrl Pts',(1.97289186263272,1.,0.486502692907661));
#29906=CARTESIAN_POINT('Ctrl Pts',(1.96792703422358,1.,0.482901662120687));
#29907=CARTESIAN_POINT('Ctrl Pts',(1.96294933055938,1.,0.479349583074846));
#29908=CARTESIAN_POINT('Ctrl Pts',(1.95796111148175,1.,0.475848034683172));
#29909=CARTESIAN_POINT('Ctrl Pts',(1.95296148278136,1.,0.47239767226408));
#29910=CARTESIAN_POINT('Ctrl Pts',(1.94794381136524,1.,0.468997482913158));
#29911=CARTESIAN_POINT('Ctrl Pts',(1.94289794196205,1.,0.465645462026065));
#29912=CARTESIAN_POINT('Ctrl Pts',(1.93781486640834,1.,0.462340031009087));
#29913=CARTESIAN_POINT('Ctrl Pts',(1.93269066517936,1.,0.459081234547932));
#29914=CARTESIAN_POINT('Ctrl Pts',(1.92753067150461,1.,0.455872005174336));
#29915=CARTESIAN_POINT('Ctrl Pts',(1.9223538064847,1.,0.452719478359356));
#29916=CARTESIAN_POINT('Ctrl Pts',(1.91718342555717,1.,0.449632260106572));
#29917=CARTESIAN_POINT('Ctrl Pts',(1.91203699981095,1.,0.446617343485651));
#29918=CARTESIAN_POINT('Ctrl Pts',(1.90691756144906,1.,0.443677556849171));
#29919=CARTESIAN_POINT('Ctrl Pts',(1.90180124389137,1.,0.440807833704161));
#29920=CARTESIAN_POINT('Ctrl Pts',(1.89663648956549,1.,0.437995003948443));
#29921=CARTESIAN_POINT('Ctrl Pts',(1.89136993975585,1.,0.43522566096358));
#29922=CARTESIAN_POINT('Ctrl Pts',(1.88596913666828,1.,0.432493038548833));
#29923=CARTESIAN_POINT('Ctrl Pts',(1.88044229001778,1.,0.429803062482217));
#29924=CARTESIAN_POINT('Ctrl Pts',(1.87486989291333,1.,0.427183828518743));
#29925=CARTESIAN_POINT('Ctrl Pts',(1.8693780394412,1.,0.424678177290876));
#29926=CARTESIAN_POINT('Ctrl Pts',(1.86408083333863,1.,0.422327307417885));
#29927=CARTESIAN_POINT('Ctrl Pts',(1.8590328109667,1.,0.420157287975583));
#29928=CARTESIAN_POINT('Ctrl Pts',(1.8541763285645,1.,0.418164129144046));
#29929=CARTESIAN_POINT('Ctrl Pts',(1.84929312930314,1.,0.416300022039885));
#29930=CARTESIAN_POINT('Ctrl Pts',(1.84405757074218,1.,0.414487438255542));
#29931=CARTESIAN_POINT('Ctrl Pts',(1.8380895347617,1.,0.412633125322945));
#29932=CARTESIAN_POINT('Ctrl Pts',(1.83100408895047,1.,0.410641256301276));
#29933=CARTESIAN_POINT('Ctrl Pts',(1.82247022677562,1.,0.408428948106228));
#29934=CARTESIAN_POINT('Ctrl Pts',(1.81223801812013,1.,0.405933518407176));
#29935=CARTESIAN_POINT('Ctrl Pts',(1.80012077173238,1.,0.403107976163396));
#29936=CARTESIAN_POINT('Ctrl Pts',(1.78598826343754,1.,0.399919403774156));
#29937=CARTESIAN_POINT('Ctrl Pts',(1.76975560043442,1.,0.396346196110688));
#29938=CARTESIAN_POINT('Ctrl Pts',(1.75137405310193,1.,0.392375812285396));
#29939=CARTESIAN_POINT('Ctrl Pts',(1.73493170972829,1.,0.388877023502615));
#29940=CARTESIAN_POINT('Ctrl Pts',(1.72162022244582,1.,0.386070790323281));
#29941=CARTESIAN_POINT('Ctrl Pts',(1.71231062891398,1.,0.384119047314215));
#29942=CARTESIAN_POINT('Ctrl Pts',(1.7075470150345,1.,0.383122945602004));
#29943=CARTESIAN_POINT('',(2.11275013067528,0.,0.613422273260091));
#29944=CARTESIAN_POINT('Origin',(2.0698113262342,0.,0.745574324794401));
#29945=CARTESIAN_POINT('',(2.0698113262342,1.,0.745574324794401));
#29946=CARTESIAN_POINT('',(2.11275013067528,1.,0.613422273260091));
#29947=CARTESIAN_POINT('',(2.0698113262342,0.,0.745574324794401));
#29948=CARTESIAN_POINT('Ctrl Pts',(1.60662857109684,-1.,0.693717979106306));
#29949=CARTESIAN_POINT('Ctrl Pts',(1.60662857109684,1.,0.693717979106306));
#29950=CARTESIAN_POINT('Ctrl Pts',(1.61106790958151,-1.,0.695712097881194));
#29951=CARTESIAN_POINT('Ctrl Pts',(1.61106790958151,1.,0.695712097881194));
#29952=CARTESIAN_POINT('Ctrl Pts',(1.61974673472612,-1.,0.699605146405088));
#29953=CARTESIAN_POINT('Ctrl Pts',(1.61974673472612,1.,0.699605146405088));
#29954=CARTESIAN_POINT('Ctrl Pts',(1.63216541664676,-1.,0.705159151988319));
#29955=CARTESIAN_POINT('Ctrl Pts',(1.63216541664676,1.,0.705159151988319));
#29956=CARTESIAN_POINT('Ctrl Pts',(1.64752408832016,-1.,0.711993139355394));
#29957=CARTESIAN_POINT('Ctrl Pts',(1.64752408832016,1.,0.711993139355394));
#29958=CARTESIAN_POINT('Ctrl Pts',(1.6647288055568,-1.,0.719585433804282));
#29959=CARTESIAN_POINT('Ctrl Pts',(1.6647288055568,1.,0.719585433804282));
#29960=CARTESIAN_POINT('Ctrl Pts',(1.67996158455503,-1.,0.726235967997433));
#29961=CARTESIAN_POINT('Ctrl Pts',(1.67996158455503,1.,0.726235967997433));
#29962=CARTESIAN_POINT('Ctrl Pts',(1.69326921975743,-1.,0.731963238697195));
#29963=CARTESIAN_POINT('Ctrl Pts',(1.69326921975743,1.,0.731963238697195));
#29964=CARTESIAN_POINT('Ctrl Pts',(1.70473309006121,-1.,0.736799665724771));
#29965=CARTESIAN_POINT('Ctrl Pts',(1.70473309006121,1.,0.736799665724771));
#29966=CARTESIAN_POINT('Ctrl Pts',(1.71447789751927,-1.,0.740795162032088));
#29967=CARTESIAN_POINT('Ctrl Pts',(1.71447789751927,1.,0.740795162032088));
#29968=CARTESIAN_POINT('Ctrl Pts',(1.7226822991693,-1.,0.744021445433765));
#29969=CARTESIAN_POINT('Ctrl Pts',(1.7226822991693,1.,0.744021445433765));
#29970=CARTESIAN_POINT('Ctrl Pts',(1.72958533647399,-1.,0.746574710096437));
#29971=CARTESIAN_POINT('Ctrl Pts',(1.72958533647399,1.,0.746574710096437));
#29972=CARTESIAN_POINT('Ctrl Pts',(1.73550351679848,-1.,0.748582462954855));
#29973=CARTESIAN_POINT('Ctrl Pts',(1.73550351679848,1.,0.748582462954855));
#29974=CARTESIAN_POINT('Ctrl Pts',(1.74080458266705,-1.,0.750193435979541));
#29975=CARTESIAN_POINT('Ctrl Pts',(1.74080458266705,1.,0.750193435979541));
#29976=CARTESIAN_POINT('Ctrl Pts',(1.74585086852298,-1.,0.751555614163629));
#29977=CARTESIAN_POINT('Ctrl Pts',(1.74585086852298,1.,0.751555614163629));
#29978=CARTESIAN_POINT('Ctrl Pts',(1.75095139468809,-1.,0.752797683531377));
#29979=CARTESIAN_POINT('Ctrl Pts',(1.75095139468809,1.,0.752797683531377));
#29980=CARTESIAN_POINT('Ctrl Pts',(1.75631083600175,-1.,0.75400925402848));
#29981=CARTESIAN_POINT('Ctrl Pts',(1.75631083600175,1.,0.75400925402848));
#29982=CARTESIAN_POINT('Ctrl Pts',(1.7619781724032,-1.,0.755220979975262));
#29983=CARTESIAN_POINT('Ctrl Pts',(1.7619781724032,1.,0.755220979975262));
#29984=CARTESIAN_POINT('Ctrl Pts',(1.76789396003141,-1.,0.756421896028403));
#29985=CARTESIAN_POINT('Ctrl Pts',(1.76789396003141,1.,0.756421896028403));
#29986=CARTESIAN_POINT('Ctrl Pts',(1.77394167108342,-1.,0.757578264077238));
#29987=CARTESIAN_POINT('Ctrl Pts',(1.77394167108342,1.,0.757578264077238));
#29988=CARTESIAN_POINT('Ctrl Pts',(1.77999411220912,-1.,0.75865062667738));
#29989=CARTESIAN_POINT('Ctrl Pts',(1.77999411220912,1.,0.75865062667738));
#29990=CARTESIAN_POINT('Ctrl Pts',(1.78596964884526,-1.,0.759614401109868));
#29991=CARTESIAN_POINT('Ctrl Pts',(1.78596964884526,1.,0.759614401109868));
#29992=CARTESIAN_POINT('Ctrl Pts',(1.79185815610802,-1.,0.760469555880425));
#29993=CARTESIAN_POINT('Ctrl Pts',(1.79185815610802,1.,0.760469555880425));
#29994=CARTESIAN_POINT('Ctrl Pts',(1.79768986997735,-1.,0.761229695230359));
#29995=CARTESIAN_POINT('Ctrl Pts',(1.79768986997735,1.,0.761229695230359));
#29996=CARTESIAN_POINT('Ctrl Pts',(1.80351583877334,-1.,0.761915336443516));
#29997=CARTESIAN_POINT('Ctrl Pts',(1.80351583877334,1.,0.761915336443516));
#29998=CARTESIAN_POINT('Ctrl Pts',(1.80938551463989,-1.,0.762546129464036));
#29999=CARTESIAN_POINT('Ctrl Pts',(1.80938551463989,1.,0.762546129464036));
#30000=CARTESIAN_POINT('Ctrl Pts',(1.81532118405566,-1.,0.763132003836783));
#30001=CARTESIAN_POINT('Ctrl Pts',(1.81532118405566,1.,0.763132003836783));
#30002=CARTESIAN_POINT('Ctrl Pts',(1.82131873145297,-1.,0.763673465462854));
#30003=CARTESIAN_POINT('Ctrl Pts',(1.82131873145297,1.,0.763673465462854));
#30004=CARTESIAN_POINT('Ctrl Pts',(1.8273599120008,-1.,0.764165902606056));
#30005=CARTESIAN_POINT('Ctrl Pts',(1.8273599120008,1.,0.764165902606056));
#30006=CARTESIAN_POINT('Ctrl Pts',(1.8334207722714,-1.,0.764602549687846));
#30007=CARTESIAN_POINT('Ctrl Pts',(1.8334207722714,1.,0.764602549687846));
#30008=CARTESIAN_POINT('Ctrl Pts',(1.83948181064823,-1.,0.764978057881688));
#30009=CARTESIAN_POINT('Ctrl Pts',(1.83948181064823,1.,0.764978057881688));
#30010=CARTESIAN_POINT('Ctrl Pts',(1.8455369887591,-1.,0.765291664861972));
#30011=CARTESIAN_POINT('Ctrl Pts',(1.8455369887591,1.,0.765291664861972));
#30012=CARTESIAN_POINT('Ctrl Pts',(1.85158945130054,-1.,0.765545710619023));
#30013=CARTESIAN_POINT('Ctrl Pts',(1.85158945130054,1.,0.765545710619023));
#30014=CARTESIAN_POINT('Ctrl Pts',(1.85764741390391,-1.,0.765744212909305));
#30015=CARTESIAN_POINT('Ctrl Pts',(1.85764741390391,1.,0.765744212909305));
#30016=CARTESIAN_POINT('Ctrl Pts',(1.86372027063314,-1.,0.765891519092557));
#30017=CARTESIAN_POINT('Ctrl Pts',(1.86372027063314,1.,0.765891519092557));
#30018=CARTESIAN_POINT('Ctrl Pts',(1.86981398314345,-1.,0.765990708546112));
#30019=CARTESIAN_POINT('Ctrl Pts',(1.86981398314345,1.,0.765990708546112));
#30020=CARTESIAN_POINT('Ctrl Pts',(1.87592888967886,-1.,0.766042837036759));
#30021=CARTESIAN_POINT('Ctrl Pts',(1.87592888967886,1.,0.766042837036759));
#30022=CARTESIAN_POINT('Ctrl Pts',(1.88206215302561,-1.,0.766047794851869));
#30023=CARTESIAN_POINT('Ctrl Pts',(1.88206215302561,1.,0.766047794851869));
#30024=CARTESIAN_POINT('Ctrl Pts',(1.88820926433409,-1.,0.76600483706209));
#30025=CARTESIAN_POINT('Ctrl Pts',(1.88820926433409,1.,0.76600483706209));
#30026=CARTESIAN_POINT('Ctrl Pts',(1.89436577771389,-1.,0.765913193856979));
#30027=CARTESIAN_POINT('Ctrl Pts',(1.89436577771389,1.,0.765913193856979));
#30028=CARTESIAN_POINT('Ctrl Pts',(1.90052930393599,-1.,0.765772772593395));
#30029=CARTESIAN_POINT('Ctrl Pts',(1.90052930393599,1.,0.765772772593395));
#30030=CARTESIAN_POINT('Ctrl Pts',(1.90669961402362,-1.,0.765584196937937));
#30031=CARTESIAN_POINT('Ctrl Pts',(1.90669961402362,1.,0.765584196937937));
#30032=CARTESIAN_POINT('Ctrl Pts',(1.91287765805174,-1.,0.765348465884739));
#30033=CARTESIAN_POINT('Ctrl Pts',(1.91287765805174,1.,0.765348465884739));
#30034=CARTESIAN_POINT('Ctrl Pts',(1.91906491634197,-1.,0.765066729667095));
#30035=CARTESIAN_POINT('Ctrl Pts',(1.91906491634197,1.,0.765066729667095));
#30036=CARTESIAN_POINT('Ctrl Pts',(1.92526263537041,-1.,0.764740025488189));
#30037=CARTESIAN_POINT('Ctrl Pts',(1.92526263537041,1.,0.764740025488189));
#30038=CARTESIAN_POINT('Ctrl Pts',(1.93147105496367,-1.,0.76436901067389));
#30039=CARTESIAN_POINT('Ctrl Pts',(1.93147105496367,1.,0.76436901067389));
#30040=CARTESIAN_POINT('Ctrl Pts',(1.93768964875867,-1.,0.763954049121394));
#30041=CARTESIAN_POINT('Ctrl Pts',(1.93768964875867,1.,0.763954049121394));
#30042=CARTESIAN_POINT('Ctrl Pts',(1.94391746617626,-1.,0.763495333538581));
#30043=CARTESIAN_POINT('Ctrl Pts',(1.94391746617626,1.,0.763495333538581));
#30044=CARTESIAN_POINT('Ctrl Pts',(1.95015342590025,-1.,0.762992990878774));
#30045=CARTESIAN_POINT('Ctrl Pts',(1.95015342590025,1.,0.762992990878774));
#30046=CARTESIAN_POINT('Ctrl Pts',(1.95639665309893,-1.,0.762447203806264));
#30047=CARTESIAN_POINT('Ctrl Pts',(1.95639665309893,1.,0.762447203806264));
#30048=CARTESIAN_POINT('Ctrl Pts',(1.96264672744229,-1.,0.761858300014575));
#30049=CARTESIAN_POINT('Ctrl Pts',(1.96264672744229,1.,0.761858300014575));
#30050=CARTESIAN_POINT('Ctrl Pts',(1.96890351582545,-1.,0.761226690483986));
#30051=CARTESIAN_POINT('Ctrl Pts',(1.96890351582545,1.,0.761226690483986));
#30052=CARTESIAN_POINT('Ctrl Pts',(1.97516705321521,-1.,0.760552825409856));
#30053=CARTESIAN_POINT('Ctrl Pts',(1.97516705321521,1.,0.760552825409856));
#30054=CARTESIAN_POINT('Ctrl Pts',(1.98143741418156,-1.,0.759837147452135));
#30055=CARTESIAN_POINT('Ctrl Pts',(1.98143741418156,1.,0.759837147452135));
#30056=CARTESIAN_POINT('Ctrl Pts',(1.98771456680806,-1.,0.759080037802243));
#30057=CARTESIAN_POINT('Ctrl Pts',(1.98771456680806,1.,0.759080037802243));
#30058=CARTESIAN_POINT('Ctrl Pts',(1.9939983109871,-1.,0.758281796766377));
#30059=CARTESIAN_POINT('Ctrl Pts',(1.9939983109871,1.,0.758281796766377));
#30060=CARTESIAN_POINT('Ctrl Pts',(2.00028834739072,-1.,0.757442676862342));
#30061=CARTESIAN_POINT('Ctrl Pts',(2.00028834739072,1.,0.757442676862342));
#30062=CARTESIAN_POINT('Ctrl Pts',(2.00658431587682,-1.,0.756562904646496));
#30063=CARTESIAN_POINT('Ctrl Pts',(2.00658431587682,1.,0.756562904646496));
#30064=CARTESIAN_POINT('Ctrl Pts',(2.01288584328149,-1.,0.755642704958101));
#30065=CARTESIAN_POINT('Ctrl Pts',(2.01288584328149,1.,0.755642704958101));
#30066=CARTESIAN_POINT('Ctrl Pts',(2.01919259406003,-1.,0.75468233072352));
#30067=CARTESIAN_POINT('Ctrl Pts',(2.01919259406003,1.,0.75468233072352));
#30068=CARTESIAN_POINT('Ctrl Pts',(2.02550428623587,-1.,0.753682061113766));
#30069=CARTESIAN_POINT('Ctrl Pts',(2.02550428623587,1.,0.753682061113766));
#30070=CARTESIAN_POINT('Ctrl Pts',(2.03182068456467,-1.,0.752642180488104));
#30071=CARTESIAN_POINT('Ctrl Pts',(2.03182068456467,1.,0.752642180488104));
#30072=CARTESIAN_POINT('Ctrl Pts',(2.03814160092173,-1.,0.751562963361384));
#30073=CARTESIAN_POINT('Ctrl Pts',(2.03814160092173,1.,0.751562963361384));
#30074=CARTESIAN_POINT('Ctrl Pts',(2.04446689147754,-1.,0.750444657874758));
#30075=CARTESIAN_POINT('Ctrl Pts',(2.04446689147754,1.,0.750444657874758));
#30076=CARTESIAN_POINT('Ctrl Pts',(2.05079645591606,-1.,0.749287468663053));
#30077=CARTESIAN_POINT('Ctrl Pts',(2.05079645591606,1.,0.749287468663053));
#30078=CARTESIAN_POINT('Ctrl Pts',(2.05713023030263,-1.,0.748091554181101));
#30079=CARTESIAN_POINT('Ctrl Pts',(2.05713023030263,1.,0.748091554181101));
#30080=CARTESIAN_POINT('Ctrl Pts',(2.06220058927162,-1.,0.747103932785504));
#30081=CARTESIAN_POINT('Ctrl Pts',(2.06220058927162,1.,0.747103932785504));
#30082=CARTESIAN_POINT('Ctrl Pts',(2.06600523016401,-1.,0.746345871542696));
#30083=CARTESIAN_POINT('Ctrl Pts',(2.06600523016401,1.,0.746345871542696));
#30084=CARTESIAN_POINT('Ctrl Pts',(2.06854248895575,-1.,0.74583279137781));
#30085=CARTESIAN_POINT('Ctrl Pts',(2.06854248895575,1.,0.74583279137781));
#30086=CARTESIAN_POINT('Ctrl Pts',(2.0698113262342,-1.,0.745574324794401));
#30087=CARTESIAN_POINT('Ctrl Pts',(2.0698113262342,1.,0.745574324794401));
#30088=CARTESIAN_POINT('',(1.60662857109684,1.,0.693717979106306));
#30089=CARTESIAN_POINT('Ctrl Pts',(1.60662857109684,1.,0.693717979106306));
#30090=CARTESIAN_POINT('Ctrl Pts',(1.61106790958151,1.,0.695712097881194));
#30091=CARTESIAN_POINT('Ctrl Pts',(1.61974673472612,1.,0.699605146405088));
#30092=CARTESIAN_POINT('Ctrl Pts',(1.63216541664676,1.,0.705159151988319));
#30093=CARTESIAN_POINT('Ctrl Pts',(1.64752408832016,1.,0.711993139355394));
#30094=CARTESIAN_POINT('Ctrl Pts',(1.6647288055568,1.,0.719585433804282));
#30095=CARTESIAN_POINT('Ctrl Pts',(1.67996158455503,1.,0.726235967997433));
#30096=CARTESIAN_POINT('Ctrl Pts',(1.69326921975743,1.,0.731963238697195));
#30097=CARTESIAN_POINT('Ctrl Pts',(1.70473309006121,1.,0.736799665724771));
#30098=CARTESIAN_POINT('Ctrl Pts',(1.71447789751927,1.,0.740795162032088));
#30099=CARTESIAN_POINT('Ctrl Pts',(1.7226822991693,1.,0.744021445433765));
#30100=CARTESIAN_POINT('Ctrl Pts',(1.72958533647399,1.,0.746574710096437));
#30101=CARTESIAN_POINT('Ctrl Pts',(1.73550351679848,1.,0.748582462954855));
#30102=CARTESIAN_POINT('Ctrl Pts',(1.74080458266705,1.,0.750193435979541));
#30103=CARTESIAN_POINT('Ctrl Pts',(1.74585086852298,1.,0.751555614163629));
#30104=CARTESIAN_POINT('Ctrl Pts',(1.75095139468809,1.,0.752797683531377));
#30105=CARTESIAN_POINT('Ctrl Pts',(1.75631083600175,1.,0.75400925402848));
#30106=CARTESIAN_POINT('Ctrl Pts',(1.7619781724032,1.,0.755220979975262));
#30107=CARTESIAN_POINT('Ctrl Pts',(1.76789396003141,1.,0.756421896028403));
#30108=CARTESIAN_POINT('Ctrl Pts',(1.77394167108342,1.,0.757578264077238));
#30109=CARTESIAN_POINT('Ctrl Pts',(1.77999411220912,1.,0.75865062667738));
#30110=CARTESIAN_POINT('Ctrl Pts',(1.78596964884526,1.,0.759614401109868));
#30111=CARTESIAN_POINT('Ctrl Pts',(1.79185815610802,1.,0.760469555880425));
#30112=CARTESIAN_POINT('Ctrl Pts',(1.79768986997735,1.,0.761229695230359));
#30113=CARTESIAN_POINT('Ctrl Pts',(1.80351583877334,1.,0.761915336443516));
#30114=CARTESIAN_POINT('Ctrl Pts',(1.80938551463989,1.,0.762546129464036));
#30115=CARTESIAN_POINT('Ctrl Pts',(1.81532118405566,1.,0.763132003836783));
#30116=CARTESIAN_POINT('Ctrl Pts',(1.82131873145297,1.,0.763673465462854));
#30117=CARTESIAN_POINT('Ctrl Pts',(1.8273599120008,1.,0.764165902606056));
#30118=CARTESIAN_POINT('Ctrl Pts',(1.8334207722714,1.,0.764602549687846));
#30119=CARTESIAN_POINT('Ctrl Pts',(1.83948181064823,1.,0.764978057881688));
#30120=CARTESIAN_POINT('Ctrl Pts',(1.8455369887591,1.,0.765291664861972));
#30121=CARTESIAN_POINT('Ctrl Pts',(1.85158945130054,1.,0.765545710619023));
#30122=CARTESIAN_POINT('Ctrl Pts',(1.85764741390391,1.,0.765744212909305));
#30123=CARTESIAN_POINT('Ctrl Pts',(1.86372027063314,1.,0.765891519092557));
#30124=CARTESIAN_POINT('Ctrl Pts',(1.86981398314345,1.,0.765990708546112));
#30125=CARTESIAN_POINT('Ctrl Pts',(1.87592888967886,1.,0.766042837036759));
#30126=CARTESIAN_POINT('Ctrl Pts',(1.88206215302561,1.,0.766047794851869));
#30127=CARTESIAN_POINT('Ctrl Pts',(1.88820926433409,1.,0.76600483706209));
#30128=CARTESIAN_POINT('Ctrl Pts',(1.89436577771389,1.,0.765913193856979));
#30129=CARTESIAN_POINT('Ctrl Pts',(1.90052930393599,1.,0.765772772593395));
#30130=CARTESIAN_POINT('Ctrl Pts',(1.90669961402362,1.,0.765584196937937));
#30131=CARTESIAN_POINT('Ctrl Pts',(1.91287765805174,1.,0.765348465884739));
#30132=CARTESIAN_POINT('Ctrl Pts',(1.91906491634197,1.,0.765066729667095));
#30133=CARTESIAN_POINT('Ctrl Pts',(1.92526263537041,1.,0.764740025488189));
#30134=CARTESIAN_POINT('Ctrl Pts',(1.93147105496367,1.,0.76436901067389));
#30135=CARTESIAN_POINT('Ctrl Pts',(1.93768964875867,1.,0.763954049121394));
#30136=CARTESIAN_POINT('Ctrl Pts',(1.94391746617626,1.,0.763495333538581));
#30137=CARTESIAN_POINT('Ctrl Pts',(1.95015342590025,1.,0.762992990878774));
#30138=CARTESIAN_POINT('Ctrl Pts',(1.95639665309893,1.,0.762447203806264));
#30139=CARTESIAN_POINT('Ctrl Pts',(1.96264672744229,1.,0.761858300014575));
#30140=CARTESIAN_POINT('Ctrl Pts',(1.96890351582545,1.,0.761226690483986));
#30141=CARTESIAN_POINT('Ctrl Pts',(1.97516705321521,1.,0.760552825409856));
#30142=CARTESIAN_POINT('Ctrl Pts',(1.98143741418156,1.,0.759837147452135));
#30143=CARTESIAN_POINT('Ctrl Pts',(1.98771456680806,1.,0.759080037802243));
#30144=CARTESIAN_POINT('Ctrl Pts',(1.9939983109871,1.,0.758281796766377));
#30145=CARTESIAN_POINT('Ctrl Pts',(2.00028834739072,1.,0.757442676862342));
#30146=CARTESIAN_POINT('Ctrl Pts',(2.00658431587682,1.,0.756562904646496));
#30147=CARTESIAN_POINT('Ctrl Pts',(2.01288584328149,1.,0.755642704958101));
#30148=CARTESIAN_POINT('Ctrl Pts',(2.01919259406003,1.,0.75468233072352));
#30149=CARTESIAN_POINT('Ctrl Pts',(2.02550428623587,1.,0.753682061113766));
#30150=CARTESIAN_POINT('Ctrl Pts',(2.03182068456467,1.,0.752642180488104));
#30151=CARTESIAN_POINT('Ctrl Pts',(2.03814160092173,1.,0.751562963361384));
#30152=CARTESIAN_POINT('Ctrl Pts',(2.04446689147754,1.,0.750444657874758));
#30153=CARTESIAN_POINT('Ctrl Pts',(2.05079645591606,1.,0.749287468663053));
#30154=CARTESIAN_POINT('Ctrl Pts',(2.05713023030263,1.,0.748091554181101));
#30155=CARTESIAN_POINT('Ctrl Pts',(2.06220058927162,1.,0.747103932785504));
#30156=CARTESIAN_POINT('Ctrl Pts',(2.06600523016401,1.,0.746345871542696));
#30157=CARTESIAN_POINT('Ctrl Pts',(2.06854248895575,1.,0.74583279137781));
#30158=CARTESIAN_POINT('Ctrl Pts',(2.0698113262342,1.,0.745574324794401));
#30159=CARTESIAN_POINT('',(1.60662857109684,0.,0.693717979106305));
#30160=CARTESIAN_POINT('Origin',(0.,0.,0.));
#30161=CARTESIAN_POINT('',(1.5055822144029,1.,0.892032620296856));
#30162=CARTESIAN_POINT('Origin',(0.,1.,0.));
#30163=CARTESIAN_POINT('',(1.5055822144029,0.,0.892032620296855));
#30164=CARTESIAN_POINT('Ctrl Pts',(1.81978687191668,-1.,1.23627494547115));
#30165=CARTESIAN_POINT('Ctrl Pts',(1.81978687191668,1.,1.23627494547115));
#30166=CARTESIAN_POINT('Ctrl Pts',(1.81925017193666,-1.,1.23509651170476));
#30167=CARTESIAN_POINT('Ctrl Pts',(1.81925017193666,1.,1.23509651170476));
#30168=CARTESIAN_POINT('Ctrl Pts',(1.81817389921279,-1.,1.2327422452705));
#30169=CARTESIAN_POINT('Ctrl Pts',(1.81817389921279,1.,1.2327422452705));
#30170=CARTESIAN_POINT('Ctrl Pts',(1.8165508718364,-1.,1.2292186489137));
#30171=CARTESIAN_POINT('Ctrl Pts',(1.8165508718364,1.,1.2292186489137));
#30172=CARTESIAN_POINT('Ctrl Pts',(1.81436959210434,-1.,1.2245361330495));
#30173=CARTESIAN_POINT('Ctrl Pts',(1.81436959210434,1.,1.2245361330495));
#30174=CARTESIAN_POINT('Ctrl Pts',(1.81161420806656,-1.,1.21870906103557));
#30175=CARTESIAN_POINT('Ctrl Pts',(1.81161420806656,1.,1.21870906103557));
#30176=CARTESIAN_POINT('Ctrl Pts',(1.80882996917129,-1.,1.21290815708314));
#30177=CARTESIAN_POINT('Ctrl Pts',(1.80882996917129,1.,1.21290815708314));
#30178=CARTESIAN_POINT('Ctrl Pts',(1.80601678480707,-1.,1.20713356605475));
#30179=CARTESIAN_POINT('Ctrl Pts',(1.80601678480707,1.,1.20713356605475));
#30180=CARTESIAN_POINT('Ctrl Pts',(1.80317454838603,-1.,1.20138548938974));
#30181=CARTESIAN_POINT('Ctrl Pts',(1.80317454838603,1.,1.20138548938974));
#30182=CARTESIAN_POINT('Ctrl Pts',(1.80030314369879,-1.,1.19566418930242));
#30183=CARTESIAN_POINT('Ctrl Pts',(1.80030314369879,1.,1.19566418930242));
#30184=CARTESIAN_POINT('Ctrl Pts',(1.79740245923478,-1.,1.18996997934445));
#30185=CARTESIAN_POINT('Ctrl Pts',(1.79740245923478,1.,1.18996997934445));
#30186=CARTESIAN_POINT('Ctrl Pts',(1.79447240321515,-1.,1.18430321697432));
#30187=CARTESIAN_POINT('Ctrl Pts',(1.79447240321515,1.,1.18430321697432));
#30188=CARTESIAN_POINT('Ctrl Pts',(1.79151291552689,-1.,1.17866429440809));
#30189=CARTESIAN_POINT('Ctrl Pts',(1.79151291552689,1.,1.17866429440809));
#30190=CARTESIAN_POINT('Ctrl Pts',(1.78852398877616,-1.,1.17305363177328));
#30191=CARTESIAN_POINT('Ctrl Pts',(1.78852398877616,1.,1.17305363177328));
#30192=CARTESIAN_POINT('Ctrl Pts',(1.78550566040443,-1.,1.16747166312303));
#30193=CARTESIAN_POINT('Ctrl Pts',(1.78550566040443,1.,1.16747166312303));
#30194=CARTESIAN_POINT('Ctrl Pts',(1.78245795881009,-1.,1.16191881298499));
#30195=CARTESIAN_POINT('Ctrl Pts',(1.78245795881009,1.,1.16191881298499));
#30196=CARTESIAN_POINT('Ctrl Pts',(1.77938085564275,-1.,1.15639547194698));
#30197=CARTESIAN_POINT('Ctrl Pts',(1.77938085564275,1.,1.15639547194698));
#30198=CARTESIAN_POINT('Ctrl Pts',(1.7762742255701,-1.,1.15090197841515));
#30199=CARTESIAN_POINT('Ctrl Pts',(1.7762742255701,1.,1.15090197841515));
#30200=CARTESIAN_POINT('Ctrl Pts',(1.77313777896194,-1.,1.1454385822692));
#30201=CARTESIAN_POINT('Ctrl Pts',(1.77313777896194,1.,1.1454385822692));
#30202=CARTESIAN_POINT('Ctrl Pts',(1.76997111386769,-1.,1.14000548336975));
#30203=CARTESIAN_POINT('Ctrl Pts',(1.76997111386769,1.,1.14000548336975));
#30204=CARTESIAN_POINT('Ctrl Pts',(1.76677384551862,-1.,1.1346029180462));
#30205=CARTESIAN_POINT('Ctrl Pts',(1.76677384551862,1.,1.1346029180462));
#30206=CARTESIAN_POINT('Ctrl Pts',(1.7635457196617,-1.,1.12923123555075));
#30207=CARTESIAN_POINT('Ctrl Pts',(1.7635457196617,1.,1.12923123555075));
#30208=CARTESIAN_POINT('Ctrl Pts',(1.76028671825096,-1.,1.12389096855086));
#30209=CARTESIAN_POINT('Ctrl Pts',(1.76028671825096,1.,1.12389096855086));
#30210=CARTESIAN_POINT('Ctrl Pts',(1.75699720772105,-1.,1.11858293216763));
#30211=CARTESIAN_POINT('Ctrl Pts',(1.75699720772105,1.,1.11858293216763));
#30212=CARTESIAN_POINT('Ctrl Pts',(1.7536777209463,-1.,1.11330807582551));
#30213=CARTESIAN_POINT('Ctrl Pts',(1.7536777209463,1.,1.11330807582551));
#30214=CARTESIAN_POINT('Ctrl Pts',(1.7503286607592,-1.,1.10806728183007));
#30215=CARTESIAN_POINT('Ctrl Pts',(1.7503286607592,1.,1.10806728183007));
#30216=CARTESIAN_POINT('Ctrl Pts',(1.74695004214923,-1.,1.10286118991143));
#30217=CARTESIAN_POINT('Ctrl Pts',(1.74695004214923,1.,1.10286118991143));
#30218=CARTESIAN_POINT('Ctrl Pts',(1.74354119236208,-1.,1.09768999241226));
#30219=CARTESIAN_POINT('Ctrl Pts',(1.74354119236208,1.,1.09768999241226));
#30220=CARTESIAN_POINT('Ctrl Pts',(1.74010053962247,-1.,1.09255329056493));
#30221=CARTESIAN_POINT('Ctrl Pts',(1.74010053962247,1.,1.09255329056493));
#30222=CARTESIAN_POINT('Ctrl Pts',(1.73662628326091,-1.,1.08745056285427));
#30223=CARTESIAN_POINT('Ctrl Pts',(1.73662628326091,1.,1.08745056285427));
#30224=CARTESIAN_POINT('Ctrl Pts',(1.73311705663407,-1.,1.08238162784749));
#30225=CARTESIAN_POINT('Ctrl Pts',(1.73311705663407,1.,1.08238162784749));
#30226=CARTESIAN_POINT('Ctrl Pts',(1.72957248977424,-1.,1.0773470373727));
#30227=CARTESIAN_POINT('Ctrl Pts',(1.72957248977424,1.,1.0773470373727));
#30228=CARTESIAN_POINT('Ctrl Pts',(1.72599406198488,-1.,1.07234866990252));
#30229=CARTESIAN_POINT('Ctrl Pts',(1.72599406198488,1.,1.07234866990252));
#30230=CARTESIAN_POINT('Ctrl Pts',(1.72238500928453,-1.,1.06738966975462));
#30231=CARTESIAN_POINT('Ctrl Pts',(1.72238500928453,1.,1.06738966975462));
#30232=CARTESIAN_POINT('Ctrl Pts',(1.71874858456904,-1.,1.06247324680647));
#30233=CARTESIAN_POINT('Ctrl Pts',(1.71874858456904,1.,1.06247324680647));
#30234=CARTESIAN_POINT('Ctrl Pts',(1.7150865442702,-1.,1.05760163192479));
#30235=CARTESIAN_POINT('Ctrl Pts',(1.7150865442702,1.,1.05760163192479));
#30236=CARTESIAN_POINT('Ctrl Pts',(1.71139783543989,-1.,1.05277517202855));
#30237=CARTESIAN_POINT('Ctrl Pts',(1.71139783543989,1.,1.05277517202855));
#30238=CARTESIAN_POINT('Ctrl Pts',(1.70767646263649,-1.,1.04799085404995));
#30239=CARTESIAN_POINT('Ctrl Pts',(1.70767646263649,1.,1.04799085404995));
#30240=CARTESIAN_POINT('Ctrl Pts',(1.70391338707982,-1.,1.04324363334554));
#30241=CARTESIAN_POINT('Ctrl Pts',(1.70391338707982,1.,1.04324363334554));
#30242=CARTESIAN_POINT('Ctrl Pts',(1.70010052930962,-1.,1.03852922490789));
#30243=CARTESIAN_POINT('Ctrl Pts',(1.70010052930962,1.,1.03852922490789));
#30244=CARTESIAN_POINT('Ctrl Pts',(1.69623414782771,-1.,1.03384646003588));
#30245=CARTESIAN_POINT('Ctrl Pts',(1.69623414782771,1.,1.03384646003588));
#30246=CARTESIAN_POINT('Ctrl Pts',(1.69231840863458,-1.,1.02919977579147));
#30247=CARTESIAN_POINT('Ctrl Pts',(1.69231840863458,1.,1.02919977579147));
#30248=CARTESIAN_POINT('Ctrl Pts',(1.68836910178447,-1.,1.02460180535255));
#30249=CARTESIAN_POINT('Ctrl Pts',(1.68836910178447,1.,1.02460180535255));
#30250=CARTESIAN_POINT('Ctrl Pts',(1.68440578021706,-1.,1.02006795074201));
#30251=CARTESIAN_POINT('Ctrl Pts',(1.68440578021706,1.,1.02006795074201));
#30252=CARTESIAN_POINT('Ctrl Pts',(1.68044289894798,-1.,1.01561026162773));
#30253=CARTESIAN_POINT('Ctrl Pts',(1.68044289894798,1.,1.01561026162773));
#30254=CARTESIAN_POINT('Ctrl Pts',(1.67648246776464,-1.,1.01123236493511));
#30255=CARTESIAN_POINT('Ctrl Pts',(1.67648246776464,1.,1.01123236493511));
#30256=CARTESIAN_POINT('Ctrl Pts',(1.67250335383293,-1.,1.00692206696414));
#30257=CARTESIAN_POINT('Ctrl Pts',(1.67250335383293,1.,1.00692206696414));
#30258=CARTESIAN_POINT('Ctrl Pts',(1.66846059277303,-1.,1.00265091003727));
#30259=CARTESIAN_POINT('Ctrl Pts',(1.66846059277303,1.,1.00265091003727));
#30260=CARTESIAN_POINT('Ctrl Pts',(1.66430758030376,-1.,0.998389654952758));
#30261=CARTESIAN_POINT('Ctrl Pts',(1.66430758030376,1.,0.998389654952758));
#30262=CARTESIAN_POINT('Ctrl Pts',(1.66001553809947,-1.,0.994121836661306));
#30263=CARTESIAN_POINT('Ctrl Pts',(1.66001553809947,1.,0.994121836661306));
#30264=CARTESIAN_POINT('Ctrl Pts',(1.65559044289699,-1.,0.989855627854165));
#30265=CARTESIAN_POINT('Ctrl Pts',(1.65559044289699,1.,0.989855627854165));
#30266=CARTESIAN_POINT('Ctrl Pts',(1.65110016612638,-1.,0.985642622920821));
#30267=CARTESIAN_POINT('Ctrl Pts',(1.65110016612638,1.,0.985642622920821));
#30268=CARTESIAN_POINT('Ctrl Pts',(1.64665139190656,-1.,0.981562530939489));
#30269=CARTESIAN_POINT('Ctrl Pts',(1.64665139190656,1.,0.981562530939489));
#30270=CARTESIAN_POINT('Ctrl Pts',(1.64233990826687,-1.,0.977689794119417));
#30271=CARTESIAN_POINT('Ctrl Pts',(1.64233990826687,1.,0.977689794119417));
#30272=CARTESIAN_POINT('Ctrl Pts',(1.63820952658144,-1.,0.974066058287419));
#30273=CARTESIAN_POINT('Ctrl Pts',(1.63820952658144,1.,0.974066058287419));
#30274=CARTESIAN_POINT('Ctrl Pts',(1.63420665729798,-1.,0.970669715997509));
#30275=CARTESIAN_POINT('Ctrl Pts',(1.63420665729798,1.,0.970669715997509));
#30276=CARTESIAN_POINT('Ctrl Pts',(1.63013849959461,-1.,0.967387853230345));
#30277=CARTESIAN_POINT('Ctrl Pts',(1.63013849959461,1.,0.967387853230345));
#30278=CARTESIAN_POINT('Ctrl Pts',(1.62571930670187,-1.,0.964046107040536));
#30279=CARTESIAN_POINT('Ctrl Pts',(1.62571930670187,1.,0.964046107040536));
#30280=CARTESIAN_POINT('Ctrl Pts',(1.62061638140221,-1.,0.960438326101729));
#30281=CARTESIAN_POINT('Ctrl Pts',(1.62061638140221,1.,0.960438326101729));
#30282=CARTESIAN_POINT('Ctrl Pts',(1.61449324337085,-1.,0.956354422920671));
#30283=CARTESIAN_POINT('Ctrl Pts',(1.61449324337085,1.,0.956354422920671));
#30284=CARTESIAN_POINT('Ctrl Pts',(1.60706069896936,-1.,0.951613284356035));
#30285=CARTESIAN_POINT('Ctrl Pts',(1.60706069896936,1.,0.951613284356035));
#30286=CARTESIAN_POINT('Ctrl Pts',(1.59810042043673,-1.,0.946078063315257));
#30287=CARTESIAN_POINT('Ctrl Pts',(1.59810042043673,1.,0.946078063315257));
#30288=CARTESIAN_POINT('Ctrl Pts',(1.58744937487176,-1.,0.939646377893399));
#30289=CARTESIAN_POINT('Ctrl Pts',(1.58744937487176,1.,0.939646377893399));
#30290=CARTESIAN_POINT('Ctrl Pts',(1.57499388382243,-1.,0.932246680108685));
#30291=CARTESIAN_POINT('Ctrl Pts',(1.57499388382243,1.,0.932246680108685));
#30292=CARTESIAN_POINT('Ctrl Pts',(1.56065988578893,-1.,0.923832188944341));
#30293=CARTESIAN_POINT('Ctrl Pts',(1.56065988578893,1.,0.923832188944341));
#30294=CARTESIAN_POINT('Ctrl Pts',(1.54440491149498,-1.,0.914375919026456));
#30295=CARTESIAN_POINT('Ctrl Pts',(1.54440491149498,1.,0.914375919026456));
#30296=CARTESIAN_POINT('Ctrl Pts',(1.52984849887993,-1.,0.905967409625651));
#30297=CARTESIAN_POINT('Ctrl Pts',(1.52984849887993,1.,0.905967409625651));
#30298=CARTESIAN_POINT('Ctrl Pts',(1.51805569590094,-1.,0.899185047483511));
#30299=CARTESIAN_POINT('Ctrl Pts',(1.51805569590094,1.,0.899185047483511));
#30300=CARTESIAN_POINT('Ctrl Pts',(1.50980486806688,-1.,0.894452006964544));
#30301=CARTESIAN_POINT('Ctrl Pts',(1.50980486806688,1.,0.894452006964544));
#30302=CARTESIAN_POINT('Ctrl Pts',(1.5055822144029,-1.,0.892032620296856));
#30303=CARTESIAN_POINT('Ctrl Pts',(1.5055822144029,1.,0.892032620296856));
#30304=CARTESIAN_POINT('',(1.81978687191668,1.,1.23627494547115));
#30305=CARTESIAN_POINT('Ctrl Pts',(1.81978687191668,1.,1.23627494547115));
#30306=CARTESIAN_POINT('Ctrl Pts',(1.81925017193666,1.,1.23509651170476));
#30307=CARTESIAN_POINT('Ctrl Pts',(1.81817389921279,1.,1.2327422452705));
#30308=CARTESIAN_POINT('Ctrl Pts',(1.8165508718364,1.,1.2292186489137));
#30309=CARTESIAN_POINT('Ctrl Pts',(1.81436959210434,1.,1.2245361330495));
#30310=CARTESIAN_POINT('Ctrl Pts',(1.81161420806656,1.,1.21870906103557));
#30311=CARTESIAN_POINT('Ctrl Pts',(1.80882996917129,1.,1.21290815708314));
#30312=CARTESIAN_POINT('Ctrl Pts',(1.80601678480707,1.,1.20713356605475));
#30313=CARTESIAN_POINT('Ctrl Pts',(1.80317454838603,1.,1.20138548938974));
#30314=CARTESIAN_POINT('Ctrl Pts',(1.80030314369879,1.,1.19566418930242));
#30315=CARTESIAN_POINT('Ctrl Pts',(1.79740245923478,1.,1.18996997934445));
#30316=CARTESIAN_POINT('Ctrl Pts',(1.79447240321515,1.,1.18430321697432));
#30317=CARTESIAN_POINT('Ctrl Pts',(1.79151291552689,1.,1.17866429440809));
#30318=CARTESIAN_POINT('Ctrl Pts',(1.78852398877616,1.,1.17305363177328));
#30319=CARTESIAN_POINT('Ctrl Pts',(1.78550566040443,1.,1.16747166312303));
#30320=CARTESIAN_POINT('Ctrl Pts',(1.78245795881009,1.,1.16191881298499));
#30321=CARTESIAN_POINT('Ctrl Pts',(1.77938085564275,1.,1.15639547194698));
#30322=CARTESIAN_POINT('Ctrl Pts',(1.7762742255701,1.,1.15090197841515));
#30323=CARTESIAN_POINT('Ctrl Pts',(1.77313777896194,1.,1.1454385822692));
#30324=CARTESIAN_POINT('Ctrl Pts',(1.76997111386769,1.,1.14000548336975));
#30325=CARTESIAN_POINT('Ctrl Pts',(1.76677384551862,1.,1.1346029180462));
#30326=CARTESIAN_POINT('Ctrl Pts',(1.7635457196617,1.,1.12923123555075));
#30327=CARTESIAN_POINT('Ctrl Pts',(1.76028671825096,1.,1.12389096855086));
#30328=CARTESIAN_POINT('Ctrl Pts',(1.75699720772105,1.,1.11858293216763));
#30329=CARTESIAN_POINT('Ctrl Pts',(1.7536777209463,1.,1.11330807582551));
#30330=CARTESIAN_POINT('Ctrl Pts',(1.7503286607592,1.,1.10806728183007));
#30331=CARTESIAN_POINT('Ctrl Pts',(1.74695004214923,1.,1.10286118991143));
#30332=CARTESIAN_POINT('Ctrl Pts',(1.74354119236208,1.,1.09768999241226));
#30333=CARTESIAN_POINT('Ctrl Pts',(1.74010053962247,1.,1.09255329056493));
#30334=CARTESIAN_POINT('Ctrl Pts',(1.73662628326091,1.,1.08745056285427));
#30335=CARTESIAN_POINT('Ctrl Pts',(1.73311705663407,1.,1.08238162784749));
#30336=CARTESIAN_POINT('Ctrl Pts',(1.72957248977424,1.,1.0773470373727));
#30337=CARTESIAN_POINT('Ctrl Pts',(1.72599406198488,1.,1.07234866990252));
#30338=CARTESIAN_POINT('Ctrl Pts',(1.72238500928453,1.,1.06738966975462));
#30339=CARTESIAN_POINT('Ctrl Pts',(1.71874858456904,1.,1.06247324680647));
#30340=CARTESIAN_POINT('Ctrl Pts',(1.7150865442702,1.,1.05760163192479));
#30341=CARTESIAN_POINT('Ctrl Pts',(1.71139783543989,1.,1.05277517202855));
#30342=CARTESIAN_POINT('Ctrl Pts',(1.70767646263649,1.,1.04799085404995));
#30343=CARTESIAN_POINT('Ctrl Pts',(1.70391338707982,1.,1.04324363334554));
#30344=CARTESIAN_POINT('Ctrl Pts',(1.70010052930962,1.,1.03852922490789));
#30345=CARTESIAN_POINT('Ctrl Pts',(1.69623414782771,1.,1.03384646003588));
#30346=CARTESIAN_POINT('Ctrl Pts',(1.69231840863458,1.,1.02919977579147));
#30347=CARTESIAN_POINT('Ctrl Pts',(1.68836910178447,1.,1.02460180535255));
#30348=CARTESIAN_POINT('Ctrl Pts',(1.68440578021706,1.,1.02006795074201));
#30349=CARTESIAN_POINT('Ctrl Pts',(1.68044289894798,1.,1.01561026162773));
#30350=CARTESIAN_POINT('Ctrl Pts',(1.67648246776464,1.,1.01123236493511));
#30351=CARTESIAN_POINT('Ctrl Pts',(1.67250335383293,1.,1.00692206696414));
#30352=CARTESIAN_POINT('Ctrl Pts',(1.66846059277303,1.,1.00265091003727));
#30353=CARTESIAN_POINT('Ctrl Pts',(1.66430758030376,1.,0.998389654952758));
#30354=CARTESIAN_POINT('Ctrl Pts',(1.66001553809947,1.,0.994121836661306));
#30355=CARTESIAN_POINT('Ctrl Pts',(1.65559044289699,1.,0.989855627854165));
#30356=CARTESIAN_POINT('Ctrl Pts',(1.65110016612638,1.,0.985642622920821));
#30357=CARTESIAN_POINT('Ctrl Pts',(1.64665139190656,1.,0.981562530939489));
#30358=CARTESIAN_POINT('Ctrl Pts',(1.64233990826687,1.,0.977689794119417));
#30359=CARTESIAN_POINT('Ctrl Pts',(1.63820952658144,1.,0.974066058287419));
#30360=CARTESIAN_POINT('Ctrl Pts',(1.63420665729798,1.,0.970669715997509));
#30361=CARTESIAN_POINT('Ctrl Pts',(1.63013849959461,1.,0.967387853230345));
#30362=CARTESIAN_POINT('Ctrl Pts',(1.62571930670187,1.,0.964046107040536));
#30363=CARTESIAN_POINT('Ctrl Pts',(1.62061638140221,1.,0.960438326101729));
#30364=CARTESIAN_POINT('Ctrl Pts',(1.61449324337085,1.,0.956354422920671));
#30365=CARTESIAN_POINT('Ctrl Pts',(1.60706069896936,1.,0.951613284356035));
#30366=CARTESIAN_POINT('Ctrl Pts',(1.59810042043673,1.,0.946078063315257));
#30367=CARTESIAN_POINT('Ctrl Pts',(1.58744937487176,1.,0.939646377893399));
#30368=CARTESIAN_POINT('Ctrl Pts',(1.57499388382243,1.,0.932246680108685));
#30369=CARTESIAN_POINT('Ctrl Pts',(1.56065988578893,1.,0.923832188944341));
#30370=CARTESIAN_POINT('Ctrl Pts',(1.54440491149498,1.,0.914375919026456));
#30371=CARTESIAN_POINT('Ctrl Pts',(1.52984849887993,1.,0.905967409625651));
#30372=CARTESIAN_POINT('Ctrl Pts',(1.51805569590094,1.,0.899185047483511));
#30373=CARTESIAN_POINT('Ctrl Pts',(1.50980486806688,1.,0.894452006964544));
#30374=CARTESIAN_POINT('Ctrl Pts',(1.5055822144029,1.,0.892032620296856));
#30375=CARTESIAN_POINT('',(1.81978687191668,0.,1.23627494547115));
#30376=CARTESIAN_POINT('Origin',(1.73811241238545,0.,1.34869019493419));
#30377=CARTESIAN_POINT('',(1.73811241238545,1.,1.34869019493419));
#30378=CARTESIAN_POINT('',(1.81978687191668,1.,1.23627494547115));
#30379=CARTESIAN_POINT('',(1.73811241238545,0.,1.34869019493419));
#30380=CARTESIAN_POINT('Ctrl Pts',(1.31362392696032,-1.,1.15624053661742));
#30381=CARTESIAN_POINT('Ctrl Pts',(1.31362392696032,1.,1.15624053661742));
#30382=CARTESIAN_POINT('Ctrl Pts',(1.31722977216397,-1.,1.15950888730809));
#30383=CARTESIAN_POINT('Ctrl Pts',(1.31722977216397,1.,1.15950888730809));
#30384=CARTESIAN_POINT('Ctrl Pts',(1.32428080721772,-1.,1.16589330093588));
#30385=CARTESIAN_POINT('Ctrl Pts',(1.32428080721772,1.,1.16589330093588));
#30386=CARTESIAN_POINT('Ctrl Pts',(1.33437539347008,-1.,1.17501305789857));
#30387=CARTESIAN_POINT('Ctrl Pts',(1.33437539347008,1.,1.17501305789857));
#30388=CARTESIAN_POINT('Ctrl Pts',(1.34687054001093,-1.,1.18625865667441));
#30389=CARTESIAN_POINT('Ctrl Pts',(1.34687054001093,1.,1.18625865667441));
#30390=CARTESIAN_POINT('Ctrl Pts',(1.36088705043885,-1.,1.1987959077932));
#30391=CARTESIAN_POINT('Ctrl Pts',(1.36088705043885,1.,1.1987959077932));
#30392=CARTESIAN_POINT('Ctrl Pts',(1.37331915607905,-1.,1.20982812925645));
#30393=CARTESIAN_POINT('Ctrl Pts',(1.37331915607905,1.,1.20982812925645));
#30394=CARTESIAN_POINT('Ctrl Pts',(1.38420564527715,-1.,1.21938737280852));
#30395=CARTESIAN_POINT('Ctrl Pts',(1.38420564527715,1.,1.21938737280852));
#30396=CARTESIAN_POINT('Ctrl Pts',(1.39361389568796,-1.,1.22752961899387));
#30397=CARTESIAN_POINT('Ctrl Pts',(1.39361389568796,1.,1.22752961899387));
#30398=CARTESIAN_POINT('Ctrl Pts',(1.40164708206106,-1.,1.23434087290423));
#30399=CARTESIAN_POINT('Ctrl Pts',(1.40164708206106,1.,1.23434087290423));
#30400=CARTESIAN_POINT('Ctrl Pts',(1.40845295531283,-1.,1.23994455029534));
#30401=CARTESIAN_POINT('Ctrl Pts',(1.40845295531283,1.,1.23994455029534));
#30402=CARTESIAN_POINT('Ctrl Pts',(1.41422913175179,-1.,1.24450600513056));
#30403=CARTESIAN_POINT('Ctrl Pts',(1.41422913175179,1.,1.24450600513056));
#30404=CARTESIAN_POINT('Ctrl Pts',(1.41923722596025,-1.,1.24824430986571));
#30405=CARTESIAN_POINT('Ctrl Pts',(1.41923722596025,1.,1.24824430986571));
#30406=CARTESIAN_POINT('Ctrl Pts',(1.42378102115575,-1.,1.2514145557001));
#30407=CARTESIAN_POINT('Ctrl Pts',(1.42378102115575,1.,1.2514145557001));
#30408=CARTESIAN_POINT('Ctrl Pts',(1.42815938799387,-1.,1.25426945222639));
#30409=CARTESIAN_POINT('Ctrl Pts',(1.42815938799387,1.,1.25426945222639));
#30410=CARTESIAN_POINT('Ctrl Pts',(1.43262645609691,-1.,1.25702687965755));
#30411=CARTESIAN_POINT('Ctrl Pts',(1.43262645609691,1.,1.25702687965755));
#30412=CARTESIAN_POINT('Ctrl Pts',(1.43734919180847,-1.,1.25983531012005));
#30413=CARTESIAN_POINT('Ctrl Pts',(1.43734919180847,1.,1.25983531012005));
#30414=CARTESIAN_POINT('Ctrl Pts',(1.44236470511303,-1.,1.26273903323859));
#30415=CARTESIAN_POINT('Ctrl Pts',(1.44236470511303,1.,1.26273903323859));
#30416=CARTESIAN_POINT('Ctrl Pts',(1.44761985001662,-1.,1.26570925118868));
#30417=CARTESIAN_POINT('Ctrl Pts',(1.44761985001662,1.,1.26570925118868));
#30418=CARTESIAN_POINT('Ctrl Pts',(1.45301422764247,-1.,1.2686778680489));
#30419=CARTESIAN_POINT('Ctrl Pts',(1.45301422764247,1.,1.2686778680489));
#30420=CARTESIAN_POINT('Ctrl Pts',(1.45843906294697,-1.,1.27156805265289));
#30421=CARTESIAN_POINT('Ctrl Pts',(1.45843906294697,1.,1.27156805265289));
#30422=CARTESIAN_POINT('Ctrl Pts',(1.46382431332476,-1.,1.27433119897822));
#30423=CARTESIAN_POINT('Ctrl Pts',(1.46382431332476,1.,1.27433119897822));
#30424=CARTESIAN_POINT('Ctrl Pts',(1.46916035917133,-1.,1.2769641483109));
#30425=CARTESIAN_POINT('Ctrl Pts',(1.46916035917133,1.,1.2769641483109));
#30426=CARTESIAN_POINT('Ctrl Pts',(1.4744717526707,-1.,1.2794891824849));
#30427=CARTESIAN_POINT('Ctrl Pts',(1.4744717526707,1.,1.2794891824849));
#30428=CARTESIAN_POINT('Ctrl Pts',(1.47980070347095,-1.,1.28194158939517));
#30429=CARTESIAN_POINT('Ctrl Pts',(1.47980070347095,1.,1.28194158939517));
#30430=CARTESIAN_POINT('Ctrl Pts',(1.4851881711891,-1.,1.28435533880201));
#30431=CARTESIAN_POINT('Ctrl Pts',(1.4851881711891,1.,1.28435533880201));
#30432=CARTESIAN_POINT('Ctrl Pts',(1.4906522831278,-1.,1.2867467611644));
#30433=CARTESIAN_POINT('Ctrl Pts',(1.4906522831278,1.,1.2867467611644));
#30434=CARTESIAN_POINT('Ctrl Pts',(1.49618896881754,-1.,1.28911506584254));
#30435=CARTESIAN_POINT('Ctrl Pts',(1.49618896881754,1.,1.28911506584254));
#30436=CARTESIAN_POINT('Ctrl Pts',(1.50178230149776,-1.,1.29145022885181));
#30437=CARTESIAN_POINT('Ctrl Pts',(1.50178230149776,1.,1.29145022885181));
#30438=CARTESIAN_POINT('Ctrl Pts',(1.50741159078365,-1.,1.29373841372842));
#30439=CARTESIAN_POINT('Ctrl Pts',(1.50741159078365,1.,1.29373841372842));
#30440=CARTESIAN_POINT('Ctrl Pts',(1.51305994241402,-1.,1.29596850710509));
#30441=CARTESIAN_POINT('Ctrl Pts',(1.51305994241402,1.,1.29596850710509));
#30442=CARTESIAN_POINT('Ctrl Pts',(1.51872184912724,-1.,1.29813791800747));
#30443=CARTESIAN_POINT('Ctrl Pts',(1.51872184912724,1.,1.29813791800747));
#30444=CARTESIAN_POINT('Ctrl Pts',(1.52439957861062,-1.,1.30024984366328));
#30445=CARTESIAN_POINT('Ctrl Pts',(1.52439957861062,1.,1.30024984366328));
#30446=CARTESIAN_POINT('Ctrl Pts',(1.53009970283891,-1.,1.30231064395568));
#30447=CARTESIAN_POINT('Ctrl Pts',(1.53009970283891,1.,1.30231064395568));
#30448=CARTESIAN_POINT('Ctrl Pts',(1.53582981268977,-1.,1.30432735639489));
#30449=CARTESIAN_POINT('Ctrl Pts',(1.53582981268977,1.,1.30432735639489));
#30450=CARTESIAN_POINT('Ctrl Pts',(1.54159462645432,-1.,1.30630475189556));
#30451=CARTESIAN_POINT('Ctrl Pts',(1.54159462645432,1.,1.30630475189556));
#30452=CARTESIAN_POINT('Ctrl Pts',(1.54739413957185,-1.,1.30824393907473));
#30453=CARTESIAN_POINT('Ctrl Pts',(1.54739413957185,1.,1.30824393907473));
#30454=CARTESIAN_POINT('Ctrl Pts',(1.55322568759481,-1.,1.31014393684222));
#30455=CARTESIAN_POINT('Ctrl Pts',(1.55322568759481,1.,1.31014393684222));
#30456=CARTESIAN_POINT('Ctrl Pts',(1.55908521254821,-1.,1.31200264341696));
#30457=CARTESIAN_POINT('Ctrl Pts',(1.55908521254821,1.,1.31200264341696));
#30458=CARTESIAN_POINT('Ctrl Pts',(1.56496872402353,-1.,1.31381795281002));
#30459=CARTESIAN_POINT('Ctrl Pts',(1.56496872402353,1.,1.31381795281002));
#30460=CARTESIAN_POINT('Ctrl Pts',(1.57087397835723,-1.,1.31558903860016));
#30461=CARTESIAN_POINT('Ctrl Pts',(1.57087397835723,1.,1.31558903860016));
#30462=CARTESIAN_POINT('Ctrl Pts',(1.5768005650559,-1.,1.31731642317187));
#30463=CARTESIAN_POINT('Ctrl Pts',(1.5768005650559,1.,1.31731642317187));
#30464=CARTESIAN_POINT('Ctrl Pts',(1.58274907898834,-1.,1.31900135021432));
#30465=CARTESIAN_POINT('Ctrl Pts',(1.58274907898834,1.,1.31900135021432));
#30466=CARTESIAN_POINT('Ctrl Pts',(1.58872057258245,-1.,1.32064537110892));
#30467=CARTESIAN_POINT('Ctrl Pts',(1.58872057258245,1.,1.32064537110892));
#30468=CARTESIAN_POINT('Ctrl Pts',(1.59471591079403,-1.,1.32224985747682));
#30469=CARTESIAN_POINT('Ctrl Pts',(1.59471591079403,1.,1.32224985747682));
#30470=CARTESIAN_POINT('Ctrl Pts',(1.60073511858687,-1.,1.32381550858256));
#30471=CARTESIAN_POINT('Ctrl Pts',(1.60073511858687,1.,1.32381550858256));
#30472=CARTESIAN_POINT('Ctrl Pts',(1.60677758290954,-1.,1.32534250785782));
#30473=CARTESIAN_POINT('Ctrl Pts',(1.60677758290954,1.,1.32534250785782));
#30474=CARTESIAN_POINT('Ctrl Pts',(1.6128423401575,-1.,1.32683074483356));
#30475=CARTESIAN_POINT('Ctrl Pts',(1.6128423401575,1.,1.32683074483356));
#30476=CARTESIAN_POINT('Ctrl Pts',(1.61892832270724,-1.,1.32828000610449));
#30477=CARTESIAN_POINT('Ctrl Pts',(1.61892832270724,1.,1.32828000610449));
#30478=CARTESIAN_POINT('Ctrl Pts',(1.62503464209797,-1.,1.3296901950568));
#30479=CARTESIAN_POINT('Ctrl Pts',(1.62503464209797,1.,1.3296901950568));
#30480=CARTESIAN_POINT('Ctrl Pts',(1.63116079730923,-1.,1.33106149345645));
#30481=CARTESIAN_POINT('Ctrl Pts',(1.63116079730923,1.,1.33106149345645));
#30482=CARTESIAN_POINT('Ctrl Pts',(1.63730653475089,-1.,1.33239425103724));
#30483=CARTESIAN_POINT('Ctrl Pts',(1.63730653475089,1.,1.33239425103724));
#30484=CARTESIAN_POINT('Ctrl Pts',(1.6434717485603,-1.,1.33368890676572));
#30485=CARTESIAN_POINT('Ctrl Pts',(1.6434717485603,1.,1.33368890676572));
#30486=CARTESIAN_POINT('Ctrl Pts',(1.6496563728683,-1.,1.33494590467993));
#30487=CARTESIAN_POINT('Ctrl Pts',(1.6496563728683,1.,1.33494590467993));
#30488=CARTESIAN_POINT('Ctrl Pts',(1.65586025952593,-1.,1.33616559745172));
#30489=CARTESIAN_POINT('Ctrl Pts',(1.65586025952593,1.,1.33616559745172));
#30490=CARTESIAN_POINT('Ctrl Pts',(1.66208312541983,-1.,1.33734820885262));
#30491=CARTESIAN_POINT('Ctrl Pts',(1.66208312541983,1.,1.33734820885262));
#30492=CARTESIAN_POINT('Ctrl Pts',(1.66832460783989,-1.,1.33849388654388));
#30493=CARTESIAN_POINT('Ctrl Pts',(1.66832460783989,1.,1.33849388654388));
#30494=CARTESIAN_POINT('Ctrl Pts',(1.67458429426086,-1.,1.3396027347034));
#30495=CARTESIAN_POINT('Ctrl Pts',(1.67458429426086,1.,1.3396027347034));
#30496=CARTESIAN_POINT('Ctrl Pts',(1.68086176030362,-1.,1.34067485185203));
#30497=CARTESIAN_POINT('Ctrl Pts',(1.68086176030362,1.,1.34067485185203));
#30498=CARTESIAN_POINT('Ctrl Pts',(1.68715660868764,-1.,1.341710374848));
#30499=CARTESIAN_POINT('Ctrl Pts',(1.68715660868764,1.,1.341710374848));
#30500=CARTESIAN_POINT('Ctrl Pts',(1.6934684849687,-1.,1.34270948206319));
#30501=CARTESIAN_POINT('Ctrl Pts',(1.6934684849687,1.,1.34270948206319));
#30502=CARTESIAN_POINT('Ctrl Pts',(1.69979707754427,-1.,1.34367237124483));
#30503=CARTESIAN_POINT('Ctrl Pts',(1.69979707754427,1.,1.34367237124483));
#30504=CARTESIAN_POINT('Ctrl Pts',(1.70614212266738,-1.,1.34459924533831));
#30505=CARTESIAN_POINT('Ctrl Pts',(1.70614212266738,1.,1.34459924533831));
#30506=CARTESIAN_POINT('Ctrl Pts',(1.71250340686822,-1.,1.34549029589416));
#30507=CARTESIAN_POINT('Ctrl Pts',(1.71250340686822,1.,1.34549029589416));
#30508=CARTESIAN_POINT('Ctrl Pts',(1.7188807715049,-1.,1.34634568653227));
#30509=CARTESIAN_POINT('Ctrl Pts',(1.7188807715049,1.,1.34634568653227));
#30510=CARTESIAN_POINT('Ctrl Pts',(1.72527410680674,-1.,1.34716554819527));
#30511=CARTESIAN_POINT('Ctrl Pts',(1.72527410680674,1.,1.34716554819527));
#30512=CARTESIAN_POINT('Ctrl Pts',(1.7304014965394,-1.,1.34779309152035));
#30513=CARTESIAN_POINT('Ctrl Pts',(1.7304014965394,1.,1.34779309152035));
#30514=CARTESIAN_POINT('Ctrl Pts',(1.73425417885907,-1.,1.34824783112887));
#30515=CARTESIAN_POINT('Ctrl Pts',(1.73425417885907,1.,1.34824783112887));
#30516=CARTESIAN_POINT('Ctrl Pts',(1.73682580585691,-1.,1.34854391898045));
#30517=CARTESIAN_POINT('Ctrl Pts',(1.73682580585691,1.,1.34854391898045));
#30518=CARTESIAN_POINT('Ctrl Pts',(1.73811241238545,-1.,1.34869019493419));
#30519=CARTESIAN_POINT('Ctrl Pts',(1.73811241238545,1.,1.34869019493419));
#30520=CARTESIAN_POINT('',(1.31362392696032,1.,1.15624053661742));
#30521=CARTESIAN_POINT('Ctrl Pts',(1.31362392696032,1.,1.15624053661742));
#30522=CARTESIAN_POINT('Ctrl Pts',(1.31722977216397,1.,1.15950888730809));
#30523=CARTESIAN_POINT('Ctrl Pts',(1.32428080721772,1.,1.16589330093588));
#30524=CARTESIAN_POINT('Ctrl Pts',(1.33437539347008,1.,1.17501305789857));
#30525=CARTESIAN_POINT('Ctrl Pts',(1.34687054001093,1.,1.18625865667441));
#30526=CARTESIAN_POINT('Ctrl Pts',(1.36088705043885,1.,1.1987959077932));
#30527=CARTESIAN_POINT('Ctrl Pts',(1.37331915607905,1.,1.20982812925645));
#30528=CARTESIAN_POINT('Ctrl Pts',(1.38420564527715,1.,1.21938737280852));
#30529=CARTESIAN_POINT('Ctrl Pts',(1.39361389568796,1.,1.22752961899387));
#30530=CARTESIAN_POINT('Ctrl Pts',(1.40164708206106,1.,1.23434087290423));
#30531=CARTESIAN_POINT('Ctrl Pts',(1.40845295531283,1.,1.23994455029534));
#30532=CARTESIAN_POINT('Ctrl Pts',(1.41422913175179,1.,1.24450600513056));
#30533=CARTESIAN_POINT('Ctrl Pts',(1.41923722596025,1.,1.24824430986571));
#30534=CARTESIAN_POINT('Ctrl Pts',(1.42378102115575,1.,1.2514145557001));
#30535=CARTESIAN_POINT('Ctrl Pts',(1.42815938799387,1.,1.25426945222639));
#30536=CARTESIAN_POINT('Ctrl Pts',(1.43262645609691,1.,1.25702687965755));
#30537=CARTESIAN_POINT('Ctrl Pts',(1.43734919180847,1.,1.25983531012005));
#30538=CARTESIAN_POINT('Ctrl Pts',(1.44236470511303,1.,1.26273903323859));
#30539=CARTESIAN_POINT('Ctrl Pts',(1.44761985001662,1.,1.26570925118868));
#30540=CARTESIAN_POINT('Ctrl Pts',(1.45301422764247,1.,1.2686778680489));
#30541=CARTESIAN_POINT('Ctrl Pts',(1.45843906294697,1.,1.27156805265289));
#30542=CARTESIAN_POINT('Ctrl Pts',(1.46382431332476,1.,1.27433119897822));
#30543=CARTESIAN_POINT('Ctrl Pts',(1.46916035917133,1.,1.2769641483109));
#30544=CARTESIAN_POINT('Ctrl Pts',(1.4744717526707,1.,1.2794891824849));
#30545=CARTESIAN_POINT('Ctrl Pts',(1.47980070347095,1.,1.28194158939517));
#30546=CARTESIAN_POINT('Ctrl Pts',(1.4851881711891,1.,1.28435533880201));
#30547=CARTESIAN_POINT('Ctrl Pts',(1.4906522831278,1.,1.2867467611644));
#30548=CARTESIAN_POINT('Ctrl Pts',(1.49618896881754,1.,1.28911506584254));
#30549=CARTESIAN_POINT('Ctrl Pts',(1.50178230149776,1.,1.29145022885181));
#30550=CARTESIAN_POINT('Ctrl Pts',(1.50741159078365,1.,1.29373841372842));
#30551=CARTESIAN_POINT('Ctrl Pts',(1.51305994241402,1.,1.29596850710509));
#30552=CARTESIAN_POINT('Ctrl Pts',(1.51872184912724,1.,1.29813791800747));
#30553=CARTESIAN_POINT('Ctrl Pts',(1.52439957861062,1.,1.30024984366328));
#30554=CARTESIAN_POINT('Ctrl Pts',(1.53009970283891,1.,1.30231064395568));
#30555=CARTESIAN_POINT('Ctrl Pts',(1.53582981268977,1.,1.30432735639489));
#30556=CARTESIAN_POINT('Ctrl Pts',(1.54159462645432,1.,1.30630475189556));
#30557=CARTESIAN_POINT('Ctrl Pts',(1.54739413957185,1.,1.30824393907473));
#30558=CARTESIAN_POINT('Ctrl Pts',(1.55322568759481,1.,1.31014393684222));
#30559=CARTESIAN_POINT('Ctrl Pts',(1.55908521254821,1.,1.31200264341696));
#30560=CARTESIAN_POINT('Ctrl Pts',(1.56496872402353,1.,1.31381795281002));
#30561=CARTESIAN_POINT('Ctrl Pts',(1.57087397835723,1.,1.31558903860016));
#30562=CARTESIAN_POINT('Ctrl Pts',(1.5768005650559,1.,1.31731642317187));
#30563=CARTESIAN_POINT('Ctrl Pts',(1.58274907898834,1.,1.31900135021432));
#30564=CARTESIAN_POINT('Ctrl Pts',(1.58872057258245,1.,1.32064537110892));
#30565=CARTESIAN_POINT('Ctrl Pts',(1.59471591079403,1.,1.32224985747682));
#30566=CARTESIAN_POINT('Ctrl Pts',(1.60073511858687,1.,1.32381550858256));
#30567=CARTESIAN_POINT('Ctrl Pts',(1.60677758290954,1.,1.32534250785782));
#30568=CARTESIAN_POINT('Ctrl Pts',(1.6128423401575,1.,1.32683074483356));
#30569=CARTESIAN_POINT('Ctrl Pts',(1.61892832270724,1.,1.32828000610449));
#30570=CARTESIAN_POINT('Ctrl Pts',(1.62503464209797,1.,1.3296901950568));
#30571=CARTESIAN_POINT('Ctrl Pts',(1.63116079730923,1.,1.33106149345645));
#30572=CARTESIAN_POINT('Ctrl Pts',(1.63730653475089,1.,1.33239425103724));
#30573=CARTESIAN_POINT('Ctrl Pts',(1.6434717485603,1.,1.33368890676572));
#30574=CARTESIAN_POINT('Ctrl Pts',(1.6496563728683,1.,1.33494590467993));
#30575=CARTESIAN_POINT('Ctrl Pts',(1.65586025952593,1.,1.33616559745172));
#30576=CARTESIAN_POINT('Ctrl Pts',(1.66208312541983,1.,1.33734820885262));
#30577=CARTESIAN_POINT('Ctrl Pts',(1.66832460783989,1.,1.33849388654388));
#30578=CARTESIAN_POINT('Ctrl Pts',(1.67458429426086,1.,1.3396027347034));
#30579=CARTESIAN_POINT('Ctrl Pts',(1.68086176030362,1.,1.34067485185203));
#30580=CARTESIAN_POINT('Ctrl Pts',(1.68715660868764,1.,1.341710374848));
#30581=CARTESIAN_POINT('Ctrl Pts',(1.6934684849687,1.,1.34270948206319));
#30582=CARTESIAN_POINT('Ctrl Pts',(1.69979707754427,1.,1.34367237124483));
#30583=CARTESIAN_POINT('Ctrl Pts',(1.70614212266738,1.,1.34459924533831));
#30584=CARTESIAN_POINT('Ctrl Pts',(1.71250340686822,1.,1.34549029589416));
#30585=CARTESIAN_POINT('Ctrl Pts',(1.7188807715049,1.,1.34634568653227));
#30586=CARTESIAN_POINT('Ctrl Pts',(1.72527410680674,1.,1.34716554819527));
#30587=CARTESIAN_POINT('Ctrl Pts',(1.7304014965394,1.,1.34779309152035));
#30588=CARTESIAN_POINT('Ctrl Pts',(1.73425417885907,1.,1.34824783112887));
#30589=CARTESIAN_POINT('Ctrl Pts',(1.73682580585691,1.,1.34854391898045));
#30590=CARTESIAN_POINT('Ctrl Pts',(1.73811241238545,1.,1.34869019493419));
#30591=CARTESIAN_POINT('',(1.31362392696032,0.,1.15624053661742));
#30592=CARTESIAN_POINT('Origin',(0.,0.,0.));
#30593=CARTESIAN_POINT('',(1.15624053661742,1.,1.31362392696033));
#30594=CARTESIAN_POINT('Origin',(0.,1.,0.));
#30595=CARTESIAN_POINT('',(1.15624053661742,0.,1.31362392696032));
#30596=CARTESIAN_POINT('Ctrl Pts',(1.34869019493419,-1.,1.73811241238545));
#30597=CARTESIAN_POINT('Ctrl Pts',(1.34869019493419,1.,1.73811241238545));
#30598=CARTESIAN_POINT('Ctrl Pts',(1.34854391898145,-1.,1.73682580585819));
#30599=CARTESIAN_POINT('Ctrl Pts',(1.34854391898145,1.,1.73682580585819));
#30600=CARTESIAN_POINT('Ctrl Pts',(1.34824783113158,-1.,1.73425417886255));
#30601=CARTESIAN_POINT('Ctrl Pts',(1.34824783113158,1.,1.73425417886255));
#30602=CARTESIAN_POINT('Ctrl Pts',(1.3477930915247,-1.,1.73040149654497));
#30603=CARTESIAN_POINT('Ctrl Pts',(1.3477930915247,1.,1.73040149654497));
#30604=CARTESIAN_POINT('Ctrl Pts',(1.34716554820013,-1.,1.72527410681298));
#30605=CARTESIAN_POINT('Ctrl Pts',(1.34716554820013,1.,1.72527410681298));
#30606=CARTESIAN_POINT('Ctrl Pts',(1.34634568653586,-1.,1.7188807715095));
#30607=CARTESIAN_POINT('Ctrl Pts',(1.34634568653586,1.,1.7188807715095));
#30608=CARTESIAN_POINT('Ctrl Pts',(1.34549029589563,-1.,1.71250340687011));
#30609=CARTESIAN_POINT('Ctrl Pts',(1.34549029589563,1.,1.71250340687011));
#30610=CARTESIAN_POINT('Ctrl Pts',(1.34459924533783,-1.,1.70614212266676));
#30611=CARTESIAN_POINT('Ctrl Pts',(1.34459924533783,1.,1.70614212266676));
#30612=CARTESIAN_POINT('Ctrl Pts',(1.34367237124322,-1.,1.69979707754221));
#30613=CARTESIAN_POINT('Ctrl Pts',(1.34367237124322,1.,1.69979707754221));
#30614=CARTESIAN_POINT('Ctrl Pts',(1.34270948206139,-1.,1.6934684849664));
#30615=CARTESIAN_POINT('Ctrl Pts',(1.34270948206139,1.,1.6934684849664));
#30616=CARTESIAN_POINT('Ctrl Pts',(1.34171037484673,-1.,1.68715660868602));
#30617=CARTESIAN_POINT('Ctrl Pts',(1.34171037484673,1.,1.68715660868602));
#30618=CARTESIAN_POINT('Ctrl Pts',(1.3406748518516,-1.,1.68086176030308));
#30619=CARTESIAN_POINT('Ctrl Pts',(1.3406748518516,1.,1.68086176030308));
#30620=CARTESIAN_POINT('Ctrl Pts',(1.33960273470372,-1.,1.67458429426126));
#30621=CARTESIAN_POINT('Ctrl Pts',(1.33960273470372,1.,1.67458429426126));
#30622=CARTESIAN_POINT('Ctrl Pts',(1.33849388654458,-1.,1.66832460784078));
#30623=CARTESIAN_POINT('Ctrl Pts',(1.33849388654458,1.,1.66832460784078));
#30624=CARTESIAN_POINT('Ctrl Pts',(1.33734820885331,-1.,1.66208312542073));
#30625=CARTESIAN_POINT('Ctrl Pts',(1.33734820885331,1.,1.66208312542073));
#30626=CARTESIAN_POINT('Ctrl Pts',(1.33616559745217,-1.,1.65586025952651));
#30627=CARTESIAN_POINT('Ctrl Pts',(1.33616559745217,1.,1.65586025952651));
#30628=CARTESIAN_POINT('Ctrl Pts',(1.33494590468003,-1.,1.64965637286843));
#30629=CARTESIAN_POINT('Ctrl Pts',(1.33494590468003,1.,1.64965637286843));
#30630=CARTESIAN_POINT('Ctrl Pts',(1.33368890676554,-1.,1.64347174856007));
#30631=CARTESIAN_POINT('Ctrl Pts',(1.33368890676554,1.,1.64347174856007));
#30632=CARTESIAN_POINT('Ctrl Pts',(1.33239425103694,-1.,1.6373065347505));
#30633=CARTESIAN_POINT('Ctrl Pts',(1.33239425103694,1.,1.6373065347505));
#30634=CARTESIAN_POINT('Ctrl Pts',(1.33106149345618,-1.,1.63116079730887));
#30635=CARTESIAN_POINT('Ctrl Pts',(1.33106149345618,1.,1.63116079730887));
#30636=CARTESIAN_POINT('Ctrl Pts',(1.32969019505665,-1.,1.62503464209777));
#30637=CARTESIAN_POINT('Ctrl Pts',(1.32969019505665,1.,1.62503464209777));
#30638=CARTESIAN_POINT('Ctrl Pts',(1.32828000610448,-1.,1.61892832270723));
#30639=CARTESIAN_POINT('Ctrl Pts',(1.32828000610448,1.,1.61892832270723));
#30640=CARTESIAN_POINT('Ctrl Pts',(1.32683074483365,-1.,1.61284234015762));
#30641=CARTESIAN_POINT('Ctrl Pts',(1.32683074483365,1.,1.61284234015762));
#30642=CARTESIAN_POINT('Ctrl Pts',(1.32534250785794,-1.,1.6067775829097));
#30643=CARTESIAN_POINT('Ctrl Pts',(1.32534250785794,1.,1.6067775829097));
#30644=CARTESIAN_POINT('Ctrl Pts',(1.32381550858266,-1.,1.600735118587));
#30645=CARTESIAN_POINT('Ctrl Pts',(1.32381550858266,1.,1.600735118587));
#30646=CARTESIAN_POINT('Ctrl Pts',(1.32224985747686,-1.,1.59471591079408));
#30647=CARTESIAN_POINT('Ctrl Pts',(1.32224985747686,1.,1.59471591079408));
#30648=CARTESIAN_POINT('Ctrl Pts',(1.32064537110891,-1.,1.58872057258244));
#30649=CARTESIAN_POINT('Ctrl Pts',(1.32064537110891,1.,1.58872057258244));
#30650=CARTESIAN_POINT('Ctrl Pts',(1.31900135021428,-1.,1.58274907898829));
#30651=CARTESIAN_POINT('Ctrl Pts',(1.31900135021428,1.,1.58274907898829));
#30652=CARTESIAN_POINT('Ctrl Pts',(1.31731642317183,-1.,1.57680056505585));
#30653=CARTESIAN_POINT('Ctrl Pts',(1.31731642317183,1.,1.57680056505585));
#30654=CARTESIAN_POINT('Ctrl Pts',(1.31558903860015,-1.,1.57087397835721));
#30655=CARTESIAN_POINT('Ctrl Pts',(1.31558903860015,1.,1.57087397835721));
#30656=CARTESIAN_POINT('Ctrl Pts',(1.31381795281002,-1.,1.56496872402352));
#30657=CARTESIAN_POINT('Ctrl Pts',(1.31381795281002,1.,1.56496872402352));
#30658=CARTESIAN_POINT('Ctrl Pts',(1.31200264341696,-1.,1.55908521254822));
#30659=CARTESIAN_POINT('Ctrl Pts',(1.31200264341696,1.,1.55908521254822));
#30660=CARTESIAN_POINT('Ctrl Pts',(1.31014393684221,-1.,1.55322568759481));
#30661=CARTESIAN_POINT('Ctrl Pts',(1.31014393684221,1.,1.55322568759481));
#30662=CARTESIAN_POINT('Ctrl Pts',(1.30824393907471,-1.,1.54739413957183));
#30663=CARTESIAN_POINT('Ctrl Pts',(1.30824393907471,1.,1.54739413957183));
#30664=CARTESIAN_POINT('Ctrl Pts',(1.30630475189553,-1.,1.54159462645428));
#30665=CARTESIAN_POINT('Ctrl Pts',(1.30630475189553,1.,1.54159462645428));
#30666=CARTESIAN_POINT('Ctrl Pts',(1.30432735639487,-1.,1.53582981268976));
#30667=CARTESIAN_POINT('Ctrl Pts',(1.30432735639487,1.,1.53582981268976));
#30668=CARTESIAN_POINT('Ctrl Pts',(1.3023106439557,-1.,1.53009970283893));
#30669=CARTESIAN_POINT('Ctrl Pts',(1.3023106439557,1.,1.53009970283893));
#30670=CARTESIAN_POINT('Ctrl Pts',(1.30024984366334,-1.,1.5243995786107));
#30671=CARTESIAN_POINT('Ctrl Pts',(1.30024984366334,1.,1.5243995786107));
#30672=CARTESIAN_POINT('Ctrl Pts',(1.29813791800757,-1.,1.51872184912735));
#30673=CARTESIAN_POINT('Ctrl Pts',(1.29813791800757,1.,1.51872184912735));
#30674=CARTESIAN_POINT('Ctrl Pts',(1.29596850710518,-1.,1.51305994241412));
#30675=CARTESIAN_POINT('Ctrl Pts',(1.29596850710518,1.,1.51305994241412));
#30676=CARTESIAN_POINT('Ctrl Pts',(1.29373841372843,-1.,1.50741159078367));
#30677=CARTESIAN_POINT('Ctrl Pts',(1.29373841372843,1.,1.50741159078367));
#30678=CARTESIAN_POINT('Ctrl Pts',(1.29145022885171,-1.,1.50178230149764));
#30679=CARTESIAN_POINT('Ctrl Pts',(1.29145022885171,1.,1.50178230149764));
#30680=CARTESIAN_POINT('Ctrl Pts',(1.28911506584232,-1.,1.49618896881729));
#30681=CARTESIAN_POINT('Ctrl Pts',(1.28911506584232,1.,1.49618896881729));
#30682=CARTESIAN_POINT('Ctrl Pts',(1.28674676116415,-1.,1.4906522831275));
#30683=CARTESIAN_POINT('Ctrl Pts',(1.28674676116415,1.,1.4906522831275));
#30684=CARTESIAN_POINT('Ctrl Pts',(1.28435533880184,-1.,1.48518817118891));
#30685=CARTESIAN_POINT('Ctrl Pts',(1.28435533880184,1.,1.48518817118891));
#30686=CARTESIAN_POINT('Ctrl Pts',(1.28194158939522,-1.,1.47980070347102));
#30687=CARTESIAN_POINT('Ctrl Pts',(1.28194158939522,1.,1.47980070347102));
#30688=CARTESIAN_POINT('Ctrl Pts',(1.27948918248524,-1.,1.4744717526711));
#30689=CARTESIAN_POINT('Ctrl Pts',(1.27948918248524,1.,1.4744717526711));
#30690=CARTESIAN_POINT('Ctrl Pts',(1.27696414831144,-1.,1.46916035917197));
#30691=CARTESIAN_POINT('Ctrl Pts',(1.27696414831144,1.,1.46916035917197));
#30692=CARTESIAN_POINT('Ctrl Pts',(1.27433119897877,-1.,1.4638243133254));
#30693=CARTESIAN_POINT('Ctrl Pts',(1.27433119897877,1.,1.4638243133254));
#30694=CARTESIAN_POINT('Ctrl Pts',(1.27156805265312,-1.,1.45843906294725));
#30695=CARTESIAN_POINT('Ctrl Pts',(1.27156805265312,1.,1.45843906294725));
#30696=CARTESIAN_POINT('Ctrl Pts',(1.26867786804854,-1.,1.45301422764205));
#30697=CARTESIAN_POINT('Ctrl Pts',(1.26867786804854,1.,1.45301422764205));
#30698=CARTESIAN_POINT('Ctrl Pts',(1.26570925118767,-1.,1.44761985001544));
#30699=CARTESIAN_POINT('Ctrl Pts',(1.26570925118767,1.,1.44761985001544));
#30700=CARTESIAN_POINT('Ctrl Pts',(1.26273903323723,-1.,1.44236470511145));
#30701=CARTESIAN_POINT('Ctrl Pts',(1.26273903323723,1.,1.44236470511145));
#30702=CARTESIAN_POINT('Ctrl Pts',(1.25983531011894,-1.,1.43734919180719));
#30703=CARTESIAN_POINT('Ctrl Pts',(1.25983531011894,1.,1.43734919180719));
#30704=CARTESIAN_POINT('Ctrl Pts',(1.25702687965744,-1.,1.43262645609679));
#30705=CARTESIAN_POINT('Ctrl Pts',(1.25702687965744,1.,1.43262645609679));
#30706=CARTESIAN_POINT('Ctrl Pts',(1.25426945222783,-1.,1.42815938799555));
#30707=CARTESIAN_POINT('Ctrl Pts',(1.25426945222783,1.,1.42815938799555));
#30708=CARTESIAN_POINT('Ctrl Pts',(1.25141455570299,-1.,1.42378102115911));
#30709=CARTESIAN_POINT('Ctrl Pts',(1.25141455570299,1.,1.42378102115911));
#30710=CARTESIAN_POINT('Ctrl Pts',(1.24824430986911,-1.,1.41923722596421));
#30711=CARTESIAN_POINT('Ctrl Pts',(1.24824430986911,1.,1.41923722596421));
#30712=CARTESIAN_POINT('Ctrl Pts',(1.24450600513278,-1.,1.41422913175437));
#30713=CARTESIAN_POINT('Ctrl Pts',(1.24450600513278,1.,1.41422913175437));
#30714=CARTESIAN_POINT('Ctrl Pts',(1.23994455029421,-1.,1.40845295531151));
#30715=CARTESIAN_POINT('Ctrl Pts',(1.23994455029421,1.,1.40845295531151));
#30716=CARTESIAN_POINT('Ctrl Pts',(1.23434087289768,-1.,1.40164708205345));
#30717=CARTESIAN_POINT('Ctrl Pts',(1.23434087289768,1.,1.40164708205345));
#30718=CARTESIAN_POINT('Ctrl Pts',(1.22752961898063,-1.,1.39361389567257));
#30719=CARTESIAN_POINT('Ctrl Pts',(1.22752961898063,1.,1.39361389567257));
#30720=CARTESIAN_POINT('Ctrl Pts',(1.21938737278853,-1.,1.38420564525391));
#30721=CARTESIAN_POINT('Ctrl Pts',(1.21938737278853,1.,1.38420564525391));
#30722=CARTESIAN_POINT('Ctrl Pts',(1.20982812923113,-1.,1.37331915604962));
#30723=CARTESIAN_POINT('Ctrl Pts',(1.20982812923113,1.,1.37331915604962));
#30724=CARTESIAN_POINT('Ctrl Pts',(1.1987959077656,-1.,1.36088705040677));
#30725=CARTESIAN_POINT('Ctrl Pts',(1.1987959077656,1.,1.36088705040677));
#30726=CARTESIAN_POINT('Ctrl Pts',(1.18625865664915,-1.,1.34687053998157));
#30727=CARTESIAN_POINT('Ctrl Pts',(1.18625865664915,1.,1.34687053998157));
#30728=CARTESIAN_POINT('Ctrl Pts',(1.17501305787994,-1.,1.33437539344842));
#30729=CARTESIAN_POINT('Ctrl Pts',(1.17501305787994,1.,1.33437539344842));
#30730=CARTESIAN_POINT('Ctrl Pts',(1.16589330092532,-1.,1.32428080720544));
#30731=CARTESIAN_POINT('Ctrl Pts',(1.16589330092532,1.,1.32428080720544));
#30732=CARTESIAN_POINT('Ctrl Pts',(1.15950888730433,-1.,1.3172297721596));
#30733=CARTESIAN_POINT('Ctrl Pts',(1.15950888730433,1.,1.3172297721596));
#30734=CARTESIAN_POINT('Ctrl Pts',(1.15624053661742,-1.,1.31362392696033));
#30735=CARTESIAN_POINT('Ctrl Pts',(1.15624053661742,1.,1.31362392696033));
#30736=CARTESIAN_POINT('',(1.34869019493419,1.,1.73811241238545));
#30737=CARTESIAN_POINT('Ctrl Pts',(1.34869019493419,1.,1.73811241238545));
#30738=CARTESIAN_POINT('Ctrl Pts',(1.34854391898145,1.,1.73682580585819));
#30739=CARTESIAN_POINT('Ctrl Pts',(1.34824783113158,1.,1.73425417886255));
#30740=CARTESIAN_POINT('Ctrl Pts',(1.3477930915247,1.,1.73040149654497));
#30741=CARTESIAN_POINT('Ctrl Pts',(1.34716554820013,1.,1.72527410681298));
#30742=CARTESIAN_POINT('Ctrl Pts',(1.34634568653586,1.,1.7188807715095));
#30743=CARTESIAN_POINT('Ctrl Pts',(1.34549029589563,1.,1.71250340687011));
#30744=CARTESIAN_POINT('Ctrl Pts',(1.34459924533783,1.,1.70614212266676));
#30745=CARTESIAN_POINT('Ctrl Pts',(1.34367237124322,1.,1.69979707754221));
#30746=CARTESIAN_POINT('Ctrl Pts',(1.34270948206139,1.,1.6934684849664));
#30747=CARTESIAN_POINT('Ctrl Pts',(1.34171037484673,1.,1.68715660868602));
#30748=CARTESIAN_POINT('Ctrl Pts',(1.3406748518516,1.,1.68086176030308));
#30749=CARTESIAN_POINT('Ctrl Pts',(1.33960273470372,1.,1.67458429426126));
#30750=CARTESIAN_POINT('Ctrl Pts',(1.33849388654458,1.,1.66832460784078));
#30751=CARTESIAN_POINT('Ctrl Pts',(1.33734820885331,1.,1.66208312542073));
#30752=CARTESIAN_POINT('Ctrl Pts',(1.33616559745217,1.,1.65586025952651));
#30753=CARTESIAN_POINT('Ctrl Pts',(1.33494590468003,1.,1.64965637286843));
#30754=CARTESIAN_POINT('Ctrl Pts',(1.33368890676554,1.,1.64347174856007));
#30755=CARTESIAN_POINT('Ctrl Pts',(1.33239425103694,1.,1.6373065347505));
#30756=CARTESIAN_POINT('Ctrl Pts',(1.33106149345618,1.,1.63116079730887));
#30757=CARTESIAN_POINT('Ctrl Pts',(1.32969019505665,1.,1.62503464209777));
#30758=CARTESIAN_POINT('Ctrl Pts',(1.32828000610448,1.,1.61892832270723));
#30759=CARTESIAN_POINT('Ctrl Pts',(1.32683074483365,1.,1.61284234015762));
#30760=CARTESIAN_POINT('Ctrl Pts',(1.32534250785794,1.,1.6067775829097));
#30761=CARTESIAN_POINT('Ctrl Pts',(1.32381550858266,1.,1.600735118587));
#30762=CARTESIAN_POINT('Ctrl Pts',(1.32224985747686,1.,1.59471591079408));
#30763=CARTESIAN_POINT('Ctrl Pts',(1.32064537110891,1.,1.58872057258244));
#30764=CARTESIAN_POINT('Ctrl Pts',(1.31900135021428,1.,1.58274907898829));
#30765=CARTESIAN_POINT('Ctrl Pts',(1.31731642317183,1.,1.57680056505585));
#30766=CARTESIAN_POINT('Ctrl Pts',(1.31558903860015,1.,1.57087397835721));
#30767=CARTESIAN_POINT('Ctrl Pts',(1.31381795281002,1.,1.56496872402352));
#30768=CARTESIAN_POINT('Ctrl Pts',(1.31200264341696,1.,1.55908521254822));
#30769=CARTESIAN_POINT('Ctrl Pts',(1.31014393684221,1.,1.55322568759481));
#30770=CARTESIAN_POINT('Ctrl Pts',(1.30824393907471,1.,1.54739413957183));
#30771=CARTESIAN_POINT('Ctrl Pts',(1.30630475189553,1.,1.54159462645428));
#30772=CARTESIAN_POINT('Ctrl Pts',(1.30432735639487,1.,1.53582981268976));
#30773=CARTESIAN_POINT('Ctrl Pts',(1.3023106439557,1.,1.53009970283893));
#30774=CARTESIAN_POINT('Ctrl Pts',(1.30024984366334,1.,1.5243995786107));
#30775=CARTESIAN_POINT('Ctrl Pts',(1.29813791800757,1.,1.51872184912735));
#30776=CARTESIAN_POINT('Ctrl Pts',(1.29596850710518,1.,1.51305994241412));
#30777=CARTESIAN_POINT('Ctrl Pts',(1.29373841372843,1.,1.50741159078367));
#30778=CARTESIAN_POINT('Ctrl Pts',(1.29145022885171,1.,1.50178230149764));
#30779=CARTESIAN_POINT('Ctrl Pts',(1.28911506584232,1.,1.49618896881729));
#30780=CARTESIAN_POINT('Ctrl Pts',(1.28674676116415,1.,1.4906522831275));
#30781=CARTESIAN_POINT('Ctrl Pts',(1.28435533880184,1.,1.48518817118891));
#30782=CARTESIAN_POINT('Ctrl Pts',(1.28194158939522,1.,1.47980070347102));
#30783=CARTESIAN_POINT('Ctrl Pts',(1.27948918248524,1.,1.4744717526711));
#30784=CARTESIAN_POINT('Ctrl Pts',(1.27696414831144,1.,1.46916035917197));
#30785=CARTESIAN_POINT('Ctrl Pts',(1.27433119897877,1.,1.4638243133254));
#30786=CARTESIAN_POINT('Ctrl Pts',(1.27156805265312,1.,1.45843906294725));
#30787=CARTESIAN_POINT('Ctrl Pts',(1.26867786804854,1.,1.45301422764205));
#30788=CARTESIAN_POINT('Ctrl Pts',(1.26570925118767,1.,1.44761985001544));
#30789=CARTESIAN_POINT('Ctrl Pts',(1.26273903323723,1.,1.44236470511145));
#30790=CARTESIAN_POINT('Ctrl Pts',(1.25983531011894,1.,1.43734919180719));
#30791=CARTESIAN_POINT('Ctrl Pts',(1.25702687965744,1.,1.43262645609679));
#30792=CARTESIAN_POINT('Ctrl Pts',(1.25426945222783,1.,1.42815938799555));
#30793=CARTESIAN_POINT('Ctrl Pts',(1.25141455570299,1.,1.42378102115911));
#30794=CARTESIAN_POINT('Ctrl Pts',(1.24824430986911,1.,1.41923722596421));
#30795=CARTESIAN_POINT('Ctrl Pts',(1.24450600513278,1.,1.41422913175437));
#30796=CARTESIAN_POINT('Ctrl Pts',(1.23994455029421,1.,1.40845295531151));
#30797=CARTESIAN_POINT('Ctrl Pts',(1.23434087289768,1.,1.40164708205345));
#30798=CARTESIAN_POINT('Ctrl Pts',(1.22752961898063,1.,1.39361389567257));
#30799=CARTESIAN_POINT('Ctrl Pts',(1.21938737278853,1.,1.38420564525391));
#30800=CARTESIAN_POINT('Ctrl Pts',(1.20982812923113,1.,1.37331915604962));
#30801=CARTESIAN_POINT('Ctrl Pts',(1.1987959077656,1.,1.36088705040677));
#30802=CARTESIAN_POINT('Ctrl Pts',(1.18625865664915,1.,1.34687053998157));
#30803=CARTESIAN_POINT('Ctrl Pts',(1.17501305787994,1.,1.33437539344842));
#30804=CARTESIAN_POINT('Ctrl Pts',(1.16589330092532,1.,1.32428080720544));
#30805=CARTESIAN_POINT('Ctrl Pts',(1.15950888730433,1.,1.3172297721596));
#30806=CARTESIAN_POINT('Ctrl Pts',(1.15624053661742,1.,1.31362392696033));
#30807=CARTESIAN_POINT('',(1.34869019493419,0.,1.73811241238545));
#30808=CARTESIAN_POINT('Origin',(1.23627494547115,0.,1.81978687191668));
#30809=CARTESIAN_POINT('',(1.23627494547115,1.,1.81978687191668));
#30810=CARTESIAN_POINT('',(1.34869019493419,1.,1.73811241238545));
#30811=CARTESIAN_POINT('',(1.23627494547115,0.,1.81978687191668));
#30812=CARTESIAN_POINT('Ctrl Pts',(0.892032620296855,-1.,1.5055822144029));
#30813=CARTESIAN_POINT('Ctrl Pts',(0.892032620296855,1.,1.5055822144029));
#30814=CARTESIAN_POINT('Ctrl Pts',(0.894452006967538,-1.,1.50980486807181));
#30815=CARTESIAN_POINT('Ctrl Pts',(0.894452006967538,1.,1.50980486807181));
#30816=CARTESIAN_POINT('Ctrl Pts',(0.89918504749193,-1.,1.51805569591479));
#30817=CARTESIAN_POINT('Ctrl Pts',(0.89918504749193,1.,1.51805569591479));
#30818=CARTESIAN_POINT('Ctrl Pts',(0.905967409640498,-1.,1.52984849890434));
#30819=CARTESIAN_POINT('Ctrl Pts',(0.905967409640498,1.,1.52984849890434));
#30820=CARTESIAN_POINT('Ctrl Pts',(0.914375919046579,-1.,1.54440491152808));
#30821=CARTESIAN_POINT('Ctrl Pts',(0.914375919046579,1.,1.54440491152808));
#30822=CARTESIAN_POINT('Ctrl Pts',(0.923832188966322,-1.,1.56065988582509));
#30823=CARTESIAN_POINT('Ctrl Pts',(0.923832188966322,1.,1.56065988582509));
#30824=CARTESIAN_POINT('Ctrl Pts',(0.932246680128848,-1.,1.57499388385561));
#30825=CARTESIAN_POINT('Ctrl Pts',(0.932246680128848,1.,1.57499388385561));
#30826=CARTESIAN_POINT('Ctrl Pts',(0.939646377909319,-1.,1.58744937489796));
#30827=CARTESIAN_POINT('Ctrl Pts',(0.939646377909319,1.,1.58744937489796));
#30828=CARTESIAN_POINT('Ctrl Pts',(0.946078063325795,-1.,1.59810042045408));
#30829=CARTESIAN_POINT('Ctrl Pts',(0.946078063325795,1.,1.59810042045408));
#30830=CARTESIAN_POINT('Ctrl Pts',(0.951613284361247,-1.,1.60706069897794));
#30831=CARTESIAN_POINT('Ctrl Pts',(0.951613284361247,1.,1.60706069897794));
#30832=CARTESIAN_POINT('Ctrl Pts',(0.956354422921572,-1.,1.61449324337233));
#30833=CARTESIAN_POINT('Ctrl Pts',(0.956354422921572,1.,1.61449324337233));
#30834=CARTESIAN_POINT('Ctrl Pts',(0.960438326099958,-1.,1.62061638139929));
#30835=CARTESIAN_POINT('Ctrl Pts',(0.960438326099958,1.,1.62061638139929));
#30836=CARTESIAN_POINT('Ctrl Pts',(0.964046107037821,-1.,1.6257193066974));
#30837=CARTESIAN_POINT('Ctrl Pts',(0.964046107037821,1.,1.6257193066974));
#30838=CARTESIAN_POINT('Ctrl Pts',(0.967387853228041,-1.,1.63013849959083));
#30839=CARTESIAN_POINT('Ctrl Pts',(0.967387853228041,1.,1.63013849959083));
#30840=CARTESIAN_POINT('Ctrl Pts',(0.970669715996356,-1.,1.63420665729609));
#30841=CARTESIAN_POINT('Ctrl Pts',(0.970669715996356,1.,1.63420665729609));
#30842=CARTESIAN_POINT('Ctrl Pts',(0.974066058287501,-1.,1.63820952658157));
#30843=CARTESIAN_POINT('Ctrl Pts',(0.974066058287501,1.,1.63820952658157));
#30844=CARTESIAN_POINT('Ctrl Pts',(0.977689794120296,-1.,1.64233990826831));
#30845=CARTESIAN_POINT('Ctrl Pts',(0.977689794120296,1.,1.64233990826831));
#30846=CARTESIAN_POINT('Ctrl Pts',(0.981562530940574,-1.,1.64665139190834));
#30847=CARTESIAN_POINT('Ctrl Pts',(0.981562530940574,1.,1.64665139190834));
#30848=CARTESIAN_POINT('Ctrl Pts',(0.985642622921626,-1.,1.6511001661277));
#30849=CARTESIAN_POINT('Ctrl Pts',(0.985642622921626,1.,1.6511001661277));
#30850=CARTESIAN_POINT('Ctrl Pts',(0.98985562785445,-1.,1.65559044289746));
#30851=CARTESIAN_POINT('Ctrl Pts',(0.98985562785445,1.,1.65559044289746));
#30852=CARTESIAN_POINT('Ctrl Pts',(0.994121836661115,-1.,1.66001553809916));
#30853=CARTESIAN_POINT('Ctrl Pts',(0.994121836661115,1.,1.66001553809916));
#30854=CARTESIAN_POINT('Ctrl Pts',(0.998389654952317,-1.,1.66430758030304));
#30855=CARTESIAN_POINT('Ctrl Pts',(0.998389654952317,1.,1.66430758030304));
#30856=CARTESIAN_POINT('Ctrl Pts',(1.00265091003682,-1.,1.66846059277231));
#30857=CARTESIAN_POINT('Ctrl Pts',(1.00265091003682,1.,1.66846059277231));
#30858=CARTESIAN_POINT('Ctrl Pts',(1.00692206696387,-1.,1.67250335383248));
#30859=CARTESIAN_POINT('Ctrl Pts',(1.00692206696387,1.,1.67250335383248));
#30860=CARTESIAN_POINT('Ctrl Pts',(1.01123236493507,-1.,1.67648246776457));
#30861=CARTESIAN_POINT('Ctrl Pts',(1.01123236493507,1.,1.67648246776457));
#30862=CARTESIAN_POINT('Ctrl Pts',(1.01561026162786,-1.,1.6804428989482));
#30863=CARTESIAN_POINT('Ctrl Pts',(1.01561026162786,1.,1.6804428989482));
#30864=CARTESIAN_POINT('Ctrl Pts',(1.02006795074222,-1.,1.68440578021739));
#30865=CARTESIAN_POINT('Ctrl Pts',(1.02006795074222,1.,1.68440578021739));
#30866=CARTESIAN_POINT('Ctrl Pts',(1.02460180535272,-1.,1.68836910178475));
#30867=CARTESIAN_POINT('Ctrl Pts',(1.02460180535272,1.,1.68836910178475));
#30868=CARTESIAN_POINT('Ctrl Pts',(1.02919977579155,-1.,1.69231840863471));
#30869=CARTESIAN_POINT('Ctrl Pts',(1.02919977579155,1.,1.69231840863471));
#30870=CARTESIAN_POINT('Ctrl Pts',(1.03384646003587,-1.,1.69623414782769));
#30871=CARTESIAN_POINT('Ctrl Pts',(1.03384646003587,1.,1.69623414782769));
#30872=CARTESIAN_POINT('Ctrl Pts',(1.03852922490782,-1.,1.70010052930951));
#30873=CARTESIAN_POINT('Ctrl Pts',(1.03852922490782,1.,1.70010052930951));
#30874=CARTESIAN_POINT('Ctrl Pts',(1.04324363334546,-1.,1.70391338707969));
#30875=CARTESIAN_POINT('Ctrl Pts',(1.04324363334546,1.,1.70391338707969));
#30876=CARTESIAN_POINT('Ctrl Pts',(1.0479908540499,-1.,1.70767646263641));
#30877=CARTESIAN_POINT('Ctrl Pts',(1.0479908540499,1.,1.70767646263641));
#30878=CARTESIAN_POINT('Ctrl Pts',(1.05277517202853,-1.,1.71139783543986));
#30879=CARTESIAN_POINT('Ctrl Pts',(1.05277517202853,1.,1.71139783543986));
#30880=CARTESIAN_POINT('Ctrl Pts',(1.05760163192481,-1.,1.71508654427022));
#30881=CARTESIAN_POINT('Ctrl Pts',(1.05760163192481,1.,1.71508654427022));
#30882=CARTESIAN_POINT('Ctrl Pts',(1.06247324680649,-1.,1.71874858456908));
#30883=CARTESIAN_POINT('Ctrl Pts',(1.06247324680649,1.,1.71874858456908));
#30884=CARTESIAN_POINT('Ctrl Pts',(1.06738966975463,-1.,1.72238500928456));
#30885=CARTESIAN_POINT('Ctrl Pts',(1.06738966975463,1.,1.72238500928456));
#30886=CARTESIAN_POINT('Ctrl Pts',(1.07234866990252,-1.,1.72599406198489));
#30887=CARTESIAN_POINT('Ctrl Pts',(1.07234866990252,1.,1.72599406198489));
#30888=CARTESIAN_POINT('Ctrl Pts',(1.0773470373727,-1.,1.72957248977424));
#30889=CARTESIAN_POINT('Ctrl Pts',(1.0773470373727,1.,1.72957248977424));
#30890=CARTESIAN_POINT('Ctrl Pts',(1.08238162784749,-1.,1.73311705663407));
#30891=CARTESIAN_POINT('Ctrl Pts',(1.08238162784749,1.,1.73311705663407));
#30892=CARTESIAN_POINT('Ctrl Pts',(1.08745056285429,-1.,1.73662628326093));
#30893=CARTESIAN_POINT('Ctrl Pts',(1.08745056285429,1.,1.73662628326093));
#30894=CARTESIAN_POINT('Ctrl Pts',(1.09255329056496,-1.,1.74010053962252));
#30895=CARTESIAN_POINT('Ctrl Pts',(1.09255329056496,1.,1.74010053962252));
#30896=CARTESIAN_POINT('Ctrl Pts',(1.09768999241229,-1.,1.74354119236212));
#30897=CARTESIAN_POINT('Ctrl Pts',(1.09768999241229,1.,1.74354119236212));
#30898=CARTESIAN_POINT('Ctrl Pts',(1.10286118991144,-1.,1.74695004214924));
#30899=CARTESIAN_POINT('Ctrl Pts',(1.10286118991144,1.,1.74695004214924));
#30900=CARTESIAN_POINT('Ctrl Pts',(1.10806728183003,-1.,1.75032866075914));
#30901=CARTESIAN_POINT('Ctrl Pts',(1.10806728183003,1.,1.75032866075914));
#30902=CARTESIAN_POINT('Ctrl Pts',(1.11330807582542,-1.,1.75367772094617));
#30903=CARTESIAN_POINT('Ctrl Pts',(1.11330807582542,1.,1.75367772094617));
#30904=CARTESIAN_POINT('Ctrl Pts',(1.11858293216752,-1.,1.75699720772089));
#30905=CARTESIAN_POINT('Ctrl Pts',(1.11858293216752,1.,1.75699720772089));
#30906=CARTESIAN_POINT('Ctrl Pts',(1.12389096855078,-1.,1.76028671825084));
#30907=CARTESIAN_POINT('Ctrl Pts',(1.12389096855078,1.,1.76028671825084));
#30908=CARTESIAN_POINT('Ctrl Pts',(1.12923123555076,-1.,1.76354571966171));
#30909=CARTESIAN_POINT('Ctrl Pts',(1.12923123555076,1.,1.76354571966171));
#30910=CARTESIAN_POINT('Ctrl Pts',(1.13460291804634,-1.,1.76677384551883));
#30911=CARTESIAN_POINT('Ctrl Pts',(1.13460291804634,1.,1.76677384551883));
#30912=CARTESIAN_POINT('Ctrl Pts',(1.14000548337,-1.,1.76997111386806));
#30913=CARTESIAN_POINT('Ctrl Pts',(1.14000548337,1.,1.76997111386806));
#30914=CARTESIAN_POINT('Ctrl Pts',(1.14543858226948,-1.,1.77313777896234));
#30915=CARTESIAN_POINT('Ctrl Pts',(1.14543858226948,1.,1.77313777896234));
#30916=CARTESIAN_POINT('Ctrl Pts',(1.15090197841531,-1.,1.77627422557034));
#30917=CARTESIAN_POINT('Ctrl Pts',(1.15090197841531,1.,1.77627422557034));
#30918=CARTESIAN_POINT('Ctrl Pts',(1.15639547194689,-1.,1.77938085564261));
#30919=CARTESIAN_POINT('Ctrl Pts',(1.15639547194689,1.,1.77938085564261));
#30920=CARTESIAN_POINT('Ctrl Pts',(1.16191881298458,-1.,1.78245795880949));
#30921=CARTESIAN_POINT('Ctrl Pts',(1.16191881298458,1.,1.78245795880949));
#30922=CARTESIAN_POINT('Ctrl Pts',(1.16747166312239,-1.,1.78550566040349));
#30923=CARTESIAN_POINT('Ctrl Pts',(1.16747166312239,1.,1.78550566040349));
#30924=CARTESIAN_POINT('Ctrl Pts',(1.17305363177265,-1.,1.78852398877523));
#30925=CARTESIAN_POINT('Ctrl Pts',(1.17305363177265,1.,1.78852398877523));
#30926=CARTESIAN_POINT('Ctrl Pts',(1.17866429440781,-1.,1.79151291552646));
#30927=CARTESIAN_POINT('Ctrl Pts',(1.17866429440781,1.,1.79151291552646));
#30928=CARTESIAN_POINT('Ctrl Pts',(1.18430321697471,-1.,1.79447240321572));
#30929=CARTESIAN_POINT('Ctrl Pts',(1.18430321697471,1.,1.79447240321572));
#30930=CARTESIAN_POINT('Ctrl Pts',(1.1899699793456,-1.,1.79740245923649));
#30931=CARTESIAN_POINT('Ctrl Pts',(1.1899699793456,1.,1.79740245923649));
#30932=CARTESIAN_POINT('Ctrl Pts',(1.19566418930405,-1.,1.80030314370121));
#30933=CARTESIAN_POINT('Ctrl Pts',(1.19566418930405,1.,1.80030314370121));
#30934=CARTESIAN_POINT('Ctrl Pts',(1.2013854893912,-1.,1.8031745483882));
#30935=CARTESIAN_POINT('Ctrl Pts',(1.2013854893912,1.,1.8031745483882));
#30936=CARTESIAN_POINT('Ctrl Pts',(1.20713356605519,-1.,1.80601678480772));
#30937=CARTESIAN_POINT('Ctrl Pts',(1.20713356605519,1.,1.80601678480772));
#30938=CARTESIAN_POINT('Ctrl Pts',(1.2129081570818,-1.,1.80882996916931));
#30939=CARTESIAN_POINT('Ctrl Pts',(1.2129081570818,1.,1.80882996916931));
#30940=CARTESIAN_POINT('Ctrl Pts',(1.2187090610323,-1.,1.81161420806172));
#30941=CARTESIAN_POINT('Ctrl Pts',(1.2187090610323,1.,1.81161420806172));
#30942=CARTESIAN_POINT('Ctrl Pts',(1.22453613304507,-1.,1.81436959209778));
#30943=CARTESIAN_POINT('Ctrl Pts',(1.22453613304507,1.,1.81436959209778));
#30944=CARTESIAN_POINT('Ctrl Pts',(1.22921864890975,-1.,1.81655087183054));
#30945=CARTESIAN_POINT('Ctrl Pts',(1.22921864890975,1.,1.81655087183054));
#30946=CARTESIAN_POINT('Ctrl Pts',(1.23274224526804,-1.,1.81817389920914));
#30947=CARTESIAN_POINT('Ctrl Pts',(1.23274224526804,1.,1.81817389920914));
#30948=CARTESIAN_POINT('Ctrl Pts',(1.23509651170384,-1.,1.81925017193531));
#30949=CARTESIAN_POINT('Ctrl Pts',(1.23509651170384,1.,1.81925017193531));
#30950=CARTESIAN_POINT('Ctrl Pts',(1.23627494547115,-1.,1.81978687191668));
#30951=CARTESIAN_POINT('Ctrl Pts',(1.23627494547115,1.,1.81978687191668));
#30952=CARTESIAN_POINT('',(0.892032620296855,1.,1.5055822144029));
#30953=CARTESIAN_POINT('Ctrl Pts',(0.892032620296855,1.,1.5055822144029));
#30954=CARTESIAN_POINT('Ctrl Pts',(0.894452006967538,1.,1.50980486807181));
#30955=CARTESIAN_POINT('Ctrl Pts',(0.89918504749193,1.,1.51805569591479));
#30956=CARTESIAN_POINT('Ctrl Pts',(0.905967409640498,1.,1.52984849890434));
#30957=CARTESIAN_POINT('Ctrl Pts',(0.914375919046579,1.,1.54440491152808));
#30958=CARTESIAN_POINT('Ctrl Pts',(0.923832188966322,1.,1.56065988582509));
#30959=CARTESIAN_POINT('Ctrl Pts',(0.932246680128848,1.,1.57499388385561));
#30960=CARTESIAN_POINT('Ctrl Pts',(0.939646377909319,1.,1.58744937489796));
#30961=CARTESIAN_POINT('Ctrl Pts',(0.946078063325795,1.,1.59810042045408));
#30962=CARTESIAN_POINT('Ctrl Pts',(0.951613284361247,1.,1.60706069897794));
#30963=CARTESIAN_POINT('Ctrl Pts',(0.956354422921572,1.,1.61449324337233));
#30964=CARTESIAN_POINT('Ctrl Pts',(0.960438326099958,1.,1.62061638139929));
#30965=CARTESIAN_POINT('Ctrl Pts',(0.964046107037821,1.,1.6257193066974));
#30966=CARTESIAN_POINT('Ctrl Pts',(0.967387853228041,1.,1.63013849959083));
#30967=CARTESIAN_POINT('Ctrl Pts',(0.970669715996356,1.,1.63420665729609));
#30968=CARTESIAN_POINT('Ctrl Pts',(0.974066058287501,1.,1.63820952658157));
#30969=CARTESIAN_POINT('Ctrl Pts',(0.977689794120296,1.,1.64233990826831));
#30970=CARTESIAN_POINT('Ctrl Pts',(0.981562530940574,1.,1.64665139190834));
#30971=CARTESIAN_POINT('Ctrl Pts',(0.985642622921626,1.,1.6511001661277));
#30972=CARTESIAN_POINT('Ctrl Pts',(0.98985562785445,1.,1.65559044289746));
#30973=CARTESIAN_POINT('Ctrl Pts',(0.994121836661115,1.,1.66001553809916));
#30974=CARTESIAN_POINT('Ctrl Pts',(0.998389654952317,1.,1.66430758030304));
#30975=CARTESIAN_POINT('Ctrl Pts',(1.00265091003682,1.,1.66846059277231));
#30976=CARTESIAN_POINT('Ctrl Pts',(1.00692206696387,1.,1.67250335383248));
#30977=CARTESIAN_POINT('Ctrl Pts',(1.01123236493507,1.,1.67648246776457));
#30978=CARTESIAN_POINT('Ctrl Pts',(1.01561026162786,1.,1.6804428989482));
#30979=CARTESIAN_POINT('Ctrl Pts',(1.02006795074222,1.,1.68440578021739));
#30980=CARTESIAN_POINT('Ctrl Pts',(1.02460180535272,1.,1.68836910178475));
#30981=CARTESIAN_POINT('Ctrl Pts',(1.02919977579155,1.,1.69231840863471));
#30982=CARTESIAN_POINT('Ctrl Pts',(1.03384646003587,1.,1.69623414782769));
#30983=CARTESIAN_POINT('Ctrl Pts',(1.03852922490782,1.,1.70010052930951));
#30984=CARTESIAN_POINT('Ctrl Pts',(1.04324363334546,1.,1.70391338707969));
#30985=CARTESIAN_POINT('Ctrl Pts',(1.0479908540499,1.,1.70767646263641));
#30986=CARTESIAN_POINT('Ctrl Pts',(1.05277517202853,1.,1.71139783543986));
#30987=CARTESIAN_POINT('Ctrl Pts',(1.05760163192481,1.,1.71508654427022));
#30988=CARTESIAN_POINT('Ctrl Pts',(1.06247324680649,1.,1.71874858456908));
#30989=CARTESIAN_POINT('Ctrl Pts',(1.06738966975463,1.,1.72238500928456));
#30990=CARTESIAN_POINT('Ctrl Pts',(1.07234866990252,1.,1.72599406198489));
#30991=CARTESIAN_POINT('Ctrl Pts',(1.0773470373727,1.,1.72957248977424));
#30992=CARTESIAN_POINT('Ctrl Pts',(1.08238162784749,1.,1.73311705663407));
#30993=CARTESIAN_POINT('Ctrl Pts',(1.08745056285429,1.,1.73662628326093));
#30994=CARTESIAN_POINT('Ctrl Pts',(1.09255329056496,1.,1.74010053962252));
#30995=CARTESIAN_POINT('Ctrl Pts',(1.09768999241229,1.,1.74354119236212));
#30996=CARTESIAN_POINT('Ctrl Pts',(1.10286118991144,1.,1.74695004214924));
#30997=CARTESIAN_POINT('Ctrl Pts',(1.10806728183003,1.,1.75032866075914));
#30998=CARTESIAN_POINT('Ctrl Pts',(1.11330807582542,1.,1.75367772094617));
#30999=CARTESIAN_POINT('Ctrl Pts',(1.11858293216752,1.,1.75699720772089));
#31000=CARTESIAN_POINT('Ctrl Pts',(1.12389096855078,1.,1.76028671825084));
#31001=CARTESIAN_POINT('Ctrl Pts',(1.12923123555076,1.,1.76354571966171));
#31002=CARTESIAN_POINT('Ctrl Pts',(1.13460291804634,1.,1.76677384551883));
#31003=CARTESIAN_POINT('Ctrl Pts',(1.14000548337,1.,1.76997111386806));
#31004=CARTESIAN_POINT('Ctrl Pts',(1.14543858226948,1.,1.77313777896234));
#31005=CARTESIAN_POINT('Ctrl Pts',(1.15090197841531,1.,1.77627422557034));
#31006=CARTESIAN_POINT('Ctrl Pts',(1.15639547194689,1.,1.77938085564261));
#31007=CARTESIAN_POINT('Ctrl Pts',(1.16191881298458,1.,1.78245795880949));
#31008=CARTESIAN_POINT('Ctrl Pts',(1.16747166312239,1.,1.78550566040349));
#31009=CARTESIAN_POINT('Ctrl Pts',(1.17305363177265,1.,1.78852398877523));
#31010=CARTESIAN_POINT('Ctrl Pts',(1.17866429440781,1.,1.79151291552646));
#31011=CARTESIAN_POINT('Ctrl Pts',(1.18430321697471,1.,1.79447240321572));
#31012=CARTESIAN_POINT('Ctrl Pts',(1.1899699793456,1.,1.79740245923649));
#31013=CARTESIAN_POINT('Ctrl Pts',(1.19566418930405,1.,1.80030314370121));
#31014=CARTESIAN_POINT('Ctrl Pts',(1.2013854893912,1.,1.8031745483882));
#31015=CARTESIAN_POINT('Ctrl Pts',(1.20713356605519,1.,1.80601678480772));
#31016=CARTESIAN_POINT('Ctrl Pts',(1.2129081570818,1.,1.80882996916931));
#31017=CARTESIAN_POINT('Ctrl Pts',(1.2187090610323,1.,1.81161420806172));
#31018=CARTESIAN_POINT('Ctrl Pts',(1.22453613304507,1.,1.81436959209778));
#31019=CARTESIAN_POINT('Ctrl Pts',(1.22921864890975,1.,1.81655087183054));
#31020=CARTESIAN_POINT('Ctrl Pts',(1.23274224526804,1.,1.81817389920914));
#31021=CARTESIAN_POINT('Ctrl Pts',(1.23509651170384,1.,1.81925017193531));
#31022=CARTESIAN_POINT('Ctrl Pts',(1.23627494547115,1.,1.81978687191668));
#31023=CARTESIAN_POINT('',(0.892032620296854,0.,1.5055822144029));
#31024=CARTESIAN_POINT('Origin',(0.,0.,0.));
#31025=CARTESIAN_POINT('',(0.693717979106305,1.,1.60662857109684));
#31026=CARTESIAN_POINT('Origin',(0.,1.,0.));
#31027=CARTESIAN_POINT('',(0.693717979106305,0.,1.60662857109684));
#31028=CARTESIAN_POINT('Ctrl Pts',(0.7455743247944,-1.,2.0698113262342));
#31029=CARTESIAN_POINT('Ctrl Pts',(0.7455743247944,1.,2.0698113262342));
#31030=CARTESIAN_POINT('Ctrl Pts',(0.745832791378367,-1.,2.06854248895728));
#31031=CARTESIAN_POINT('Ctrl Pts',(0.745832791378367,1.,2.06854248895728));
#31032=CARTESIAN_POINT('Ctrl Pts',(0.7463458715442,-1.,2.06600523016815));
#31033=CARTESIAN_POINT('Ctrl Pts',(0.7463458715442,1.,2.06600523016815));
#31034=CARTESIAN_POINT('Ctrl Pts',(0.747103932787919,-1.,2.06220058927826));
#31035=CARTESIAN_POINT('Ctrl Pts',(0.747103932787919,1.,2.06220058927826));
#31036=CARTESIAN_POINT('Ctrl Pts',(0.748091554183802,-1.,2.05713023031007));
#31037=CARTESIAN_POINT('Ctrl Pts',(0.748091554183802,1.,2.05713023031007));
#31038=CARTESIAN_POINT('Ctrl Pts',(0.749287468665046,-1.,2.05079645592154));
#31039=CARTESIAN_POINT('Ctrl Pts',(0.749287468665046,1.,2.05079645592154));
#31040=CARTESIAN_POINT('Ctrl Pts',(0.750444657875575,-1.,2.04446689147979));
#31041=CARTESIAN_POINT('Ctrl Pts',(0.750444657875575,1.,2.04446689147979));
#31042=CARTESIAN_POINT('Ctrl Pts',(0.751562963361115,-1.,2.03814160092099));
#31043=CARTESIAN_POINT('Ctrl Pts',(0.751562963361115,1.,2.03814160092099));
#31044=CARTESIAN_POINT('Ctrl Pts',(0.75264218048721,-1.,2.03182068456221));
#31045=CARTESIAN_POINT('Ctrl Pts',(0.75264218048721,1.,2.03182068456221));
#31046=CARTESIAN_POINT('Ctrl Pts',(0.753682061112768,-1.,2.02550428623313));
#31047=CARTESIAN_POINT('Ctrl Pts',(0.753682061112768,1.,2.02550428623313));
#31048=CARTESIAN_POINT('Ctrl Pts',(0.754682330722816,-1.,2.01919259405809));
#31049=CARTESIAN_POINT('Ctrl Pts',(0.754682330722816,1.,2.01919259405809));
#31050=CARTESIAN_POINT('Ctrl Pts',(0.755642704957865,-1.,2.01288584328084));
#31051=CARTESIAN_POINT('Ctrl Pts',(0.755642704957865,1.,2.01288584328084));
#31052=CARTESIAN_POINT('Ctrl Pts',(0.75656290464667,-1.,2.0065843158773));
#31053=CARTESIAN_POINT('Ctrl Pts',(0.75656290464667,1.,2.0065843158773));
#31054=CARTESIAN_POINT('Ctrl Pts',(0.757442676862724,-1.,2.00028834739178));
#31055=CARTESIAN_POINT('Ctrl Pts',(0.757442676862724,1.,2.00028834739178));
#31056=CARTESIAN_POINT('Ctrl Pts',(0.758281796766761,-1.,1.99399831098817));
#31057=CARTESIAN_POINT('Ctrl Pts',(0.758281796766761,1.,1.99399831098817));
#31058=CARTESIAN_POINT('Ctrl Pts',(0.759080037802488,-1.,1.98771456680874));
#31059=CARTESIAN_POINT('Ctrl Pts',(0.759080037802488,1.,1.98771456680874));
#31060=CARTESIAN_POINT('Ctrl Pts',(0.75983714745219,-1.,1.98143741418172));
#31061=CARTESIAN_POINT('Ctrl Pts',(0.75983714745219,1.,1.98143741418172));
#31062=CARTESIAN_POINT('Ctrl Pts',(0.760552825409757,-1.,1.97516705321494));
#31063=CARTESIAN_POINT('Ctrl Pts',(0.760552825409757,1.,1.97516705321494));
#31064=CARTESIAN_POINT('Ctrl Pts',(0.76122669048382,-1.,1.96890351582499));
#31065=CARTESIAN_POINT('Ctrl Pts',(0.76122669048382,1.,1.96890351582499));
#31066=CARTESIAN_POINT('Ctrl Pts',(0.761858300014423,-1.,1.96264672744186));
#31067=CARTESIAN_POINT('Ctrl Pts',(0.761858300014423,1.,1.96264672744186));
#31068=CARTESIAN_POINT('Ctrl Pts',(0.762447203806178,-1.,1.95639665309869));
#31069=CARTESIAN_POINT('Ctrl Pts',(0.762447203806178,1.,1.95639665309869));
#31070=CARTESIAN_POINT('Ctrl Pts',(0.762992990878769,-1.,1.95015342590024));
#31071=CARTESIAN_POINT('Ctrl Pts',(0.762992990878769,1.,1.95015342590024));
#31072=CARTESIAN_POINT('Ctrl Pts',(0.763495333538629,-1.,1.9439174661764));
#31073=CARTESIAN_POINT('Ctrl Pts',(0.763495333538629,1.,1.9439174661764));
#31074=CARTESIAN_POINT('Ctrl Pts',(0.763954049121458,-1.,1.93768964875886));
#31075=CARTESIAN_POINT('Ctrl Pts',(0.763954049121458,1.,1.93768964875886));
#31076=CARTESIAN_POINT('Ctrl Pts',(0.76436901067394,-1.,1.93147105496382));
#31077=CARTESIAN_POINT('Ctrl Pts',(0.76436901067394,1.,1.93147105496382));
#31078=CARTESIAN_POINT('Ctrl Pts',(0.764740025488211,-1.,1.92526263537048));
#31079=CARTESIAN_POINT('Ctrl Pts',(0.764740025488211,1.,1.92526263537048));
#31080=CARTESIAN_POINT('Ctrl Pts',(0.765066729667088,-1.,1.91906491634196));
#31081=CARTESIAN_POINT('Ctrl Pts',(0.765066729667088,1.,1.91906491634196));
#31082=CARTESIAN_POINT('Ctrl Pts',(0.765348465884722,-1.,1.91287765805169));
#31083=CARTESIAN_POINT('Ctrl Pts',(0.765348465884722,1.,1.91287765805169));
#31084=CARTESIAN_POINT('Ctrl Pts',(0.765584196937919,-1.,1.90669961402356));
#31085=CARTESIAN_POINT('Ctrl Pts',(0.765584196937919,1.,1.90669961402356));
#31086=CARTESIAN_POINT('Ctrl Pts',(0.765772772593386,-1.,1.90052930393596));
#31087=CARTESIAN_POINT('Ctrl Pts',(0.765772772593386,1.,1.90052930393596));
#31088=CARTESIAN_POINT('Ctrl Pts',(0.765913193856978,-1.,1.89436577771388));
#31089=CARTESIAN_POINT('Ctrl Pts',(0.765913193856978,1.,1.89436577771388));
#31090=CARTESIAN_POINT('Ctrl Pts',(0.766004837062091,-1.,1.88820926433409));
#31091=CARTESIAN_POINT('Ctrl Pts',(0.766004837062091,1.,1.88820926433409));
#31092=CARTESIAN_POINT('Ctrl Pts',(0.766047794851864,-1.,1.88206215302561));
#31093=CARTESIAN_POINT('Ctrl Pts',(0.766047794851864,1.,1.88206215302561));
#31094=CARTESIAN_POINT('Ctrl Pts',(0.766042837036744,-1.,1.87592888967883));
#31095=CARTESIAN_POINT('Ctrl Pts',(0.766042837036744,1.,1.87592888967883));
#31096=CARTESIAN_POINT('Ctrl Pts',(0.765990708546091,-1.,1.86981398314341));
#31097=CARTESIAN_POINT('Ctrl Pts',(0.765990708546091,1.,1.86981398314341));
#31098=CARTESIAN_POINT('Ctrl Pts',(0.765891519092547,-1.,1.86372027063312));
#31099=CARTESIAN_POINT('Ctrl Pts',(0.765891519092547,1.,1.86372027063312));
#31100=CARTESIAN_POINT('Ctrl Pts',(0.765744212909318,-1.,1.85764741390394));
#31101=CARTESIAN_POINT('Ctrl Pts',(0.765744212909318,1.,1.85764741390394));
#31102=CARTESIAN_POINT('Ctrl Pts',(0.765545710619062,-1.,1.85158945130063));
#31103=CARTESIAN_POINT('Ctrl Pts',(0.765545710619062,1.,1.85158945130063));
#31104=CARTESIAN_POINT('Ctrl Pts',(0.765291664862029,-1.,1.84553698875924));
#31105=CARTESIAN_POINT('Ctrl Pts',(0.765291664862029,1.,1.84553698875924));
#31106=CARTESIAN_POINT('Ctrl Pts',(0.764978057881737,-1.,1.83948181064835));
#31107=CARTESIAN_POINT('Ctrl Pts',(0.764978057881737,1.,1.83948181064835));
#31108=CARTESIAN_POINT('Ctrl Pts',(0.764602549687853,-1.,1.83342077227142));
#31109=CARTESIAN_POINT('Ctrl Pts',(0.764602549687853,1.,1.83342077227142));
#31110=CARTESIAN_POINT('Ctrl Pts',(0.764165902605995,-1.,1.82735991200065));
#31111=CARTESIAN_POINT('Ctrl Pts',(0.764165902605995,1.,1.82735991200065));
#31112=CARTESIAN_POINT('Ctrl Pts',(0.763673465462726,-1.,1.82131873145266));
#31113=CARTESIAN_POINT('Ctrl Pts',(0.763673465462726,1.,1.82131873145266));
#31114=CARTESIAN_POINT('Ctrl Pts',(0.763132003836634,-1.,1.8153211840553));
#31115=CARTESIAN_POINT('Ctrl Pts',(0.763132003836634,1.,1.8153211840553));
#31116=CARTESIAN_POINT('Ctrl Pts',(0.762546129463938,-1.,1.80938551463965));
#31117=CARTESIAN_POINT('Ctrl Pts',(0.762546129463938,1.,1.80938551463965));
#31118=CARTESIAN_POINT('Ctrl Pts',(0.761915336443547,-1.,1.80351583877342));
#31119=CARTESIAN_POINT('Ctrl Pts',(0.761915336443547,1.,1.80351583877342));
#31120=CARTESIAN_POINT('Ctrl Pts',(0.761229695230558,-1.,1.79768986997783));
#31121=CARTESIAN_POINT('Ctrl Pts',(0.761229695230558,1.,1.79768986997783));
#31122=CARTESIAN_POINT('Ctrl Pts',(0.760469555880749,-1.,1.7918581561088));
#31123=CARTESIAN_POINT('Ctrl Pts',(0.760469555880749,1.,1.7918581561088));
#31124=CARTESIAN_POINT('Ctrl Pts',(0.759614401110189,-1.,1.78596964884604));
#31125=CARTESIAN_POINT('Ctrl Pts',(0.759614401110189,1.,1.78596964884604));
#31126=CARTESIAN_POINT('Ctrl Pts',(0.758650626677518,-1.,1.77999411220945));
#31127=CARTESIAN_POINT('Ctrl Pts',(0.758650626677518,1.,1.77999411220945));
#31128=CARTESIAN_POINT('Ctrl Pts',(0.757578264077028,-1.,1.77394167108292));
#31129=CARTESIAN_POINT('Ctrl Pts',(0.757578264077028,1.,1.77394167108292));
#31130=CARTESIAN_POINT('Ctrl Pts',(0.75642189602781,-1.,1.76789396002998));
#31131=CARTESIAN_POINT('Ctrl Pts',(0.75642189602781,1.,1.76789396002998));
#31132=CARTESIAN_POINT('Ctrl Pts',(0.755220979974461,-1.,1.76197817240128));
#31133=CARTESIAN_POINT('Ctrl Pts',(0.755220979974461,1.,1.76197817240128));
#31134=CARTESIAN_POINT('Ctrl Pts',(0.754009254027828,-1.,1.75631083600019));
#31135=CARTESIAN_POINT('Ctrl Pts',(0.754009254027828,1.,1.75631083600019));
#31136=CARTESIAN_POINT('Ctrl Pts',(0.752797683531314,-1.,1.75095139468794));
#31137=CARTESIAN_POINT('Ctrl Pts',(0.752797683531314,1.,1.75095139468794));
#31138=CARTESIAN_POINT('Ctrl Pts',(0.751555614164482,-1.,1.74585086852502));
#31139=CARTESIAN_POINT('Ctrl Pts',(0.751555614164482,1.,1.74585086852502));
#31140=CARTESIAN_POINT('Ctrl Pts',(0.750193435981249,-1.,1.74080458267114));
#31141=CARTESIAN_POINT('Ctrl Pts',(0.750193435981249,1.,1.74080458267114));
#31142=CARTESIAN_POINT('Ctrl Pts',(0.74858246295687,-1.,1.7355035168033));
#31143=CARTESIAN_POINT('Ctrl Pts',(0.74858246295687,1.,1.7355035168033));
#31144=CARTESIAN_POINT('Ctrl Pts',(0.746574710097752,-1.,1.72958533647714));
#31145=CARTESIAN_POINT('Ctrl Pts',(0.746574710097752,1.,1.72958533647714));
#31146=CARTESIAN_POINT('Ctrl Pts',(0.744021445433093,-1.,1.72268229916769));
#31147=CARTESIAN_POINT('Ctrl Pts',(0.744021445433093,1.,1.72268229916769));
#31148=CARTESIAN_POINT('Ctrl Pts',(0.74079516202821,-1.,1.71447789751001));
#31149=CARTESIAN_POINT('Ctrl Pts',(0.74079516202821,1.,1.71447789751001));
#31150=CARTESIAN_POINT('Ctrl Pts',(0.736799665716932,-1.,1.70473309004249));
#31151=CARTESIAN_POINT('Ctrl Pts',(0.736799665716932,1.,1.70473309004249));
#31152=CARTESIAN_POINT('Ctrl Pts',(0.731963238685357,-1.,1.69326921972915));
#31153=CARTESIAN_POINT('Ctrl Pts',(0.731963238685357,1.,1.69326921972915));
#31154=CARTESIAN_POINT('Ctrl Pts',(0.726235967982445,-1.,1.67996158451922));
#31155=CARTESIAN_POINT('Ctrl Pts',(0.726235967982445,1.,1.67996158451922));
#31156=CARTESIAN_POINT('Ctrl Pts',(0.719585433787949,-1.,1.66472880551777));
#31157=CARTESIAN_POINT('Ctrl Pts',(0.719585433787949,1.,1.66472880551777));
#31158=CARTESIAN_POINT('Ctrl Pts',(0.711993139340447,-1.,1.64752408828442));
#31159=CARTESIAN_POINT('Ctrl Pts',(0.711993139340447,1.,1.64752408828442));
#31160=CARTESIAN_POINT('Ctrl Pts',(0.705159151977294,-1.,1.6321654166204));
#31161=CARTESIAN_POINT('Ctrl Pts',(0.705159151977294,1.,1.6321654166204));
#31162=CARTESIAN_POINT('Ctrl Pts',(0.699605146398836,-1.,1.61974673471117));
#31163=CARTESIAN_POINT('Ctrl Pts',(0.699605146398836,1.,1.61974673471117));
#31164=CARTESIAN_POINT('Ctrl Pts',(0.69571209787897,-1.,1.61106790957619));
#31165=CARTESIAN_POINT('Ctrl Pts',(0.69571209787897,1.,1.61106790957619));
#31166=CARTESIAN_POINT('Ctrl Pts',(0.693717979106305,-1.,1.60662857109684));
#31167=CARTESIAN_POINT('Ctrl Pts',(0.693717979106305,1.,1.60662857109684));
#31168=CARTESIAN_POINT('',(0.7455743247944,1.,2.0698113262342));
#31169=CARTESIAN_POINT('Ctrl Pts',(0.7455743247944,1.,2.0698113262342));
#31170=CARTESIAN_POINT('Ctrl Pts',(0.745832791378367,1.,2.06854248895728));
#31171=CARTESIAN_POINT('Ctrl Pts',(0.7463458715442,1.,2.06600523016815));
#31172=CARTESIAN_POINT('Ctrl Pts',(0.747103932787919,1.,2.06220058927826));
#31173=CARTESIAN_POINT('Ctrl Pts',(0.748091554183802,1.,2.05713023031007));
#31174=CARTESIAN_POINT('Ctrl Pts',(0.749287468665046,1.,2.05079645592154));
#31175=CARTESIAN_POINT('Ctrl Pts',(0.750444657875575,1.,2.04446689147979));
#31176=CARTESIAN_POINT('Ctrl Pts',(0.751562963361115,1.,2.03814160092099));
#31177=CARTESIAN_POINT('Ctrl Pts',(0.75264218048721,1.,2.03182068456221));
#31178=CARTESIAN_POINT('Ctrl Pts',(0.753682061112768,1.,2.02550428623313));
#31179=CARTESIAN_POINT('Ctrl Pts',(0.754682330722816,1.,2.01919259405809));
#31180=CARTESIAN_POINT('Ctrl Pts',(0.755642704957865,1.,2.01288584328084));
#31181=CARTESIAN_POINT('Ctrl Pts',(0.75656290464667,1.,2.0065843158773));
#31182=CARTESIAN_POINT('Ctrl Pts',(0.757442676862724,1.,2.00028834739178));
#31183=CARTESIAN_POINT('Ctrl Pts',(0.758281796766761,1.,1.99399831098817));
#31184=CARTESIAN_POINT('Ctrl Pts',(0.759080037802488,1.,1.98771456680874));
#31185=CARTESIAN_POINT('Ctrl Pts',(0.75983714745219,1.,1.98143741418172));
#31186=CARTESIAN_POINT('Ctrl Pts',(0.760552825409757,1.,1.97516705321494));
#31187=CARTESIAN_POINT('Ctrl Pts',(0.76122669048382,1.,1.96890351582499));
#31188=CARTESIAN_POINT('Ctrl Pts',(0.761858300014423,1.,1.96264672744186));
#31189=CARTESIAN_POINT('Ctrl Pts',(0.762447203806178,1.,1.95639665309869));
#31190=CARTESIAN_POINT('Ctrl Pts',(0.762992990878769,1.,1.95015342590024));
#31191=CARTESIAN_POINT('Ctrl Pts',(0.763495333538629,1.,1.9439174661764));
#31192=CARTESIAN_POINT('Ctrl Pts',(0.763954049121458,1.,1.93768964875886));
#31193=CARTESIAN_POINT('Ctrl Pts',(0.76436901067394,1.,1.93147105496382));
#31194=CARTESIAN_POINT('Ctrl Pts',(0.764740025488211,1.,1.92526263537048));
#31195=CARTESIAN_POINT('Ctrl Pts',(0.765066729667088,1.,1.91906491634196));
#31196=CARTESIAN_POINT('Ctrl Pts',(0.765348465884722,1.,1.91287765805169));
#31197=CARTESIAN_POINT('Ctrl Pts',(0.765584196937919,1.,1.90669961402356));
#31198=CARTESIAN_POINT('Ctrl Pts',(0.765772772593386,1.,1.90052930393596));
#31199=CARTESIAN_POINT('Ctrl Pts',(0.765913193856978,1.,1.89436577771388));
#31200=CARTESIAN_POINT('Ctrl Pts',(0.766004837062091,1.,1.88820926433409));
#31201=CARTESIAN_POINT('Ctrl Pts',(0.766047794851864,1.,1.88206215302561));
#31202=CARTESIAN_POINT('Ctrl Pts',(0.766042837036744,1.,1.87592888967883));
#31203=CARTESIAN_POINT('Ctrl Pts',(0.765990708546091,1.,1.86981398314341));
#31204=CARTESIAN_POINT('Ctrl Pts',(0.765891519092547,1.,1.86372027063312));
#31205=CARTESIAN_POINT('Ctrl Pts',(0.765744212909318,1.,1.85764741390394));
#31206=CARTESIAN_POINT('Ctrl Pts',(0.765545710619062,1.,1.85158945130063));
#31207=CARTESIAN_POINT('Ctrl Pts',(0.765291664862029,1.,1.84553698875924));
#31208=CARTESIAN_POINT('Ctrl Pts',(0.764978057881737,1.,1.83948181064835));
#31209=CARTESIAN_POINT('Ctrl Pts',(0.764602549687853,1.,1.83342077227142));
#31210=CARTESIAN_POINT('Ctrl Pts',(0.764165902605995,1.,1.82735991200065));
#31211=CARTESIAN_POINT('Ctrl Pts',(0.763673465462726,1.,1.82131873145266));
#31212=CARTESIAN_POINT('Ctrl Pts',(0.763132003836634,1.,1.8153211840553));
#31213=CARTESIAN_POINT('Ctrl Pts',(0.762546129463938,1.,1.80938551463965));
#31214=CARTESIAN_POINT('Ctrl Pts',(0.761915336443547,1.,1.80351583877342));
#31215=CARTESIAN_POINT('Ctrl Pts',(0.761229695230558,1.,1.79768986997783));
#31216=CARTESIAN_POINT('Ctrl Pts',(0.760469555880749,1.,1.7918581561088));
#31217=CARTESIAN_POINT('Ctrl Pts',(0.759614401110189,1.,1.78596964884604));
#31218=CARTESIAN_POINT('Ctrl Pts',(0.758650626677518,1.,1.77999411220945));
#31219=CARTESIAN_POINT('Ctrl Pts',(0.757578264077028,1.,1.77394167108292));
#31220=CARTESIAN_POINT('Ctrl Pts',(0.75642189602781,1.,1.76789396002998));
#31221=CARTESIAN_POINT('Ctrl Pts',(0.755220979974461,1.,1.76197817240128));
#31222=CARTESIAN_POINT('Ctrl Pts',(0.754009254027828,1.,1.75631083600019));
#31223=CARTESIAN_POINT('Ctrl Pts',(0.752797683531314,1.,1.75095139468794));
#31224=CARTESIAN_POINT('Ctrl Pts',(0.751555614164482,1.,1.74585086852502));
#31225=CARTESIAN_POINT('Ctrl Pts',(0.750193435981249,1.,1.74080458267114));
#31226=CARTESIAN_POINT('Ctrl Pts',(0.74858246295687,1.,1.7355035168033));
#31227=CARTESIAN_POINT('Ctrl Pts',(0.746574710097752,1.,1.72958533647714));
#31228=CARTESIAN_POINT('Ctrl Pts',(0.744021445433093,1.,1.72268229916769));
#31229=CARTESIAN_POINT('Ctrl Pts',(0.74079516202821,1.,1.71447789751001));
#31230=CARTESIAN_POINT('Ctrl Pts',(0.736799665716932,1.,1.70473309004249));
#31231=CARTESIAN_POINT('Ctrl Pts',(0.731963238685357,1.,1.69326921972915));
#31232=CARTESIAN_POINT('Ctrl Pts',(0.726235967982445,1.,1.67996158451922));
#31233=CARTESIAN_POINT('Ctrl Pts',(0.719585433787949,1.,1.66472880551777));
#31234=CARTESIAN_POINT('Ctrl Pts',(0.711993139340447,1.,1.64752408828442));
#31235=CARTESIAN_POINT('Ctrl Pts',(0.705159151977294,1.,1.6321654166204));
#31236=CARTESIAN_POINT('Ctrl Pts',(0.699605146398836,1.,1.61974673471117));
#31237=CARTESIAN_POINT('Ctrl Pts',(0.69571209787897,1.,1.61106790957619));
#31238=CARTESIAN_POINT('Ctrl Pts',(0.693717979106305,1.,1.60662857109684));
#31239=CARTESIAN_POINT('',(0.7455743247944,0.,2.0698113262342));
#31240=CARTESIAN_POINT('Origin',(0.61342227326009,0.,2.11275013067528));
#31241=CARTESIAN_POINT('',(0.61342227326009,1.,2.11275013067528));
#31242=CARTESIAN_POINT('',(0.7455743247944,1.,2.0698113262342));
#31243=CARTESIAN_POINT('',(0.61342227326009,0.,2.11275013067528));
#31244=CARTESIAN_POINT('Ctrl Pts',(0.383122945602004,-1.,1.7075470150345));
#31245=CARTESIAN_POINT('Ctrl Pts',(0.383122945602004,1.,1.7075470150345));
#31246=CARTESIAN_POINT('Ctrl Pts',(0.384119047315541,-1.,1.71231062891958));
#31247=CARTESIAN_POINT('Ctrl Pts',(0.384119047315541,1.,1.71231062891958));
#31248=CARTESIAN_POINT('Ctrl Pts',(0.38607079032701,-1.,1.72162022246158));
#31249=CARTESIAN_POINT('Ctrl Pts',(0.38607079032701,1.,1.72162022246158));
#31250=CARTESIAN_POINT('Ctrl Pts',(0.388877023509191,-1.,1.7349317097561));
#31251=CARTESIAN_POINT('Ctrl Pts',(0.388877023509191,1.,1.7349317097561));
#31252=CARTESIAN_POINT('Ctrl Pts',(0.392375812294307,-1.,1.75137405313962));
#31253=CARTESIAN_POINT('Ctrl Pts',(0.392375812294307,1.,1.75137405313962));
#31254=CARTESIAN_POINT('Ctrl Pts',(0.39634619612042,-1.,1.7697556004756));
#31255=CARTESIAN_POINT('Ctrl Pts',(0.39634619612042,1.,1.7697556004756));
#31256=CARTESIAN_POINT('Ctrl Pts',(0.39991940378308,-1.,1.78598826347533));
#31257=CARTESIAN_POINT('Ctrl Pts',(0.39991940378308,1.,1.78598826347533));
#31258=CARTESIAN_POINT('Ctrl Pts',(0.403107976170441,-1.,1.80012077176221));
#31259=CARTESIAN_POINT('Ctrl Pts',(0.403107976170441,1.,1.80012077176221));
#31260=CARTESIAN_POINT('Ctrl Pts',(0.405933518411838,-1.,1.81223801813988));
#31261=CARTESIAN_POINT('Ctrl Pts',(0.405933518411838,1.,1.81223801813988));
#31262=CARTESIAN_POINT('Ctrl Pts',(0.408428948108533,-1.,1.8224702267854));
#31263=CARTESIAN_POINT('Ctrl Pts',(0.408428948108533,1.,1.8224702267854));
#31264=CARTESIAN_POINT('Ctrl Pts',(0.410641256301674,-1.,1.83100408895216));
#31265=CARTESIAN_POINT('Ctrl Pts',(0.410641256301674,1.,1.83100408895216));
#31266=CARTESIAN_POINT('Ctrl Pts',(0.412633125322161,-1.,1.83808953475839));
#31267=CARTESIAN_POINT('Ctrl Pts',(0.412633125322161,1.,1.83808953475839));
#31268=CARTESIAN_POINT('Ctrl Pts',(0.41448743825434,-1.,1.8440575707371));
#31269=CARTESIAN_POINT('Ctrl Pts',(0.41448743825434,1.,1.8440575707371));
#31270=CARTESIAN_POINT('Ctrl Pts',(0.416300022038864,-1.,1.84929312929882));
#31271=CARTESIAN_POINT('Ctrl Pts',(0.416300022038864,1.,1.84929312929882));
#31272=CARTESIAN_POINT('Ctrl Pts',(0.418164129143534,-1.,1.85417632856234));
#31273=CARTESIAN_POINT('Ctrl Pts',(0.418164129143534,1.,1.85417632856234));
#31274=CARTESIAN_POINT('Ctrl Pts',(0.420157287975619,-1.,1.85903281096686));
#31275=CARTESIAN_POINT('Ctrl Pts',(0.420157287975619,1.,1.85903281096686));
#31276=CARTESIAN_POINT('Ctrl Pts',(0.422327307418275,-1.,1.86408083334028));
#31277=CARTESIAN_POINT('Ctrl Pts',(0.422327307418275,1.,1.86408083334028));
#31278=CARTESIAN_POINT('Ctrl Pts',(0.424678177291358,-1.,1.86937803944323));
#31279=CARTESIAN_POINT('Ctrl Pts',(0.424678177291358,1.,1.86937803944323));
#31280=CARTESIAN_POINT('Ctrl Pts',(0.427183828519102,-1.,1.87486989291484));
#31281=CARTESIAN_POINT('Ctrl Pts',(0.427183828519102,1.,1.87486989291484));
#31282=CARTESIAN_POINT('Ctrl Pts',(0.429803062482344,-1.,1.88044229001832));
#31283=CARTESIAN_POINT('Ctrl Pts',(0.429803062482344,1.,1.88044229001832));
#31284=CARTESIAN_POINT('Ctrl Pts',(0.432493038548748,-1.,1.88596913666793));
#31285=CARTESIAN_POINT('Ctrl Pts',(0.432493038548748,1.,1.88596913666793));
#31286=CARTESIAN_POINT('Ctrl Pts',(0.435225660963383,-1.,1.89136993975504));
#31287=CARTESIAN_POINT('Ctrl Pts',(0.435225660963383,1.,1.89136993975504));
#31288=CARTESIAN_POINT('Ctrl Pts',(0.437995003948244,-1.,1.89663648956466));
#31289=CARTESIAN_POINT('Ctrl Pts',(0.437995003948244,1.,1.89663648956466));
#31290=CARTESIAN_POINT('Ctrl Pts',(0.440807833704038,-1.,1.90180124389086));
#31291=CARTESIAN_POINT('Ctrl Pts',(0.440807833704038,1.,1.90180124389086));
#31292=CARTESIAN_POINT('Ctrl Pts',(0.44367755684915,-1.,1.90691756144898));
#31293=CARTESIAN_POINT('Ctrl Pts',(0.44367755684915,1.,1.90691756144898));
#31294=CARTESIAN_POINT('Ctrl Pts',(0.446617343485711,-1.,1.9120369998112));
#31295=CARTESIAN_POINT('Ctrl Pts',(0.446617343485711,1.,1.9120369998112));
#31296=CARTESIAN_POINT('Ctrl Pts',(0.449632260106662,-1.,1.91718342555755));
#31297=CARTESIAN_POINT('Ctrl Pts',(0.449632260106662,1.,1.91718342555755));
#31298=CARTESIAN_POINT('Ctrl Pts',(0.452719478359432,-1.,1.92235380648502));
#31299=CARTESIAN_POINT('Ctrl Pts',(0.452719478359432,1.,1.92235380648502));
#31300=CARTESIAN_POINT('Ctrl Pts',(0.45587200517437,-1.,1.92753067150476));
#31301=CARTESIAN_POINT('Ctrl Pts',(0.45587200517437,1.,1.92753067150476));
#31302=CARTESIAN_POINT('Ctrl Pts',(0.459081234547926,-1.,1.93269066517934));
#31303=CARTESIAN_POINT('Ctrl Pts',(0.459081234547926,1.,1.93269066517934));
#31304=CARTESIAN_POINT('Ctrl Pts',(0.462340031009056,-1.,1.93781486640821));
#31305=CARTESIAN_POINT('Ctrl Pts',(0.462340031009056,1.,1.93781486640821));
#31306=CARTESIAN_POINT('Ctrl Pts',(0.46564546202603,-1.,1.9428979419619));
#31307=CARTESIAN_POINT('Ctrl Pts',(0.46564546202603,1.,1.9428979419619));
#31308=CARTESIAN_POINT('Ctrl Pts',(0.468997482913135,-1.,1.94794381136514));
#31309=CARTESIAN_POINT('Ctrl Pts',(0.468997482913135,1.,1.94794381136514));
#31310=CARTESIAN_POINT('Ctrl Pts',(0.472397672264072,-1.,1.95296148278133));
#31311=CARTESIAN_POINT('Ctrl Pts',(0.472397672264072,1.,1.95296148278133));
#31312=CARTESIAN_POINT('Ctrl Pts',(0.475848034683176,-1.,1.95796111148177));
#31313=CARTESIAN_POINT('Ctrl Pts',(0.475848034683176,1.,1.95796111148177));
#31314=CARTESIAN_POINT('Ctrl Pts',(0.479349583074855,-1.,1.96294933055943));
#31315=CARTESIAN_POINT('Ctrl Pts',(0.479349583074855,1.,1.96294933055943));
#31316=CARTESIAN_POINT('Ctrl Pts',(0.48290166212069,-1.,1.96792703422362));
#31317=CARTESIAN_POINT('Ctrl Pts',(0.48290166212069,1.,1.96792703422362));
#31318=CARTESIAN_POINT('Ctrl Pts',(0.486502692907658,-1.,1.97289186263272));
#31319=CARTESIAN_POINT('Ctrl Pts',(0.486502692907658,1.,1.97289186263272));
#31320=CARTESIAN_POINT('Ctrl Pts',(0.490150627860952,-1.,1.97783973019229));
#31321=CARTESIAN_POINT('Ctrl Pts',(0.490150627860952,1.,1.97783973019229));
#31322=CARTESIAN_POINT('Ctrl Pts',(0.493843476541494,-1.,1.98276658761821));
#31323=CARTESIAN_POINT('Ctrl Pts',(0.493843476541494,1.,1.98276658761821));
#31324=CARTESIAN_POINT('Ctrl Pts',(0.497579909545574,-1.,1.98767044752932));
#31325=CARTESIAN_POINT('Ctrl Pts',(0.497579909545574,1.,1.98767044752932));
#31326=CARTESIAN_POINT('Ctrl Pts',(0.501359287727146,-1.,1.99255149126155));
#31327=CARTESIAN_POINT('Ctrl Pts',(0.501359287727146,1.,1.99255149126155));
#31328=CARTESIAN_POINT('Ctrl Pts',(0.505181361323026,-1.,1.99741107463572));
#31329=CARTESIAN_POINT('Ctrl Pts',(0.505181361323026,1.,1.99741107463572));
#31330=CARTESIAN_POINT('Ctrl Pts',(0.509046069886157,-1.,2.00225107134734));
#31331=CARTESIAN_POINT('Ctrl Pts',(0.509046069886157,1.,2.00225107134734));
#31332=CARTESIAN_POINT('Ctrl Pts',(0.512953306961792,-1.,2.00707309946949));
#31333=CARTESIAN_POINT('Ctrl Pts',(0.512953306961792,1.,2.00707309946949));
#31334=CARTESIAN_POINT('Ctrl Pts',(0.516902681728687,-1.,2.01187773939242));
#31335=CARTESIAN_POINT('Ctrl Pts',(0.516902681728687,1.,2.01187773939242));
#31336=CARTESIAN_POINT('Ctrl Pts',(0.52089359039937,-1.,2.01666477917286));
#31337=CARTESIAN_POINT('Ctrl Pts',(0.52089359039937,1.,2.01666477917286));
#31338=CARTESIAN_POINT('Ctrl Pts',(0.524925318333476,-1.,2.02143356304698));
#31339=CARTESIAN_POINT('Ctrl Pts',(0.524925318333476,1.,2.02143356304698));
#31340=CARTESIAN_POINT('Ctrl Pts',(0.528997127241914,-1.,2.0261832908329));
#31341=CARTESIAN_POINT('Ctrl Pts',(0.528997127241914,1.,2.0261832908329));
#31342=CARTESIAN_POINT('Ctrl Pts',(0.533108355132976,-1.,2.03091336214426));
#31343=CARTESIAN_POINT('Ctrl Pts',(0.533108355132976,1.,2.03091336214426));
#31344=CARTESIAN_POINT('Ctrl Pts',(0.537258489833262,-1.,2.03562362954037));
#31345=CARTESIAN_POINT('Ctrl Pts',(0.537258489833262,1.,2.03562362954037));
#31346=CARTESIAN_POINT('Ctrl Pts',(0.541447120615659,-1.,2.04031422690527));
#31347=CARTESIAN_POINT('Ctrl Pts',(0.541447120615659,1.,2.04031422690527));
#31348=CARTESIAN_POINT('Ctrl Pts',(0.54567390381743,-1.,2.04498544714588));
#31349=CARTESIAN_POINT('Ctrl Pts',(0.54567390381743,1.,2.04498544714588));
#31350=CARTESIAN_POINT('Ctrl Pts',(0.549938525150295,-1.,2.04963761077958));
#31351=CARTESIAN_POINT('Ctrl Pts',(0.549938525150295,1.,2.04963761077958));
#31352=CARTESIAN_POINT('Ctrl Pts',(0.554240657463906,-1.,2.05427091604413));
#31353=CARTESIAN_POINT('Ctrl Pts',(0.554240657463906,1.,2.05427091604413));
#31354=CARTESIAN_POINT('Ctrl Pts',(0.558579940185151,-1.,2.05888537756462));
#31355=CARTESIAN_POINT('Ctrl Pts',(0.558579940185151,1.,2.05888537756462));
#31356=CARTESIAN_POINT('Ctrl Pts',(0.562955993082261,-1.,2.06348090160589));
#31357=CARTESIAN_POINT('Ctrl Pts',(0.562955993082261,1.,2.06348090160589));
#31358=CARTESIAN_POINT('Ctrl Pts',(0.567368421181087,-1.,2.06805732997334));
#31359=CARTESIAN_POINT('Ctrl Pts',(0.567368421181087,1.,2.06805732997334));
#31360=CARTESIAN_POINT('Ctrl Pts',(0.571816823242602,-1.,2.07261449292824));
#31361=CARTESIAN_POINT('Ctrl Pts',(0.571816823242602,1.,2.07261449292824));
#31362=CARTESIAN_POINT('Ctrl Pts',(0.576300797416844,-1.,2.07715226767559));
#31363=CARTESIAN_POINT('Ctrl Pts',(0.576300797416844,1.,2.07715226767559));
#31364=CARTESIAN_POINT('Ctrl Pts',(0.580819952108063,-1.,2.08167059018418));
#31365=CARTESIAN_POINT('Ctrl Pts',(0.580819952108063,1.,2.08167059018418));
#31366=CARTESIAN_POINT('Ctrl Pts',(0.585373918991617,-1.,2.08616943727951));
#31367=CARTESIAN_POINT('Ctrl Pts',(0.585373918991617,1.,2.08616943727951));
#31368=CARTESIAN_POINT('Ctrl Pts',(0.589962365403406,-1.,2.09064881812129));
#31369=CARTESIAN_POINT('Ctrl Pts',(0.589962365403406,1.,2.09064881812129));
#31370=CARTESIAN_POINT('Ctrl Pts',(0.594585006052162,-1.,2.0951087622027));
#31371=CARTESIAN_POINT('Ctrl Pts',(0.594585006052162,1.,2.0951087622027));
#31372=CARTESIAN_POINT('Ctrl Pts',(0.599241616420533,-1.,2.0995493086477));
#31373=CARTESIAN_POINT('Ctrl Pts',(0.599241616420533,1.,2.0995493086477));
#31374=CARTESIAN_POINT('Ctrl Pts',(0.60393203073603,-1.,2.10397049886949));
#31375=CARTESIAN_POINT('Ctrl Pts',(0.60393203073603,1.,2.10397049886949));
#31376=CARTESIAN_POINT('Ctrl Pts',(0.607711315454876,-1.,2.1074919961518));
#31377=CARTESIAN_POINT('Ctrl Pts',(0.607711315454876,1.,2.1074919961518));
#31378=CARTESIAN_POINT('Ctrl Pts',(0.610560911689898,-1.,2.11012443807238));
#31379=CARTESIAN_POINT('Ctrl Pts',(0.610560911689898,1.,2.11012443807238));
#31380=CARTESIAN_POINT('Ctrl Pts',(0.6124673655618,-1.,2.11187554259986));
#31381=CARTESIAN_POINT('Ctrl Pts',(0.6124673655618,1.,2.11187554259986));
#31382=CARTESIAN_POINT('Ctrl Pts',(0.61342227326009,-1.,2.11275013067528));
#31383=CARTESIAN_POINT('Ctrl Pts',(0.61342227326009,1.,2.11275013067528));
#31384=CARTESIAN_POINT('',(0.383122945602004,1.,1.7075470150345));
#31385=CARTESIAN_POINT('Ctrl Pts',(0.383122945602004,1.,1.7075470150345));
#31386=CARTESIAN_POINT('Ctrl Pts',(0.384119047315541,1.,1.71231062891958));
#31387=CARTESIAN_POINT('Ctrl Pts',(0.38607079032701,1.,1.72162022246158));
#31388=CARTESIAN_POINT('Ctrl Pts',(0.388877023509191,1.,1.7349317097561));
#31389=CARTESIAN_POINT('Ctrl Pts',(0.392375812294307,1.,1.75137405313962));
#31390=CARTESIAN_POINT('Ctrl Pts',(0.39634619612042,1.,1.7697556004756));
#31391=CARTESIAN_POINT('Ctrl Pts',(0.39991940378308,1.,1.78598826347533));
#31392=CARTESIAN_POINT('Ctrl Pts',(0.403107976170441,1.,1.80012077176221));
#31393=CARTESIAN_POINT('Ctrl Pts',(0.405933518411838,1.,1.81223801813988));
#31394=CARTESIAN_POINT('Ctrl Pts',(0.408428948108533,1.,1.8224702267854));
#31395=CARTESIAN_POINT('Ctrl Pts',(0.410641256301674,1.,1.83100408895216));
#31396=CARTESIAN_POINT('Ctrl Pts',(0.412633125322161,1.,1.83808953475839));
#31397=CARTESIAN_POINT('Ctrl Pts',(0.41448743825434,1.,1.8440575707371));
#31398=CARTESIAN_POINT('Ctrl Pts',(0.416300022038864,1.,1.84929312929882));
#31399=CARTESIAN_POINT('Ctrl Pts',(0.418164129143534,1.,1.85417632856234));
#31400=CARTESIAN_POINT('Ctrl Pts',(0.420157287975619,1.,1.85903281096686));
#31401=CARTESIAN_POINT('Ctrl Pts',(0.422327307418275,1.,1.86408083334028));
#31402=CARTESIAN_POINT('Ctrl Pts',(0.424678177291358,1.,1.86937803944323));
#31403=CARTESIAN_POINT('Ctrl Pts',(0.427183828519102,1.,1.87486989291484));
#31404=CARTESIAN_POINT('Ctrl Pts',(0.429803062482344,1.,1.88044229001832));
#31405=CARTESIAN_POINT('Ctrl Pts',(0.432493038548748,1.,1.88596913666793));
#31406=CARTESIAN_POINT('Ctrl Pts',(0.435225660963383,1.,1.89136993975504));
#31407=CARTESIAN_POINT('Ctrl Pts',(0.437995003948244,1.,1.89663648956466));
#31408=CARTESIAN_POINT('Ctrl Pts',(0.440807833704038,1.,1.90180124389086));
#31409=CARTESIAN_POINT('Ctrl Pts',(0.44367755684915,1.,1.90691756144898));
#31410=CARTESIAN_POINT('Ctrl Pts',(0.446617343485711,1.,1.9120369998112));
#31411=CARTESIAN_POINT('Ctrl Pts',(0.449632260106662,1.,1.91718342555755));
#31412=CARTESIAN_POINT('Ctrl Pts',(0.452719478359432,1.,1.92235380648502));
#31413=CARTESIAN_POINT('Ctrl Pts',(0.45587200517437,1.,1.92753067150476));
#31414=CARTESIAN_POINT('Ctrl Pts',(0.459081234547926,1.,1.93269066517934));
#31415=CARTESIAN_POINT('Ctrl Pts',(0.462340031009056,1.,1.93781486640821));
#31416=CARTESIAN_POINT('Ctrl Pts',(0.46564546202603,1.,1.9428979419619));
#31417=CARTESIAN_POINT('Ctrl Pts',(0.468997482913135,1.,1.94794381136514));
#31418=CARTESIAN_POINT('Ctrl Pts',(0.472397672264072,1.,1.95296148278133));
#31419=CARTESIAN_POINT('Ctrl Pts',(0.475848034683176,1.,1.95796111148177));
#31420=CARTESIAN_POINT('Ctrl Pts',(0.479349583074855,1.,1.96294933055943));
#31421=CARTESIAN_POINT('Ctrl Pts',(0.48290166212069,1.,1.96792703422362));
#31422=CARTESIAN_POINT('Ctrl Pts',(0.486502692907658,1.,1.97289186263272));
#31423=CARTESIAN_POINT('Ctrl Pts',(0.490150627860952,1.,1.97783973019229));
#31424=CARTESIAN_POINT('Ctrl Pts',(0.493843476541494,1.,1.98276658761821));
#31425=CARTESIAN_POINT('Ctrl Pts',(0.497579909545574,1.,1.98767044752932));
#31426=CARTESIAN_POINT('Ctrl Pts',(0.501359287727146,1.,1.99255149126155));
#31427=CARTESIAN_POINT('Ctrl Pts',(0.505181361323026,1.,1.99741107463572));
#31428=CARTESIAN_POINT('Ctrl Pts',(0.509046069886157,1.,2.00225107134734));
#31429=CARTESIAN_POINT('Ctrl Pts',(0.512953306961792,1.,2.00707309946949));
#31430=CARTESIAN_POINT('Ctrl Pts',(0.516902681728687,1.,2.01187773939242));
#31431=CARTESIAN_POINT('Ctrl Pts',(0.52089359039937,1.,2.01666477917286));
#31432=CARTESIAN_POINT('Ctrl Pts',(0.524925318333476,1.,2.02143356304698));
#31433=CARTESIAN_POINT('Ctrl Pts',(0.528997127241914,1.,2.0261832908329));
#31434=CARTESIAN_POINT('Ctrl Pts',(0.533108355132976,1.,2.03091336214426));
#31435=CARTESIAN_POINT('Ctrl Pts',(0.537258489833262,1.,2.03562362954037));
#31436=CARTESIAN_POINT('Ctrl Pts',(0.541447120615659,1.,2.04031422690527));
#31437=CARTESIAN_POINT('Ctrl Pts',(0.54567390381743,1.,2.04498544714588));
#31438=CARTESIAN_POINT('Ctrl Pts',(0.549938525150295,1.,2.04963761077958));
#31439=CARTESIAN_POINT('Ctrl Pts',(0.554240657463906,1.,2.05427091604413));
#31440=CARTESIAN_POINT('Ctrl Pts',(0.558579940185151,1.,2.05888537756462));
#31441=CARTESIAN_POINT('Ctrl Pts',(0.562955993082261,1.,2.06348090160589));
#31442=CARTESIAN_POINT('Ctrl Pts',(0.567368421181087,1.,2.06805732997334));
#31443=CARTESIAN_POINT('Ctrl Pts',(0.571816823242602,1.,2.07261449292824));
#31444=CARTESIAN_POINT('Ctrl Pts',(0.576300797416844,1.,2.07715226767559));
#31445=CARTESIAN_POINT('Ctrl Pts',(0.580819952108063,1.,2.08167059018418));
#31446=CARTESIAN_POINT('Ctrl Pts',(0.585373918991617,1.,2.08616943727951));
#31447=CARTESIAN_POINT('Ctrl Pts',(0.589962365403406,1.,2.09064881812129));
#31448=CARTESIAN_POINT('Ctrl Pts',(0.594585006052162,1.,2.0951087622027));
#31449=CARTESIAN_POINT('Ctrl Pts',(0.599241616420533,1.,2.0995493086477));
#31450=CARTESIAN_POINT('Ctrl Pts',(0.60393203073603,1.,2.10397049886949));
#31451=CARTESIAN_POINT('Ctrl Pts',(0.607711315454876,1.,2.1074919961518));
#31452=CARTESIAN_POINT('Ctrl Pts',(0.610560911689898,1.,2.11012443807238));
#31453=CARTESIAN_POINT('Ctrl Pts',(0.6124673655618,1.,2.11187554259986));
#31454=CARTESIAN_POINT('Ctrl Pts',(0.61342227326009,1.,2.11275013067528));
#31455=CARTESIAN_POINT('',(0.383122945602003,0.,1.7075470150345));
#31456=CARTESIAN_POINT('Origin',(0.,0.,0.));
#31457=CARTESIAN_POINT('',(0.163289472382896,1.,1.74236521665491));
#31458=CARTESIAN_POINT('Origin',(0.,1.,0.));
#31459=CARTESIAN_POINT('',(0.163289472382896,0.,1.74236521665491));
#31460=CARTESIAN_POINT('Ctrl Pts',(0.0694764450219578,-1.,2.19890268624765));
#31461=CARTESIAN_POINT('Ctrl Pts',(0.0694764450219578,1.,2.19890268624765));
#31462=CARTESIAN_POINT('Ctrl Pts',(0.0701143536325487,-1.,2.19777582085423));
#31463=CARTESIAN_POINT('Ctrl Pts',(0.0701143536325487,1.,2.19777582085423));
#31464=CARTESIAN_POINT('Ctrl Pts',(0.0713863779526151,-1.,2.19552129484002));
#31465=CARTESIAN_POINT('Ctrl Pts',(0.0713863779526151,1.,2.19552129484002));
#31466=CARTESIAN_POINT('Ctrl Pts',(0.0732830357306722,-1.,2.19213712013662));
#31467=CARTESIAN_POINT('Ctrl Pts',(0.0732830357306722,1.,2.19213712013662));
#31468=CARTESIAN_POINT('Ctrl Pts',(0.0757891465836145,-1.,2.1876201139953));
#31469=CARTESIAN_POINT('Ctrl Pts',(0.0757891465836145,1.,2.1876201139953));
#31470=CARTESIAN_POINT('Ctrl Pts',(0.078883772768524,-1.,2.18196589448887));
#31471=CARTESIAN_POINT('Ctrl Pts',(0.078883772768524,1.,2.18196589448887));
#31472=CARTESIAN_POINT('Ctrl Pts',(0.0819402680872763,-1.,2.176303712113));
#31473=CARTESIAN_POINT('Ctrl Pts',(0.0819402680872763,1.,2.176303712113));
#31474=CARTESIAN_POINT('Ctrl Pts',(0.084958462083537,-1.,2.17063357870952));
#31475=CARTESIAN_POINT('Ctrl Pts',(0.084958462083537,1.,2.17063357870952));
#31476=CARTESIAN_POINT('Ctrl Pts',(0.087938129138692,-1.,2.16495552645014));
#31477=CARTESIAN_POINT('Ctrl Pts',(0.087938129138692,1.,2.16495552645014));
#31478=CARTESIAN_POINT('Ctrl Pts',(0.0908789888107263,-1.,2.15926961544516));
#31479=CARTESIAN_POINT('Ctrl Pts',(0.0908789888107263,1.,2.15926961544516));
#31480=CARTESIAN_POINT('Ctrl Pts',(0.0937807218867641,-1.,2.1535759397817));
#31481=CARTESIAN_POINT('Ctrl Pts',(0.0937807218867641,1.,2.1535759397817));
#31482=CARTESIAN_POINT('Ctrl Pts',(0.0966429852305456,-1.,2.14787463531795));
#31483=CARTESIAN_POINT('Ctrl Pts',(0.0966429852305456,1.,2.14787463531795));
#31484=CARTESIAN_POINT('Ctrl Pts',(0.0994654261990913,-1.,2.14216588396025));
#31485=CARTESIAN_POINT('Ctrl Pts',(0.0994654261990913,1.,2.14216588396025));
#31486=CARTESIAN_POINT('Ctrl Pts',(0.1022477005561,-1.,2.13644992667165));
#31487=CARTESIAN_POINT('Ctrl Pts',(0.1022477005561,1.,2.13644992667165));
#31488=CARTESIAN_POINT('Ctrl Pts',(0.104989479152739,-1.,2.13072704887293));
#31489=CARTESIAN_POINT('Ctrl Pts',(0.104989479152739,1.,2.13072704887293));
#31490=CARTESIAN_POINT('Ctrl Pts',(0.10769043523109,-1.,2.12499752307));
#31491=CARTESIAN_POINT('Ctrl Pts',(0.10769043523109,1.,2.12499752307));
#31492=CARTESIAN_POINT('Ctrl Pts',(0.110350236135025,-1.,2.11926155590865));
#31493=CARTESIAN_POINT('Ctrl Pts',(0.110350236135025,1.,2.11926155590865));
#31494=CARTESIAN_POINT('Ctrl Pts',(0.112968534419737,-1.,2.11351924490306));
#31495=CARTESIAN_POINT('Ctrl Pts',(0.112968534419737,1.,2.11351924490306));
#31496=CARTESIAN_POINT('Ctrl Pts',(0.115544957687926,-1.,2.10777050261309));
#31497=CARTESIAN_POINT('Ctrl Pts',(0.115544957687926,1.,2.10777050261309));
#31498=CARTESIAN_POINT('Ctrl Pts',(0.118079107988355,-1.,2.102015121329));
#31499=CARTESIAN_POINT('Ctrl Pts',(0.118079107988355,1.,2.102015121329));
#31500=CARTESIAN_POINT('Ctrl Pts',(0.120570567965122,-1.,2.0962529286773));
#31501=CARTESIAN_POINT('Ctrl Pts',(0.120570567965122,1.,2.0962529286773));
#31502=CARTESIAN_POINT('Ctrl Pts',(0.123018905621083,-1.,2.09048392424825));
#31503=CARTESIAN_POINT('Ctrl Pts',(0.123018905621083,1.,2.09048392424825));
#31504=CARTESIAN_POINT('Ctrl Pts',(0.125423679412061,-1.,2.08470840653643));
#31505=CARTESIAN_POINT('Ctrl Pts',(0.125423679412061,1.,2.08470840653643));
#31506=CARTESIAN_POINT('Ctrl Pts',(0.12778444527612,-1.,2.07892715110987));
#31507=CARTESIAN_POINT('Ctrl Pts',(0.12778444527612,1.,2.07892715110987));
#31508=CARTESIAN_POINT('Ctrl Pts',(0.130100748328403,-1.,2.07314114713063));
#31509=CARTESIAN_POINT('Ctrl Pts',(0.130100748328403,1.,2.07314114713063));
#31510=CARTESIAN_POINT('Ctrl Pts',(0.13237211154771,-1.,2.06735123910326));
#31511=CARTESIAN_POINT('Ctrl Pts',(0.13237211154771,1.,2.06735123910326));
#31512=CARTESIAN_POINT('Ctrl Pts',(0.134598026192106,-1.,2.06155781517842));
#31513=CARTESIAN_POINT('Ctrl Pts',(0.134598026192106,1.,2.06155781517842));
#31514=CARTESIAN_POINT('Ctrl Pts',(0.136777941218043,-1.,2.05576044414264));
#31515=CARTESIAN_POINT('Ctrl Pts',(0.136777941218043,1.,2.05576044414264));
#31516=CARTESIAN_POINT('Ctrl Pts',(0.138911255368966,-1.,2.04995762001328));
#31517=CARTESIAN_POINT('Ctrl Pts',(0.138911255368966,1.,2.04995762001328));
#31518=CARTESIAN_POINT('Ctrl Pts',(0.140997332152546,-1.,2.04414757947916));
#31519=CARTESIAN_POINT('Ctrl Pts',(0.140997332152546,1.,2.04414757947916));
#31520=CARTESIAN_POINT('Ctrl Pts',(0.143035515058208,-1.,2.03832911025912));
#31521=CARTESIAN_POINT('Ctrl Pts',(0.143035515058208,1.,2.03832911025912));
#31522=CARTESIAN_POINT('Ctrl Pts',(0.145025140186057,-1.,2.03250223739942));
#31523=CARTESIAN_POINT('Ctrl Pts',(0.145025140186057,1.,2.03250223739942));
#31524=CARTESIAN_POINT('Ctrl Pts',(0.146965557332583,-1.,2.02666926182017));
#31525=CARTESIAN_POINT('Ctrl Pts',(0.146965557332583,1.,2.02666926182017));
#31526=CARTESIAN_POINT('Ctrl Pts',(0.148856124775337,-1.,2.02083464969894));
#31527=CARTESIAN_POINT('Ctrl Pts',(0.148856124775337,1.,2.02083464969894));
#31528=CARTESIAN_POINT('Ctrl Pts',(0.150696157673078,-1.,2.01500291940238));
#31529=CARTESIAN_POINT('Ctrl Pts',(0.150696157673078,1.,2.01500291940238));
#31530=CARTESIAN_POINT('Ctrl Pts',(0.152484883621449,-1.,2.00917680318424));
#31531=CARTESIAN_POINT('Ctrl Pts',(0.152484883621449,1.,2.00917680318424));
#31532=CARTESIAN_POINT('Ctrl Pts',(0.154221403049722,-1.,2.00335565310543));
#31533=CARTESIAN_POINT('Ctrl Pts',(0.154221403049722,1.,2.00335565310543));
#31534=CARTESIAN_POINT('Ctrl Pts',(0.155904629548783,-1.,1.99753284771497));
#31535=CARTESIAN_POINT('Ctrl Pts',(0.155904629548783,1.,1.99753284771497));
#31536=CARTESIAN_POINT('Ctrl Pts',(0.157533331459227,-1.,1.99169810931908));
#31537=CARTESIAN_POINT('Ctrl Pts',(0.157533331459227,1.,1.99169810931908));
#31538=CARTESIAN_POINT('Ctrl Pts',(0.159106226437299,-1.,1.98584238283292));
#31539=CARTESIAN_POINT('Ctrl Pts',(0.159106226437299,1.,1.98584238283292));
#31540=CARTESIAN_POINT('Ctrl Pts',(0.160622060784611,-1.,1.97996195437559));
#31541=CARTESIAN_POINT('Ctrl Pts',(0.160622060784611,1.,1.97996195437559));
#31542=CARTESIAN_POINT('Ctrl Pts',(0.162079693556288,-1.,1.97406280235188));
#31543=CARTESIAN_POINT('Ctrl Pts',(0.162079693556288,1.,1.97406280235188));
#31544=CARTESIAN_POINT('Ctrl Pts',(0.163478185457734,-1.,1.96816512677967));
#31545=CARTESIAN_POINT('Ctrl Pts',(0.163478185457734,1.,1.96816512677967));
#31546=CARTESIAN_POINT('Ctrl Pts',(0.164816568920269,-1.,1.96229379940136));
#31547=CARTESIAN_POINT('Ctrl Pts',(0.164816568920269,1.,1.96229379940136));
#31548=CARTESIAN_POINT('Ctrl Pts',(0.166093592002812,-1.,1.9564675971873));
#31549=CARTESIAN_POINT('Ctrl Pts',(0.166093592002812,1.,1.9564675971873));
#31550=CARTESIAN_POINT('Ctrl Pts',(0.167307501784475,-1.,1.95069027794294));
#31551=CARTESIAN_POINT('Ctrl Pts',(0.167307501784475,1.,1.95069027794294));
#31552=CARTESIAN_POINT('Ctrl Pts',(0.168455741607556,-1.,1.94493757756931));
#31553=CARTESIAN_POINT('Ctrl Pts',(0.168455741607556,1.,1.94493757756931));
#31554=CARTESIAN_POINT('Ctrl Pts',(0.16953490481749,-1.,1.93915639211581));
#31555=CARTESIAN_POINT('Ctrl Pts',(0.16953490481749,1.,1.93915639211581));
#31556=CARTESIAN_POINT('Ctrl Pts',(0.170541253116201,-1.,1.93329183155539));
#31557=CARTESIAN_POINT('Ctrl Pts',(0.170541253116201,1.,1.93329183155539));
#31558=CARTESIAN_POINT('Ctrl Pts',(0.171471191532988,-1.,1.92731093582036));
#31559=CARTESIAN_POINT('Ctrl Pts',(0.171471191532988,1.,1.92731093582036));
#31560=CARTESIAN_POINT('Ctrl Pts',(0.172321621259513,-1.,1.9212233439798));
#31561=CARTESIAN_POINT('Ctrl Pts',(0.172321621259513,1.,1.9212233439798));
#31562=CARTESIAN_POINT('Ctrl Pts',(0.173090695383496,-1.,1.91511429159527));
#31563=CARTESIAN_POINT('Ctrl Pts',(0.173090695383496,1.,1.91511429159527));
#31564=CARTESIAN_POINT('Ctrl Pts',(0.173776635257816,-1.,1.90911693975267));
#31565=CARTESIAN_POINT('Ctrl Pts',(0.173776635257816,1.,1.90911693975267));
#31566=CARTESIAN_POINT('Ctrl Pts',(0.174375518661085,-1.,1.90335253862834));
#31567=CARTESIAN_POINT('Ctrl Pts',(0.174375518661085,1.,1.90335253862834));
#31568=CARTESIAN_POINT('Ctrl Pts',(0.174879405091263,-1.,1.89788101117132));
#31569=CARTESIAN_POINT('Ctrl Pts',(0.174879405091263,1.,1.89788101117132));
#31570=CARTESIAN_POINT('Ctrl Pts',(0.175274276190844,-1.,1.892646301985));
#31571=CARTESIAN_POINT('Ctrl Pts',(0.175274276190844,1.,1.892646301985));
#31572=CARTESIAN_POINT('Ctrl Pts',(0.175538155840648,-1.,1.88742606273259));
#31573=CARTESIAN_POINT('Ctrl Pts',(0.175538155840648,1.,1.88742606273259));
#31574=CARTESIAN_POINT('Ctrl Pts',(0.175644148889698,-1.,1.88188663145367));
#31575=CARTESIAN_POINT('Ctrl Pts',(0.175644148889698,1.,1.88188663145367));
#31576=CARTESIAN_POINT('Ctrl Pts',(0.175563480746485,-1.,1.87563767773588));
#31577=CARTESIAN_POINT('Ctrl Pts',(0.175563480746485,1.,1.87563767773588));
#31578=CARTESIAN_POINT('Ctrl Pts',(0.175268337590757,-1.,1.86828349694799));
#31579=CARTESIAN_POINT('Ctrl Pts',(0.175268337590757,1.,1.86828349694799));
#31580=CARTESIAN_POINT('Ctrl Pts',(0.17473525927603,-1.,1.85948367088837));
#31581=CARTESIAN_POINT('Ctrl Pts',(0.17473525927603,1.,1.85948367088837));
#31582=CARTESIAN_POINT('Ctrl Pts',(0.173946627587731,-1.,1.8489811319852));
#31583=CARTESIAN_POINT('Ctrl Pts',(0.173946627587731,1.,1.8489811319852));
#31584=CARTESIAN_POINT('Ctrl Pts',(0.1728894428919,-1.,1.83658380527692));
#31585=CARTESIAN_POINT('Ctrl Pts',(0.1728894428919,1.,1.83658380527692));
#31586=CARTESIAN_POINT('Ctrl Pts',(0.171554770204119,-1.,1.82215766811545));
#31587=CARTESIAN_POINT('Ctrl Pts',(0.171554770204119,1.,1.82215766811545));
#31588=CARTESIAN_POINT('Ctrl Pts',(0.169936923904608,-1.,1.80561530629706));
#31589=CARTESIAN_POINT('Ctrl Pts',(0.169936923904608,1.,1.80561530629706));
#31590=CARTESIAN_POINT('Ctrl Pts',(0.168032772805197,-1.,1.7869064998507));
#31591=CARTESIAN_POINT('Ctrl Pts',(0.168032772805197,1.,1.7869064998507));
#31592=CARTESIAN_POINT('Ctrl Pts',(0.1662793551464,-1.,1.77018771684844));
#31593=CARTESIAN_POINT('Ctrl Pts',(0.1662793551464,1.,1.77018771684844));
#31594=CARTESIAN_POINT('Ctrl Pts',(0.164834765707158,-1.,1.75666056638427));
#31595=CARTESIAN_POINT('Ctrl Pts',(0.164834765707158,1.,1.75666056638427));
#31596=CARTESIAN_POINT('Ctrl Pts',(0.163814161002002,-1.,1.7472034950333));
#31597=CARTESIAN_POINT('Ctrl Pts',(0.163814161002002,1.,1.7472034950333));
#31598=CARTESIAN_POINT('Ctrl Pts',(0.163289472382896,-1.,1.74236521665491));
#31599=CARTESIAN_POINT('Ctrl Pts',(0.163289472382896,1.,1.74236521665491));
#31600=CARTESIAN_POINT('',(0.0694764450219578,1.,2.19890268624765));
#31601=CARTESIAN_POINT('Ctrl Pts',(0.0694764450219578,1.,2.19890268624765));
#31602=CARTESIAN_POINT('Ctrl Pts',(0.0701143536325487,1.,2.19777582085423));
#31603=CARTESIAN_POINT('Ctrl Pts',(0.0713863779526151,1.,2.19552129484002));
#31604=CARTESIAN_POINT('Ctrl Pts',(0.0732830357306722,1.,2.19213712013662));
#31605=CARTESIAN_POINT('Ctrl Pts',(0.0757891465836145,1.,2.1876201139953));
#31606=CARTESIAN_POINT('Ctrl Pts',(0.078883772768524,1.,2.18196589448887));
#31607=CARTESIAN_POINT('Ctrl Pts',(0.0819402680872763,1.,2.176303712113));
#31608=CARTESIAN_POINT('Ctrl Pts',(0.084958462083537,1.,2.17063357870952));
#31609=CARTESIAN_POINT('Ctrl Pts',(0.087938129138692,1.,2.16495552645014));
#31610=CARTESIAN_POINT('Ctrl Pts',(0.0908789888107263,1.,2.15926961544516));
#31611=CARTESIAN_POINT('Ctrl Pts',(0.0937807218867641,1.,2.1535759397817));
#31612=CARTESIAN_POINT('Ctrl Pts',(0.0966429852305456,1.,2.14787463531795));
#31613=CARTESIAN_POINT('Ctrl Pts',(0.0994654261990913,1.,2.14216588396025));
#31614=CARTESIAN_POINT('Ctrl Pts',(0.1022477005561,1.,2.13644992667165));
#31615=CARTESIAN_POINT('Ctrl Pts',(0.104989479152739,1.,2.13072704887293));
#31616=CARTESIAN_POINT('Ctrl Pts',(0.10769043523109,1.,2.12499752307));
#31617=CARTESIAN_POINT('Ctrl Pts',(0.110350236135025,1.,2.11926155590865));
#31618=CARTESIAN_POINT('Ctrl Pts',(0.112968534419737,1.,2.11351924490306));
#31619=CARTESIAN_POINT('Ctrl Pts',(0.115544957687926,1.,2.10777050261309));
#31620=CARTESIAN_POINT('Ctrl Pts',(0.118079107988355,1.,2.102015121329));
#31621=CARTESIAN_POINT('Ctrl Pts',(0.120570567965122,1.,2.0962529286773));
#31622=CARTESIAN_POINT('Ctrl Pts',(0.123018905621083,1.,2.09048392424825));
#31623=CARTESIAN_POINT('Ctrl Pts',(0.125423679412061,1.,2.08470840653643));
#31624=CARTESIAN_POINT('Ctrl Pts',(0.12778444527612,1.,2.07892715110987));
#31625=CARTESIAN_POINT('Ctrl Pts',(0.130100748328403,1.,2.07314114713063));
#31626=CARTESIAN_POINT('Ctrl Pts',(0.13237211154771,1.,2.06735123910326));
#31627=CARTESIAN_POINT('Ctrl Pts',(0.134598026192106,1.,2.06155781517842));
#31628=CARTESIAN_POINT('Ctrl Pts',(0.136777941218043,1.,2.05576044414264));
#31629=CARTESIAN_POINT('Ctrl Pts',(0.138911255368966,1.,2.04995762001328));
#31630=CARTESIAN_POINT('Ctrl Pts',(0.140997332152546,1.,2.04414757947916));
#31631=CARTESIAN_POINT('Ctrl Pts',(0.143035515058208,1.,2.03832911025912));
#31632=CARTESIAN_POINT('Ctrl Pts',(0.145025140186057,1.,2.03250223739942));
#31633=CARTESIAN_POINT('Ctrl Pts',(0.146965557332583,1.,2.02666926182017));
#31634=CARTESIAN_POINT('Ctrl Pts',(0.148856124775337,1.,2.02083464969894));
#31635=CARTESIAN_POINT('Ctrl Pts',(0.150696157673078,1.,2.01500291940238));
#31636=CARTESIAN_POINT('Ctrl Pts',(0.152484883621449,1.,2.00917680318424));
#31637=CARTESIAN_POINT('Ctrl Pts',(0.154221403049722,1.,2.00335565310543));
#31638=CARTESIAN_POINT('Ctrl Pts',(0.155904629548783,1.,1.99753284771497));
#31639=CARTESIAN_POINT('Ctrl Pts',(0.157533331459227,1.,1.99169810931908));
#31640=CARTESIAN_POINT('Ctrl Pts',(0.159106226437299,1.,1.98584238283292));
#31641=CARTESIAN_POINT('Ctrl Pts',(0.160622060784611,1.,1.97996195437559));
#31642=CARTESIAN_POINT('Ctrl Pts',(0.162079693556288,1.,1.97406280235188));
#31643=CARTESIAN_POINT('Ctrl Pts',(0.163478185457734,1.,1.96816512677967));
#31644=CARTESIAN_POINT('Ctrl Pts',(0.164816568920269,1.,1.96229379940136));
#31645=CARTESIAN_POINT('Ctrl Pts',(0.166093592002812,1.,1.9564675971873));
#31646=CARTESIAN_POINT('Ctrl Pts',(0.167307501784475,1.,1.95069027794294));
#31647=CARTESIAN_POINT('Ctrl Pts',(0.168455741607556,1.,1.94493757756931));
#31648=CARTESIAN_POINT('Ctrl Pts',(0.16953490481749,1.,1.93915639211581));
#31649=CARTESIAN_POINT('Ctrl Pts',(0.170541253116201,1.,1.93329183155539));
#31650=CARTESIAN_POINT('Ctrl Pts',(0.171471191532988,1.,1.92731093582036));
#31651=CARTESIAN_POINT('Ctrl Pts',(0.172321621259513,1.,1.9212233439798));
#31652=CARTESIAN_POINT('Ctrl Pts',(0.173090695383496,1.,1.91511429159527));
#31653=CARTESIAN_POINT('Ctrl Pts',(0.173776635257816,1.,1.90911693975267));
#31654=CARTESIAN_POINT('Ctrl Pts',(0.174375518661085,1.,1.90335253862834));
#31655=CARTESIAN_POINT('Ctrl Pts',(0.174879405091263,1.,1.89788101117132));
#31656=CARTESIAN_POINT('Ctrl Pts',(0.175274276190844,1.,1.892646301985));
#31657=CARTESIAN_POINT('Ctrl Pts',(0.175538155840648,1.,1.88742606273259));
#31658=CARTESIAN_POINT('Ctrl Pts',(0.175644148889698,1.,1.88188663145367));
#31659=CARTESIAN_POINT('Ctrl Pts',(0.175563480746485,1.,1.87563767773588));
#31660=CARTESIAN_POINT('Ctrl Pts',(0.175268337590757,1.,1.86828349694799));
#31661=CARTESIAN_POINT('Ctrl Pts',(0.17473525927603,1.,1.85948367088837));
#31662=CARTESIAN_POINT('Ctrl Pts',(0.173946627587731,1.,1.8489811319852));
#31663=CARTESIAN_POINT('Ctrl Pts',(0.1728894428919,1.,1.83658380527692));
#31664=CARTESIAN_POINT('Ctrl Pts',(0.171554770204119,1.,1.82215766811545));
#31665=CARTESIAN_POINT('Ctrl Pts',(0.169936923904608,1.,1.80561530629706));
#31666=CARTESIAN_POINT('Ctrl Pts',(0.168032772805197,1.,1.7869064998507));
#31667=CARTESIAN_POINT('Ctrl Pts',(0.1662793551464,1.,1.77018771684844));
#31668=CARTESIAN_POINT('Ctrl Pts',(0.164834765707158,1.,1.75666056638427));
#31669=CARTESIAN_POINT('Ctrl Pts',(0.163814161002002,1.,1.7472034950333));
#31670=CARTESIAN_POINT('Ctrl Pts',(0.163289472382896,1.,1.74236521665491));
#31671=CARTESIAN_POINT('',(0.0694764450219578,0.,2.19890268624765));
#31672=CARTESIAN_POINT('Origin',(-0.0694764450219586,0.,2.19890268624765));
#31673=CARTESIAN_POINT('',(-0.0694764450219586,1.,2.19890268624765));
#31674=CARTESIAN_POINT('',(0.0694764450219578,1.,2.19890268624765));
#31675=CARTESIAN_POINT('',(-0.0694764450219586,0.,2.19890268624765));
#31676=CARTESIAN_POINT('Ctrl Pts',(-0.163289472382896,-1.,1.74236521665491));
#31677=CARTESIAN_POINT('Ctrl Pts',(-0.163289472382896,1.,1.74236521665491));
#31678=CARTESIAN_POINT('Ctrl Pts',(-0.163814161002474,-1.,1.74720349503904));
#31679=CARTESIAN_POINT('Ctrl Pts',(-0.163814161002474,1.,1.74720349503904));
#31680=CARTESIAN_POINT('Ctrl Pts',(-0.164834765708484,-1.,1.75666056640041));
#31681=CARTESIAN_POINT('Ctrl Pts',(-0.164834765708484,1.,1.75666056640041));
#31682=CARTESIAN_POINT('Ctrl Pts',(-0.166279355148738,-1.,1.77018771687692));
#31683=CARTESIAN_POINT('Ctrl Pts',(-0.166279355148738,1.,1.77018771687692));
#31684=CARTESIAN_POINT('Ctrl Pts',(-0.16803277280837,-1.,1.78690649988931));
#31685=CARTESIAN_POINT('Ctrl Pts',(-0.16803277280837,1.,1.78690649988931));
#31686=CARTESIAN_POINT('Ctrl Pts',(-0.169936923908078,-1.,1.80561530633924));
#31687=CARTESIAN_POINT('Ctrl Pts',(-0.169936923908078,1.,1.80561530633924));
#31688=CARTESIAN_POINT('Ctrl Pts',(-0.171554770207306,-1.,1.82215766815414));
#31689=CARTESIAN_POINT('Ctrl Pts',(-0.171554770207306,1.,1.82215766815414));
#31690=CARTESIAN_POINT('Ctrl Pts',(-0.17288944289442,-1.,1.83658380530747));
#31691=CARTESIAN_POINT('Ctrl Pts',(-0.17288944289442,1.,1.83658380530747));
#31692=CARTESIAN_POINT('Ctrl Pts',(-0.173946627589401,-1.,1.84898113200543));
#31693=CARTESIAN_POINT('Ctrl Pts',(-0.173946627589401,1.,1.84898113200543));
#31694=CARTESIAN_POINT('Ctrl Pts',(-0.174735259276856,-1.,1.85948367089838));
#31695=CARTESIAN_POINT('Ctrl Pts',(-0.174735259276856,1.,1.85948367089838));
#31696=CARTESIAN_POINT('Ctrl Pts',(-0.175268337590901,-1.,1.86828349694972));
#31697=CARTESIAN_POINT('Ctrl Pts',(-0.175268337590901,1.,1.86828349694972));
#31698=CARTESIAN_POINT('Ctrl Pts',(-0.175563480746206,-1.,1.87563767773249));
#31699=CARTESIAN_POINT('Ctrl Pts',(-0.175563480746206,1.,1.87563767773249));
#31700=CARTESIAN_POINT('Ctrl Pts',(-0.175644148889271,-1.,1.88188663144846));
#31701=CARTESIAN_POINT('Ctrl Pts',(-0.175644148889271,1.,1.88188663144846));
#31702=CARTESIAN_POINT('Ctrl Pts',(-0.175538155840286,-1.,1.88742606272818));
#31703=CARTESIAN_POINT('Ctrl Pts',(-0.175538155840286,1.,1.88742606272818));
#31704=CARTESIAN_POINT('Ctrl Pts',(-0.175274276190664,-1.,1.89264630198279));
#31705=CARTESIAN_POINT('Ctrl Pts',(-0.175274276190664,1.,1.89264630198279));
#31706=CARTESIAN_POINT('Ctrl Pts',(-0.174879405091277,-1.,1.89788101117148));
#31707=CARTESIAN_POINT('Ctrl Pts',(-0.174879405091277,1.,1.89788101117148));
#31708=CARTESIAN_POINT('Ctrl Pts',(-0.174375518661222,-1.,1.90335253863003));
#31709=CARTESIAN_POINT('Ctrl Pts',(-0.174375518661222,1.,1.90335253863003));
#31710=CARTESIAN_POINT('Ctrl Pts',(-0.173776635257984,-1.,1.90911693975475));
#31711=CARTESIAN_POINT('Ctrl Pts',(-0.173776635257984,1.,1.90911693975475));
#31712=CARTESIAN_POINT('Ctrl Pts',(-0.173090695383619,-1.,1.91511429159681));
#31713=CARTESIAN_POINT('Ctrl Pts',(-0.173090695383619,1.,1.91511429159681));
#31714=CARTESIAN_POINT('Ctrl Pts',(-0.172321621259557,-1.,1.92122334398034));
#31715=CARTESIAN_POINT('Ctrl Pts',(-0.172321621259557,1.,1.92122334398034));
#31716=CARTESIAN_POINT('Ctrl Pts',(-0.17147119153296,-1.,1.92731093582));
#31717=CARTESIAN_POINT('Ctrl Pts',(-0.17147119153296,1.,1.92731093582));
#31718=CARTESIAN_POINT('Ctrl Pts',(-0.170541253116136,-1.,1.93329183155455));
#31719=CARTESIAN_POINT('Ctrl Pts',(-0.170541253116136,1.,1.93329183155455));
#31720=CARTESIAN_POINT('Ctrl Pts',(-0.169534904817425,-1.,1.93915639211497));
#31721=CARTESIAN_POINT('Ctrl Pts',(-0.169534904817425,1.,1.93915639211497));
#31722=CARTESIAN_POINT('Ctrl Pts',(-0.168455741607516,-1.,1.94493757756879));
#31723=CARTESIAN_POINT('Ctrl Pts',(-0.168455741607516,1.,1.94493757756879));
#31724=CARTESIAN_POINT('Ctrl Pts',(-0.167307501784469,-1.,1.95069027794286));
#31725=CARTESIAN_POINT('Ctrl Pts',(-0.167307501784469,1.,1.95069027794286));
#31726=CARTESIAN_POINT('Ctrl Pts',(-0.166093592002833,-1.,1.95646759718755));
#31727=CARTESIAN_POINT('Ctrl Pts',(-0.166093592002833,1.,1.95646759718755));
#31728=CARTESIAN_POINT('Ctrl Pts',(-0.1648165689203,-1.,1.96229379940174));
#31729=CARTESIAN_POINT('Ctrl Pts',(-0.1648165689203,1.,1.96229379940174));
#31730=CARTESIAN_POINT('Ctrl Pts',(-0.16347818545776,-1.,1.96816512678));
#31731=CARTESIAN_POINT('Ctrl Pts',(-0.16347818545776,1.,1.96816512678));
#31732=CARTESIAN_POINT('Ctrl Pts',(-0.162079693556302,-1.,1.97406280235204));
#31733=CARTESIAN_POINT('Ctrl Pts',(-0.162079693556302,1.,1.97406280235204));
#31734=CARTESIAN_POINT('Ctrl Pts',(-0.16062206078461,-1.,1.97996195437557));
#31735=CARTESIAN_POINT('Ctrl Pts',(-0.16062206078461,1.,1.97996195437557));
#31736=CARTESIAN_POINT('Ctrl Pts',(-0.159106226437289,-1.,1.98584238283279));
#31737=CARTESIAN_POINT('Ctrl Pts',(-0.159106226437289,1.,1.98584238283279));
#31738=CARTESIAN_POINT('Ctrl Pts',(-0.157533331459215,-1.,1.99169810931893));
#31739=CARTESIAN_POINT('Ctrl Pts',(-0.157533331459215,1.,1.99169810931893));
#31740=CARTESIAN_POINT('Ctrl Pts',(-0.155904629548775,-1.,1.99753284771487));
#31741=CARTESIAN_POINT('Ctrl Pts',(-0.155904629548775,1.,1.99753284771487));
#31742=CARTESIAN_POINT('Ctrl Pts',(-0.154221403049719,-1.,2.00335565310539));
#31743=CARTESIAN_POINT('Ctrl Pts',(-0.154221403049719,1.,2.00335565310539));
#31744=CARTESIAN_POINT('Ctrl Pts',(-0.152484883621452,-1.,2.00917680318426));
#31745=CARTESIAN_POINT('Ctrl Pts',(-0.152484883621452,1.,2.00917680318426));
#31746=CARTESIAN_POINT('Ctrl Pts',(-0.150696157673084,-1.,2.01500291940243));
#31747=CARTESIAN_POINT('Ctrl Pts',(-0.150696157673084,1.,2.01500291940243));
#31748=CARTESIAN_POINT('Ctrl Pts',(-0.148856124775343,-1.,2.02083464969897));
#31749=CARTESIAN_POINT('Ctrl Pts',(-0.148856124775343,1.,2.02083464969897));
#31750=CARTESIAN_POINT('Ctrl Pts',(-0.146965557332586,-1.,2.02666926182017));
#31751=CARTESIAN_POINT('Ctrl Pts',(-0.146965557332586,1.,2.02666926182017));
#31752=CARTESIAN_POINT('Ctrl Pts',(-0.145025140186058,-1.,2.03250223739941));
#31753=CARTESIAN_POINT('Ctrl Pts',(-0.145025140186058,1.,2.03250223739941));
#31754=CARTESIAN_POINT('Ctrl Pts',(-0.143035515058208,-1.,2.03832911025913));
#31755=CARTESIAN_POINT('Ctrl Pts',(-0.143035515058208,1.,2.03832911025913));
#31756=CARTESIAN_POINT('Ctrl Pts',(-0.140997332152546,-1.,2.04414757947919));
#31757=CARTESIAN_POINT('Ctrl Pts',(-0.140997332152546,1.,2.04414757947919));
#31758=CARTESIAN_POINT('Ctrl Pts',(-0.138911255368966,-1.,2.04995762001333));
#31759=CARTESIAN_POINT('Ctrl Pts',(-0.138911255368966,1.,2.04995762001333));
#31760=CARTESIAN_POINT('Ctrl Pts',(-0.136777941218044,-1.,2.0557604441427));
#31761=CARTESIAN_POINT('Ctrl Pts',(-0.136777941218044,1.,2.0557604441427));
#31762=CARTESIAN_POINT('Ctrl Pts',(-0.134598026192107,-1.,2.06155781517844));
#31763=CARTESIAN_POINT('Ctrl Pts',(-0.134598026192107,1.,2.06155781517844));
#31764=CARTESIAN_POINT('Ctrl Pts',(-0.13237211154771,-1.,2.06735123910319));
#31765=CARTESIAN_POINT('Ctrl Pts',(-0.13237211154771,1.,2.06735123910319));
#31766=CARTESIAN_POINT('Ctrl Pts',(-0.130100748328401,-1.,2.07314114713047));
#31767=CARTESIAN_POINT('Ctrl Pts',(-0.130100748328401,1.,2.07314114713047));
#31768=CARTESIAN_POINT('Ctrl Pts',(-0.127784445276116,-1.,2.07892715110967));
#31769=CARTESIAN_POINT('Ctrl Pts',(-0.127784445276116,1.,2.07892715110967));
#31770=CARTESIAN_POINT('Ctrl Pts',(-0.125423679412058,-1.,2.08470840653628));
#31771=CARTESIAN_POINT('Ctrl Pts',(-0.125423679412058,1.,2.08470840653628));
#31772=CARTESIAN_POINT('Ctrl Pts',(-0.123018905621083,-1.,2.09048392424826));
#31773=CARTESIAN_POINT('Ctrl Pts',(-0.123018905621083,1.,2.09048392424826));
#31774=CARTESIAN_POINT('Ctrl Pts',(-0.120570567965129,-1.,2.09625292867756));
#31775=CARTESIAN_POINT('Ctrl Pts',(-0.120570567965129,1.,2.09625292867756));
#31776=CARTESIAN_POINT('Ctrl Pts',(-0.118079107988368,-1.,2.10201512132945));
#31777=CARTESIAN_POINT('Ctrl Pts',(-0.118079107988368,1.,2.10201512132945));
#31778=CARTESIAN_POINT('Ctrl Pts',(-0.115544957687941,-1.,2.10777050261359));
#31779=CARTESIAN_POINT('Ctrl Pts',(-0.115544957687941,1.,2.10777050261359));
#31780=CARTESIAN_POINT('Ctrl Pts',(-0.112968534419746,-1.,2.11351924490335));
#31781=CARTESIAN_POINT('Ctrl Pts',(-0.112968534419746,1.,2.11351924490335));
#31782=CARTESIAN_POINT('Ctrl Pts',(-0.11035023613502,-1.,2.11926155590849));
#31783=CARTESIAN_POINT('Ctrl Pts',(-0.11035023613502,1.,2.11926155590849));
#31784=CARTESIAN_POINT('Ctrl Pts',(-0.107690435231068,-1.,2.12499752306927));
#31785=CARTESIAN_POINT('Ctrl Pts',(-0.107690435231068,1.,2.12499752306927));
#31786=CARTESIAN_POINT('Ctrl Pts',(-0.104989479152703,-1.,2.1307270488718));
#31787=CARTESIAN_POINT('Ctrl Pts',(-0.104989479152703,1.,2.1307270488718));
#31788=CARTESIAN_POINT('Ctrl Pts',(-0.102247700556064,-1.,2.13644992667052));
#31789=CARTESIAN_POINT('Ctrl Pts',(-0.102247700556064,1.,2.13644992667052));
#31790=CARTESIAN_POINT('Ctrl Pts',(-0.0994654261990745,-1.,2.14216588395974));
#31791=CARTESIAN_POINT('Ctrl Pts',(-0.0994654261990745,1.,2.14216588395974));
#31792=CARTESIAN_POINT('Ctrl Pts',(-0.0966429852305691,-1.,2.14787463531864));
#31793=CARTESIAN_POINT('Ctrl Pts',(-0.0966429852305691,1.,2.14787463531864));
#31794=CARTESIAN_POINT('Ctrl Pts',(-0.0937807218868348,-1.,2.15357593978377));
#31795=CARTESIAN_POINT('Ctrl Pts',(-0.0937807218868348,1.,2.15357593978377));
#31796=CARTESIAN_POINT('Ctrl Pts',(-0.0908789888108269,-1.,2.15926961544808));
#31797=CARTESIAN_POINT('Ctrl Pts',(-0.0908789888108269,1.,2.15926961544808));
#31798=CARTESIAN_POINT('Ctrl Pts',(-0.0879381291387825,-1.,2.16495552645275));
#31799=CARTESIAN_POINT('Ctrl Pts',(-0.0879381291387825,1.,2.16495552645275));
#31800=CARTESIAN_POINT('Ctrl Pts',(-0.0849584620835646,-1.,2.17063357871031));
#31801=CARTESIAN_POINT('Ctrl Pts',(-0.0849584620835646,1.,2.17063357871031));
#31802=CARTESIAN_POINT('Ctrl Pts',(-0.0819402680871942,-1.,2.1763037121106));
#31803=CARTESIAN_POINT('Ctrl Pts',(-0.0819402680871942,1.,2.1763037121106));
#31804=CARTESIAN_POINT('Ctrl Pts',(-0.078883772768323,-1.,2.18196589448304));
#31805=CARTESIAN_POINT('Ctrl Pts',(-0.078883772768323,1.,2.18196589448304));
#31806=CARTESIAN_POINT('Ctrl Pts',(-0.0757891465833414,-1.,2.1876201139874));
#31807=CARTESIAN_POINT('Ctrl Pts',(-0.0757891465833414,1.,2.1876201139874));
#31808=CARTESIAN_POINT('Ctrl Pts',(-0.0732830357304279,-1.,2.19213712012956));
#31809=CARTESIAN_POINT('Ctrl Pts',(-0.0732830357304279,1.,2.19213712012956));
#31810=CARTESIAN_POINT('Ctrl Pts',(-0.071386377952463,-1.,2.19552129483562));
#31811=CARTESIAN_POINT('Ctrl Pts',(-0.071386377952463,1.,2.19552129483562));
#31812=CARTESIAN_POINT('Ctrl Pts',(-0.0701143536324929,-1.,2.19777582085261));
#31813=CARTESIAN_POINT('Ctrl Pts',(-0.0701143536324929,1.,2.19777582085261));
#31814=CARTESIAN_POINT('Ctrl Pts',(-0.0694764450219586,-1.,2.19890268624765));
#31815=CARTESIAN_POINT('Ctrl Pts',(-0.0694764450219586,1.,2.19890268624765));
#31816=CARTESIAN_POINT('',(-0.163289472382896,1.,1.74236521665491));
#31817=CARTESIAN_POINT('Ctrl Pts',(-0.163289472382896,1.,1.74236521665491));
#31818=CARTESIAN_POINT('Ctrl Pts',(-0.163814161002474,1.,1.74720349503904));
#31819=CARTESIAN_POINT('Ctrl Pts',(-0.164834765708484,1.,1.75666056640041));
#31820=CARTESIAN_POINT('Ctrl Pts',(-0.166279355148738,1.,1.77018771687692));
#31821=CARTESIAN_POINT('Ctrl Pts',(-0.16803277280837,1.,1.78690649988931));
#31822=CARTESIAN_POINT('Ctrl Pts',(-0.169936923908078,1.,1.80561530633924));
#31823=CARTESIAN_POINT('Ctrl Pts',(-0.171554770207306,1.,1.82215766815414));
#31824=CARTESIAN_POINT('Ctrl Pts',(-0.17288944289442,1.,1.83658380530747));
#31825=CARTESIAN_POINT('Ctrl Pts',(-0.173946627589401,1.,1.84898113200543));
#31826=CARTESIAN_POINT('Ctrl Pts',(-0.174735259276856,1.,1.85948367089838));
#31827=CARTESIAN_POINT('Ctrl Pts',(-0.175268337590901,1.,1.86828349694972));
#31828=CARTESIAN_POINT('Ctrl Pts',(-0.175563480746206,1.,1.87563767773249));
#31829=CARTESIAN_POINT('Ctrl Pts',(-0.175644148889271,1.,1.88188663144846));
#31830=CARTESIAN_POINT('Ctrl Pts',(-0.175538155840286,1.,1.88742606272818));
#31831=CARTESIAN_POINT('Ctrl Pts',(-0.175274276190664,1.,1.89264630198279));
#31832=CARTESIAN_POINT('Ctrl Pts',(-0.174879405091277,1.,1.89788101117148));
#31833=CARTESIAN_POINT('Ctrl Pts',(-0.174375518661222,1.,1.90335253863003));
#31834=CARTESIAN_POINT('Ctrl Pts',(-0.173776635257984,1.,1.90911693975475));
#31835=CARTESIAN_POINT('Ctrl Pts',(-0.173090695383619,1.,1.91511429159681));
#31836=CARTESIAN_POINT('Ctrl Pts',(-0.172321621259557,1.,1.92122334398034));
#31837=CARTESIAN_POINT('Ctrl Pts',(-0.17147119153296,1.,1.92731093582));
#31838=CARTESIAN_POINT('Ctrl Pts',(-0.170541253116136,1.,1.93329183155455));
#31839=CARTESIAN_POINT('Ctrl Pts',(-0.169534904817425,1.,1.93915639211497));
#31840=CARTESIAN_POINT('Ctrl Pts',(-0.168455741607516,1.,1.94493757756879));
#31841=CARTESIAN_POINT('Ctrl Pts',(-0.167307501784469,1.,1.95069027794286));
#31842=CARTESIAN_POINT('Ctrl Pts',(-0.166093592002833,1.,1.95646759718755));
#31843=CARTESIAN_POINT('Ctrl Pts',(-0.1648165689203,1.,1.96229379940174));
#31844=CARTESIAN_POINT('Ctrl Pts',(-0.16347818545776,1.,1.96816512678));
#31845=CARTESIAN_POINT('Ctrl Pts',(-0.162079693556302,1.,1.97406280235204));
#31846=CARTESIAN_POINT('Ctrl Pts',(-0.16062206078461,1.,1.97996195437557));
#31847=CARTESIAN_POINT('Ctrl Pts',(-0.159106226437289,1.,1.98584238283279));
#31848=CARTESIAN_POINT('Ctrl Pts',(-0.157533331459215,1.,1.99169810931893));
#31849=CARTESIAN_POINT('Ctrl Pts',(-0.155904629548775,1.,1.99753284771487));
#31850=CARTESIAN_POINT('Ctrl Pts',(-0.154221403049719,1.,2.00335565310539));
#31851=CARTESIAN_POINT('Ctrl Pts',(-0.152484883621452,1.,2.00917680318426));
#31852=CARTESIAN_POINT('Ctrl Pts',(-0.150696157673084,1.,2.01500291940243));
#31853=CARTESIAN_POINT('Ctrl Pts',(-0.148856124775343,1.,2.02083464969897));
#31854=CARTESIAN_POINT('Ctrl Pts',(-0.146965557332586,1.,2.02666926182017));
#31855=CARTESIAN_POINT('Ctrl Pts',(-0.145025140186058,1.,2.03250223739941));
#31856=CARTESIAN_POINT('Ctrl Pts',(-0.143035515058208,1.,2.03832911025913));
#31857=CARTESIAN_POINT('Ctrl Pts',(-0.140997332152546,1.,2.04414757947919));
#31858=CARTESIAN_POINT('Ctrl Pts',(-0.138911255368966,1.,2.04995762001333));
#31859=CARTESIAN_POINT('Ctrl Pts',(-0.136777941218044,1.,2.0557604441427));
#31860=CARTESIAN_POINT('Ctrl Pts',(-0.134598026192107,1.,2.06155781517844));
#31861=CARTESIAN_POINT('Ctrl Pts',(-0.13237211154771,1.,2.06735123910319));
#31862=CARTESIAN_POINT('Ctrl Pts',(-0.130100748328401,1.,2.07314114713047));
#31863=CARTESIAN_POINT('Ctrl Pts',(-0.127784445276116,1.,2.07892715110967));
#31864=CARTESIAN_POINT('Ctrl Pts',(-0.125423679412058,1.,2.08470840653628));
#31865=CARTESIAN_POINT('Ctrl Pts',(-0.123018905621083,1.,2.09048392424826));
#31866=CARTESIAN_POINT('Ctrl Pts',(-0.120570567965129,1.,2.09625292867756));
#31867=CARTESIAN_POINT('Ctrl Pts',(-0.118079107988368,1.,2.10201512132945));
#31868=CARTESIAN_POINT('Ctrl Pts',(-0.115544957687941,1.,2.10777050261359));
#31869=CARTESIAN_POINT('Ctrl Pts',(-0.112968534419746,1.,2.11351924490335));
#31870=CARTESIAN_POINT('Ctrl Pts',(-0.11035023613502,1.,2.11926155590849));
#31871=CARTESIAN_POINT('Ctrl Pts',(-0.107690435231068,1.,2.12499752306927));
#31872=CARTESIAN_POINT('Ctrl Pts',(-0.104989479152703,1.,2.1307270488718));
#31873=CARTESIAN_POINT('Ctrl Pts',(-0.102247700556064,1.,2.13644992667052));
#31874=CARTESIAN_POINT('Ctrl Pts',(-0.0994654261990745,1.,2.14216588395974));
#31875=CARTESIAN_POINT('Ctrl Pts',(-0.0966429852305691,1.,2.14787463531864));
#31876=CARTESIAN_POINT('Ctrl Pts',(-0.0937807218868348,1.,2.15357593978377));
#31877=CARTESIAN_POINT('Ctrl Pts',(-0.0908789888108269,1.,2.15926961544808));
#31878=CARTESIAN_POINT('Ctrl Pts',(-0.0879381291387825,1.,2.16495552645275));
#31879=CARTESIAN_POINT('Ctrl Pts',(-0.0849584620835646,1.,2.17063357871031));
#31880=CARTESIAN_POINT('Ctrl Pts',(-0.0819402680871942,1.,2.1763037121106));
#31881=CARTESIAN_POINT('Ctrl Pts',(-0.078883772768323,1.,2.18196589448304));
#31882=CARTESIAN_POINT('Ctrl Pts',(-0.0757891465833414,1.,2.1876201139874));
#31883=CARTESIAN_POINT('Ctrl Pts',(-0.0732830357304279,1.,2.19213712012956));
#31884=CARTESIAN_POINT('Ctrl Pts',(-0.071386377952463,1.,2.19552129483562));
#31885=CARTESIAN_POINT('Ctrl Pts',(-0.0701143536324929,1.,2.19777582085261));
#31886=CARTESIAN_POINT('Ctrl Pts',(-0.0694764450219586,1.,2.19890268624765));
#31887=CARTESIAN_POINT('',(-0.163289472382897,0.,1.74236521665491));
#31888=CARTESIAN_POINT('Origin',(0.,0.,0.));
#31889=CARTESIAN_POINT('',(-0.383122945602004,1.,1.7075470150345));
#31890=CARTESIAN_POINT('Origin',(0.,1.,0.));
#31891=CARTESIAN_POINT('',(-0.383122945602004,0.,1.7075470150345));
#31892=CARTESIAN_POINT('Ctrl Pts',(-0.61342227326009,-1.,2.11275013067528));
#31893=CARTESIAN_POINT('Ctrl Pts',(-0.61342227326009,1.,2.11275013067528));
#31894=CARTESIAN_POINT('Ctrl Pts',(-0.61246736556225,-1.,2.11187554260142));
#31895=CARTESIAN_POINT('Ctrl Pts',(-0.61246736556225,1.,2.11187554260142));
#31896=CARTESIAN_POINT('Ctrl Pts',(-0.610560911691113,-1.,2.11012443807661));
#31897=CARTESIAN_POINT('Ctrl Pts',(-0.610560911691113,1.,2.11012443807661));
#31898=CARTESIAN_POINT('Ctrl Pts',(-0.607711315456826,-1.,2.10749199615859));
#31899=CARTESIAN_POINT('Ctrl Pts',(-0.607711315456826,1.,2.10749199615859));
#31900=CARTESIAN_POINT('Ctrl Pts',(-0.603932030738212,-1.,2.10397049887709));
#31901=CARTESIAN_POINT('Ctrl Pts',(-0.603932030738212,1.,2.10397049887709));
#31902=CARTESIAN_POINT('Ctrl Pts',(-0.599241616422144,-1.,2.09954930865331));
#31903=CARTESIAN_POINT('Ctrl Pts',(-0.599241616422144,1.,2.09954930865331));
#31904=CARTESIAN_POINT('Ctrl Pts',(-0.594585006052824,-1.,2.09510876220501));
#31905=CARTESIAN_POINT('Ctrl Pts',(-0.594585006052824,1.,2.09510876220501));
#31906=CARTESIAN_POINT('Ctrl Pts',(-0.589962365403189,-1.,2.09064881812053));
#31907=CARTESIAN_POINT('Ctrl Pts',(-0.589962365403189,1.,2.09064881812053));
#31908=CARTESIAN_POINT('Ctrl Pts',(-0.585373918990895,-1.,2.086169437277));
#31909=CARTESIAN_POINT('Ctrl Pts',(-0.585373918990895,1.,2.086169437277));
#31910=CARTESIAN_POINT('Ctrl Pts',(-0.580819952107257,-1.,2.08167059018138));
#31911=CARTESIAN_POINT('Ctrl Pts',(-0.580819952107257,1.,2.08167059018138));
#31912=CARTESIAN_POINT('Ctrl Pts',(-0.576300797416275,-1.,2.07715226767361));
#31913=CARTESIAN_POINT('Ctrl Pts',(-0.576300797416275,1.,2.07715226767361));
#31914=CARTESIAN_POINT('Ctrl Pts',(-0.571816823242411,-1.,2.07261449292757));
#31915=CARTESIAN_POINT('Ctrl Pts',(-0.571816823242411,1.,2.07261449292757));
#31916=CARTESIAN_POINT('Ctrl Pts',(-0.567368421181229,-1.,2.06805732997383));
#31917=CARTESIAN_POINT('Ctrl Pts',(-0.567368421181229,1.,2.06805732997383));
#31918=CARTESIAN_POINT('Ctrl Pts',(-0.562955993082574,-1.,2.06348090160697));
#31919=CARTESIAN_POINT('Ctrl Pts',(-0.562955993082574,1.,2.06348090160697));
#31920=CARTESIAN_POINT('Ctrl Pts',(-0.558579940185467,-1.,2.05888537756571));
#31921=CARTESIAN_POINT('Ctrl Pts',(-0.558579940185467,1.,2.05888537756571));
#31922=CARTESIAN_POINT('Ctrl Pts',(-0.55424065746411,-1.,2.05427091604482));
#31923=CARTESIAN_POINT('Ctrl Pts',(-0.55424065746411,1.,2.05427091604482));
#31924=CARTESIAN_POINT('Ctrl Pts',(-0.549938525150342,-1.,2.04963761077974));
#31925=CARTESIAN_POINT('Ctrl Pts',(-0.549938525150342,1.,2.04963761077974));
#31926=CARTESIAN_POINT('Ctrl Pts',(-0.545673903817348,-1.,2.0449854471456));
#31927=CARTESIAN_POINT('Ctrl Pts',(-0.545673903817348,1.,2.0449854471456));
#31928=CARTESIAN_POINT('Ctrl Pts',(-0.54144712061552,-1.,2.0403142269048));
#31929=CARTESIAN_POINT('Ctrl Pts',(-0.54144712061552,1.,2.0403142269048));
#31930=CARTESIAN_POINT('Ctrl Pts',(-0.537258489833134,-1.,2.03562362953993));
#31931=CARTESIAN_POINT('Ctrl Pts',(-0.537258489833134,1.,2.03562362953993));
#31932=CARTESIAN_POINT('Ctrl Pts',(-0.533108355132905,-1.,2.03091336214401));
#31933=CARTESIAN_POINT('Ctrl Pts',(-0.533108355132905,1.,2.03091336214401));
#31934=CARTESIAN_POINT('Ctrl Pts',(-0.528997127241911,-1.,2.02618329083289));
#31935=CARTESIAN_POINT('Ctrl Pts',(-0.528997127241911,1.,2.02618329083289));
#31936=CARTESIAN_POINT('Ctrl Pts',(-0.524925318333518,-1.,2.02143356304712));
#31937=CARTESIAN_POINT('Ctrl Pts',(-0.524925318333518,1.,2.02143356304712));
#31938=CARTESIAN_POINT('Ctrl Pts',(-0.520893590399428,-1.,2.01666477917305));
#31939=CARTESIAN_POINT('Ctrl Pts',(-0.520893590399428,1.,2.01666477917305));
#31940=CARTESIAN_POINT('Ctrl Pts',(-0.516902681728733,-1.,2.01187773939257));
#31941=CARTESIAN_POINT('Ctrl Pts',(-0.516902681728733,1.,2.01187773939257));
#31942=CARTESIAN_POINT('Ctrl Pts',(-0.512953306961814,-1.,2.00707309946955));
#31943=CARTESIAN_POINT('Ctrl Pts',(-0.512953306961814,1.,2.00707309946955));
#31944=CARTESIAN_POINT('Ctrl Pts',(-0.509046069886152,-1.,2.00225107134733));
#31945=CARTESIAN_POINT('Ctrl Pts',(-0.509046069886152,1.,2.00225107134733));
#31946=CARTESIAN_POINT('Ctrl Pts',(-0.505181361323011,-1.,1.99741107463567));
#31947=CARTESIAN_POINT('Ctrl Pts',(-0.505181361323011,1.,1.99741107463567));
#31948=CARTESIAN_POINT('Ctrl Pts',(-0.501359287727129,-1.,1.9925514912615));
#31949=CARTESIAN_POINT('Ctrl Pts',(-0.501359287727129,1.,1.9925514912615));
#31950=CARTESIAN_POINT('Ctrl Pts',(-0.497579909545564,-1.,1.98767044752929));
#31951=CARTESIAN_POINT('Ctrl Pts',(-0.497579909545564,1.,1.98767044752929));
#31952=CARTESIAN_POINT('Ctrl Pts',(-0.493843476541492,-1.,1.9827665876182));
#31953=CARTESIAN_POINT('Ctrl Pts',(-0.493843476541492,1.,1.9827665876182));
#31954=CARTESIAN_POINT('Ctrl Pts',(-0.490150627860955,-1.,1.97783973019229));
#31955=CARTESIAN_POINT('Ctrl Pts',(-0.490150627860955,1.,1.97783973019229));
#31956=CARTESIAN_POINT('Ctrl Pts',(-0.486502692907661,-1.,1.97289186263272));
#31957=CARTESIAN_POINT('Ctrl Pts',(-0.486502692907661,1.,1.97289186263272));
#31958=CARTESIAN_POINT('Ctrl Pts',(-0.482901662120687,-1.,1.96792703422358));
#31959=CARTESIAN_POINT('Ctrl Pts',(-0.482901662120687,1.,1.96792703422358));
#31960=CARTESIAN_POINT('Ctrl Pts',(-0.479349583074846,-1.,1.96294933055938));
#31961=CARTESIAN_POINT('Ctrl Pts',(-0.479349583074846,1.,1.96294933055938));
#31962=CARTESIAN_POINT('Ctrl Pts',(-0.475848034683172,-1.,1.95796111148175));
#31963=CARTESIAN_POINT('Ctrl Pts',(-0.475848034683172,1.,1.95796111148175));
#31964=CARTESIAN_POINT('Ctrl Pts',(-0.47239767226408,-1.,1.95296148278136));
#31965=CARTESIAN_POINT('Ctrl Pts',(-0.47239767226408,1.,1.95296148278136));
#31966=CARTESIAN_POINT('Ctrl Pts',(-0.468997482913158,-1.,1.94794381136524));
#31967=CARTESIAN_POINT('Ctrl Pts',(-0.468997482913158,1.,1.94794381136524));
#31968=CARTESIAN_POINT('Ctrl Pts',(-0.465645462026065,-1.,1.94289794196205));
#31969=CARTESIAN_POINT('Ctrl Pts',(-0.465645462026065,1.,1.94289794196205));
#31970=CARTESIAN_POINT('Ctrl Pts',(-0.462340031009087,-1.,1.93781486640834));
#31971=CARTESIAN_POINT('Ctrl Pts',(-0.462340031009087,1.,1.93781486640834));
#31972=CARTESIAN_POINT('Ctrl Pts',(-0.459081234547931,-1.,1.93269066517936));
#31973=CARTESIAN_POINT('Ctrl Pts',(-0.459081234547931,1.,1.93269066517936));
#31974=CARTESIAN_POINT('Ctrl Pts',(-0.455872005174335,-1.,1.92753067150461));
#31975=CARTESIAN_POINT('Ctrl Pts',(-0.455872005174335,1.,1.92753067150461));
#31976=CARTESIAN_POINT('Ctrl Pts',(-0.452719478359356,-1.,1.9223538064847));
#31977=CARTESIAN_POINT('Ctrl Pts',(-0.452719478359356,1.,1.9223538064847));
#31978=CARTESIAN_POINT('Ctrl Pts',(-0.449632260106572,-1.,1.91718342555717));
#31979=CARTESIAN_POINT('Ctrl Pts',(-0.449632260106572,1.,1.91718342555717));
#31980=CARTESIAN_POINT('Ctrl Pts',(-0.446617343485651,-1.,1.91203699981095));
#31981=CARTESIAN_POINT('Ctrl Pts',(-0.446617343485651,1.,1.91203699981095));
#31982=CARTESIAN_POINT('Ctrl Pts',(-0.44367755684917,-1.,1.90691756144906));
#31983=CARTESIAN_POINT('Ctrl Pts',(-0.44367755684917,1.,1.90691756144906));
#31984=CARTESIAN_POINT('Ctrl Pts',(-0.440807833704161,-1.,1.90180124389137));
#31985=CARTESIAN_POINT('Ctrl Pts',(-0.440807833704161,1.,1.90180124389137));
#31986=CARTESIAN_POINT('Ctrl Pts',(-0.437995003948443,-1.,1.89663648956549));
#31987=CARTESIAN_POINT('Ctrl Pts',(-0.437995003948443,1.,1.89663648956549));
#31988=CARTESIAN_POINT('Ctrl Pts',(-0.43522566096358,-1.,1.89136993975585));
#31989=CARTESIAN_POINT('Ctrl Pts',(-0.43522566096358,1.,1.89136993975585));
#31990=CARTESIAN_POINT('Ctrl Pts',(-0.432493038548833,-1.,1.88596913666828));
#31991=CARTESIAN_POINT('Ctrl Pts',(-0.432493038548833,1.,1.88596913666828));
#31992=CARTESIAN_POINT('Ctrl Pts',(-0.429803062482217,-1.,1.88044229001778));
#31993=CARTESIAN_POINT('Ctrl Pts',(-0.429803062482217,1.,1.88044229001778));
#31994=CARTESIAN_POINT('Ctrl Pts',(-0.427183828518743,-1.,1.87486989291333));
#31995=CARTESIAN_POINT('Ctrl Pts',(-0.427183828518743,1.,1.87486989291333));
#31996=CARTESIAN_POINT('Ctrl Pts',(-0.424678177290876,-1.,1.8693780394412));
#31997=CARTESIAN_POINT('Ctrl Pts',(-0.424678177290876,1.,1.8693780394412));
#31998=CARTESIAN_POINT('Ctrl Pts',(-0.422327307417885,-1.,1.86408083333863));
#31999=CARTESIAN_POINT('Ctrl Pts',(-0.422327307417885,1.,1.86408083333863));
#32000=CARTESIAN_POINT('Ctrl Pts',(-0.420157287975583,-1.,1.8590328109667));
#32001=CARTESIAN_POINT('Ctrl Pts',(-0.420157287975583,1.,1.8590328109667));
#32002=CARTESIAN_POINT('Ctrl Pts',(-0.418164129144045,-1.,1.8541763285645));
#32003=CARTESIAN_POINT('Ctrl Pts',(-0.418164129144045,1.,1.8541763285645));
#32004=CARTESIAN_POINT('Ctrl Pts',(-0.416300022039885,-1.,1.84929312930314));
#32005=CARTESIAN_POINT('Ctrl Pts',(-0.416300022039885,1.,1.84929312930314));
#32006=CARTESIAN_POINT('Ctrl Pts',(-0.414487438255542,-1.,1.84405757074218));
#32007=CARTESIAN_POINT('Ctrl Pts',(-0.414487438255542,1.,1.84405757074218));
#32008=CARTESIAN_POINT('Ctrl Pts',(-0.412633125322945,-1.,1.8380895347617));
#32009=CARTESIAN_POINT('Ctrl Pts',(-0.412633125322945,1.,1.8380895347617));
#32010=CARTESIAN_POINT('Ctrl Pts',(-0.410641256301276,-1.,1.83100408895047));
#32011=CARTESIAN_POINT('Ctrl Pts',(-0.410641256301276,1.,1.83100408895047));
#32012=CARTESIAN_POINT('Ctrl Pts',(-0.408428948106227,-1.,1.82247022677562));
#32013=CARTESIAN_POINT('Ctrl Pts',(-0.408428948106227,1.,1.82247022677562));
#32014=CARTESIAN_POINT('Ctrl Pts',(-0.405933518407175,-1.,1.81223801812013));
#32015=CARTESIAN_POINT('Ctrl Pts',(-0.405933518407175,1.,1.81223801812013));
#32016=CARTESIAN_POINT('Ctrl Pts',(-0.403107976163396,-1.,1.80012077173238));
#32017=CARTESIAN_POINT('Ctrl Pts',(-0.403107976163396,1.,1.80012077173238));
#32018=CARTESIAN_POINT('Ctrl Pts',(-0.399919403774155,-1.,1.78598826343754));
#32019=CARTESIAN_POINT('Ctrl Pts',(-0.399919403774155,1.,1.78598826343754));
#32020=CARTESIAN_POINT('Ctrl Pts',(-0.396346196110688,-1.,1.76975560043442));
#32021=CARTESIAN_POINT('Ctrl Pts',(-0.396346196110688,1.,1.76975560043442));
#32022=CARTESIAN_POINT('Ctrl Pts',(-0.392375812285395,-1.,1.75137405310193));
#32023=CARTESIAN_POINT('Ctrl Pts',(-0.392375812285395,1.,1.75137405310193));
#32024=CARTESIAN_POINT('Ctrl Pts',(-0.388877023502615,-1.,1.73493170972829));
#32025=CARTESIAN_POINT('Ctrl Pts',(-0.388877023502615,1.,1.73493170972829));
#32026=CARTESIAN_POINT('Ctrl Pts',(-0.386070790323281,-1.,1.72162022244582));
#32027=CARTESIAN_POINT('Ctrl Pts',(-0.386070790323281,1.,1.72162022244582));
#32028=CARTESIAN_POINT('Ctrl Pts',(-0.384119047314215,-1.,1.71231062891398));
#32029=CARTESIAN_POINT('Ctrl Pts',(-0.384119047314215,1.,1.71231062891398));
#32030=CARTESIAN_POINT('Ctrl Pts',(-0.383122945602004,-1.,1.7075470150345));
#32031=CARTESIAN_POINT('Ctrl Pts',(-0.383122945602004,1.,1.7075470150345));
#32032=CARTESIAN_POINT('',(-0.61342227326009,1.,2.11275013067528));
#32033=CARTESIAN_POINT('Ctrl Pts',(-0.61342227326009,1.,2.11275013067528));
#32034=CARTESIAN_POINT('Ctrl Pts',(-0.61246736556225,1.,2.11187554260142));
#32035=CARTESIAN_POINT('Ctrl Pts',(-0.610560911691113,1.,2.11012443807661));
#32036=CARTESIAN_POINT('Ctrl Pts',(-0.607711315456826,1.,2.10749199615859));
#32037=CARTESIAN_POINT('Ctrl Pts',(-0.603932030738212,1.,2.10397049887709));
#32038=CARTESIAN_POINT('Ctrl Pts',(-0.599241616422144,1.,2.09954930865331));
#32039=CARTESIAN_POINT('Ctrl Pts',(-0.594585006052824,1.,2.09510876220501));
#32040=CARTESIAN_POINT('Ctrl Pts',(-0.589962365403189,1.,2.09064881812053));
#32041=CARTESIAN_POINT('Ctrl Pts',(-0.585373918990895,1.,2.086169437277));
#32042=CARTESIAN_POINT('Ctrl Pts',(-0.580819952107257,1.,2.08167059018138));
#32043=CARTESIAN_POINT('Ctrl Pts',(-0.576300797416275,1.,2.07715226767361));
#32044=CARTESIAN_POINT('Ctrl Pts',(-0.571816823242411,1.,2.07261449292757));
#32045=CARTESIAN_POINT('Ctrl Pts',(-0.567368421181229,1.,2.06805732997383));
#32046=CARTESIAN_POINT('Ctrl Pts',(-0.562955993082574,1.,2.06348090160697));
#32047=CARTESIAN_POINT('Ctrl Pts',(-0.558579940185467,1.,2.05888537756571));
#32048=CARTESIAN_POINT('Ctrl Pts',(-0.55424065746411,1.,2.05427091604482));
#32049=CARTESIAN_POINT('Ctrl Pts',(-0.549938525150342,1.,2.04963761077974));
#32050=CARTESIAN_POINT('Ctrl Pts',(-0.545673903817348,1.,2.0449854471456));
#32051=CARTESIAN_POINT('Ctrl Pts',(-0.54144712061552,1.,2.0403142269048));
#32052=CARTESIAN_POINT('Ctrl Pts',(-0.537258489833134,1.,2.03562362953993));
#32053=CARTESIAN_POINT('Ctrl Pts',(-0.533108355132905,1.,2.03091336214401));
#32054=CARTESIAN_POINT('Ctrl Pts',(-0.528997127241911,1.,2.02618329083289));
#32055=CARTESIAN_POINT('Ctrl Pts',(-0.524925318333518,1.,2.02143356304712));
#32056=CARTESIAN_POINT('Ctrl Pts',(-0.520893590399428,1.,2.01666477917305));
#32057=CARTESIAN_POINT('Ctrl Pts',(-0.516902681728733,1.,2.01187773939257));
#32058=CARTESIAN_POINT('Ctrl Pts',(-0.512953306961814,1.,2.00707309946955));
#32059=CARTESIAN_POINT('Ctrl Pts',(-0.509046069886152,1.,2.00225107134733));
#32060=CARTESIAN_POINT('Ctrl Pts',(-0.505181361323011,1.,1.99741107463567));
#32061=CARTESIAN_POINT('Ctrl Pts',(-0.501359287727129,1.,1.9925514912615));
#32062=CARTESIAN_POINT('Ctrl Pts',(-0.497579909545564,1.,1.98767044752929));
#32063=CARTESIAN_POINT('Ctrl Pts',(-0.493843476541492,1.,1.9827665876182));
#32064=CARTESIAN_POINT('Ctrl Pts',(-0.490150627860955,1.,1.97783973019229));
#32065=CARTESIAN_POINT('Ctrl Pts',(-0.486502692907661,1.,1.97289186263272));
#32066=CARTESIAN_POINT('Ctrl Pts',(-0.482901662120687,1.,1.96792703422358));
#32067=CARTESIAN_POINT('Ctrl Pts',(-0.479349583074846,1.,1.96294933055938));
#32068=CARTESIAN_POINT('Ctrl Pts',(-0.475848034683172,1.,1.95796111148175));
#32069=CARTESIAN_POINT('Ctrl Pts',(-0.47239767226408,1.,1.95296148278136));
#32070=CARTESIAN_POINT('Ctrl Pts',(-0.468997482913158,1.,1.94794381136524));
#32071=CARTESIAN_POINT('Ctrl Pts',(-0.465645462026065,1.,1.94289794196205));
#32072=CARTESIAN_POINT('Ctrl Pts',(-0.462340031009087,1.,1.93781486640834));
#32073=CARTESIAN_POINT('Ctrl Pts',(-0.459081234547931,1.,1.93269066517936));
#32074=CARTESIAN_POINT('Ctrl Pts',(-0.455872005174335,1.,1.92753067150461));
#32075=CARTESIAN_POINT('Ctrl Pts',(-0.452719478359356,1.,1.9223538064847));
#32076=CARTESIAN_POINT('Ctrl Pts',(-0.449632260106572,1.,1.91718342555717));
#32077=CARTESIAN_POINT('Ctrl Pts',(-0.446617343485651,1.,1.91203699981095));
#32078=CARTESIAN_POINT('Ctrl Pts',(-0.44367755684917,1.,1.90691756144906));
#32079=CARTESIAN_POINT('Ctrl Pts',(-0.440807833704161,1.,1.90180124389137));
#32080=CARTESIAN_POINT('Ctrl Pts',(-0.437995003948443,1.,1.89663648956549));
#32081=CARTESIAN_POINT('Ctrl Pts',(-0.43522566096358,1.,1.89136993975585));
#32082=CARTESIAN_POINT('Ctrl Pts',(-0.432493038548833,1.,1.88596913666828));
#32083=CARTESIAN_POINT('Ctrl Pts',(-0.429803062482217,1.,1.88044229001778));
#32084=CARTESIAN_POINT('Ctrl Pts',(-0.427183828518743,1.,1.87486989291333));
#32085=CARTESIAN_POINT('Ctrl Pts',(-0.424678177290876,1.,1.8693780394412));
#32086=CARTESIAN_POINT('Ctrl Pts',(-0.422327307417885,1.,1.86408083333863));
#32087=CARTESIAN_POINT('Ctrl Pts',(-0.420157287975583,1.,1.8590328109667));
#32088=CARTESIAN_POINT('Ctrl Pts',(-0.418164129144045,1.,1.8541763285645));
#32089=CARTESIAN_POINT('Ctrl Pts',(-0.416300022039885,1.,1.84929312930314));
#32090=CARTESIAN_POINT('Ctrl Pts',(-0.414487438255542,1.,1.84405757074218));
#32091=CARTESIAN_POINT('Ctrl Pts',(-0.412633125322945,1.,1.8380895347617));
#32092=CARTESIAN_POINT('Ctrl Pts',(-0.410641256301276,1.,1.83100408895047));
#32093=CARTESIAN_POINT('Ctrl Pts',(-0.408428948106227,1.,1.82247022677562));
#32094=CARTESIAN_POINT('Ctrl Pts',(-0.405933518407175,1.,1.81223801812013));
#32095=CARTESIAN_POINT('Ctrl Pts',(-0.403107976163396,1.,1.80012077173238));
#32096=CARTESIAN_POINT('Ctrl Pts',(-0.399919403774155,1.,1.78598826343754));
#32097=CARTESIAN_POINT('Ctrl Pts',(-0.396346196110688,1.,1.76975560043442));
#32098=CARTESIAN_POINT('Ctrl Pts',(-0.392375812285395,1.,1.75137405310193));
#32099=CARTESIAN_POINT('Ctrl Pts',(-0.388877023502615,1.,1.73493170972829));
#32100=CARTESIAN_POINT('Ctrl Pts',(-0.386070790323281,1.,1.72162022244582));
#32101=CARTESIAN_POINT('Ctrl Pts',(-0.384119047314215,1.,1.71231062891398));
#32102=CARTESIAN_POINT('Ctrl Pts',(-0.383122945602004,1.,1.7075470150345));
#32103=CARTESIAN_POINT('',(-0.61342227326009,0.,2.11275013067528));
#32104=CARTESIAN_POINT('Origin',(-0.745574324794401,0.,2.0698113262342));
#32105=CARTESIAN_POINT('',(-0.745574324794401,1.,2.0698113262342));
#32106=CARTESIAN_POINT('',(-0.61342227326009,1.,2.11275013067528));
#32107=CARTESIAN_POINT('',(-0.745574324794401,0.,2.0698113262342));
#32108=CARTESIAN_POINT('Ctrl Pts',(-0.693717979106306,-1.,1.60662857109684));
#32109=CARTESIAN_POINT('Ctrl Pts',(-0.693717979106306,1.,1.60662857109684));
#32110=CARTESIAN_POINT('Ctrl Pts',(-0.695712097881194,-1.,1.61106790958151));
#32111=CARTESIAN_POINT('Ctrl Pts',(-0.695712097881194,1.,1.61106790958151));
#32112=CARTESIAN_POINT('Ctrl Pts',(-0.699605146405088,-1.,1.61974673472612));
#32113=CARTESIAN_POINT('Ctrl Pts',(-0.699605146405088,1.,1.61974673472612));
#32114=CARTESIAN_POINT('Ctrl Pts',(-0.705159151988319,-1.,1.63216541664676));
#32115=CARTESIAN_POINT('Ctrl Pts',(-0.705159151988319,1.,1.63216541664676));
#32116=CARTESIAN_POINT('Ctrl Pts',(-0.711993139355394,-1.,1.64752408832016));
#32117=CARTESIAN_POINT('Ctrl Pts',(-0.711993139355394,1.,1.64752408832016));
#32118=CARTESIAN_POINT('Ctrl Pts',(-0.719585433804282,-1.,1.6647288055568));
#32119=CARTESIAN_POINT('Ctrl Pts',(-0.719585433804282,1.,1.6647288055568));
#32120=CARTESIAN_POINT('Ctrl Pts',(-0.726235967997433,-1.,1.67996158455503));
#32121=CARTESIAN_POINT('Ctrl Pts',(-0.726235967997433,1.,1.67996158455503));
#32122=CARTESIAN_POINT('Ctrl Pts',(-0.731963238697195,-1.,1.69326921975743));
#32123=CARTESIAN_POINT('Ctrl Pts',(-0.731963238697195,1.,1.69326921975743));
#32124=CARTESIAN_POINT('Ctrl Pts',(-0.736799665724771,-1.,1.70473309006121));
#32125=CARTESIAN_POINT('Ctrl Pts',(-0.736799665724771,1.,1.70473309006121));
#32126=CARTESIAN_POINT('Ctrl Pts',(-0.740795162032088,-1.,1.71447789751927));
#32127=CARTESIAN_POINT('Ctrl Pts',(-0.740795162032088,1.,1.71447789751927));
#32128=CARTESIAN_POINT('Ctrl Pts',(-0.744021445433764,-1.,1.7226822991693));
#32129=CARTESIAN_POINT('Ctrl Pts',(-0.744021445433764,1.,1.7226822991693));
#32130=CARTESIAN_POINT('Ctrl Pts',(-0.746574710096436,-1.,1.72958533647399));
#32131=CARTESIAN_POINT('Ctrl Pts',(-0.746574710096436,1.,1.72958533647399));
#32132=CARTESIAN_POINT('Ctrl Pts',(-0.748582462954855,-1.,1.73550351679848));
#32133=CARTESIAN_POINT('Ctrl Pts',(-0.748582462954855,1.,1.73550351679848));
#32134=CARTESIAN_POINT('Ctrl Pts',(-0.75019343597954,-1.,1.74080458266705));
#32135=CARTESIAN_POINT('Ctrl Pts',(-0.75019343597954,1.,1.74080458266705));
#32136=CARTESIAN_POINT('Ctrl Pts',(-0.751555614163629,-1.,1.74585086852298));
#32137=CARTESIAN_POINT('Ctrl Pts',(-0.751555614163629,1.,1.74585086852298));
#32138=CARTESIAN_POINT('Ctrl Pts',(-0.752797683531377,-1.,1.75095139468809));
#32139=CARTESIAN_POINT('Ctrl Pts',(-0.752797683531377,1.,1.75095139468809));
#32140=CARTESIAN_POINT('Ctrl Pts',(-0.75400925402848,-1.,1.75631083600175));
#32141=CARTESIAN_POINT('Ctrl Pts',(-0.75400925402848,1.,1.75631083600175));
#32142=CARTESIAN_POINT('Ctrl Pts',(-0.755220979975262,-1.,1.7619781724032));
#32143=CARTESIAN_POINT('Ctrl Pts',(-0.755220979975262,1.,1.7619781724032));
#32144=CARTESIAN_POINT('Ctrl Pts',(-0.756421896028403,-1.,1.76789396003141));
#32145=CARTESIAN_POINT('Ctrl Pts',(-0.756421896028403,1.,1.76789396003141));
#32146=CARTESIAN_POINT('Ctrl Pts',(-0.757578264077238,-1.,1.77394167108342));
#32147=CARTESIAN_POINT('Ctrl Pts',(-0.757578264077238,1.,1.77394167108342));
#32148=CARTESIAN_POINT('Ctrl Pts',(-0.75865062667738,-1.,1.77999411220912));
#32149=CARTESIAN_POINT('Ctrl Pts',(-0.75865062667738,1.,1.77999411220912));
#32150=CARTESIAN_POINT('Ctrl Pts',(-0.759614401109868,-1.,1.78596964884526));
#32151=CARTESIAN_POINT('Ctrl Pts',(-0.759614401109868,1.,1.78596964884526));
#32152=CARTESIAN_POINT('Ctrl Pts',(-0.760469555880425,-1.,1.79185815610802));
#32153=CARTESIAN_POINT('Ctrl Pts',(-0.760469555880425,1.,1.79185815610802));
#32154=CARTESIAN_POINT('Ctrl Pts',(-0.761229695230359,-1.,1.79768986997735));
#32155=CARTESIAN_POINT('Ctrl Pts',(-0.761229695230359,1.,1.79768986997735));
#32156=CARTESIAN_POINT('Ctrl Pts',(-0.761915336443516,-1.,1.80351583877334));
#32157=CARTESIAN_POINT('Ctrl Pts',(-0.761915336443516,1.,1.80351583877334));
#32158=CARTESIAN_POINT('Ctrl Pts',(-0.762546129464036,-1.,1.80938551463989));
#32159=CARTESIAN_POINT('Ctrl Pts',(-0.762546129464036,1.,1.80938551463989));
#32160=CARTESIAN_POINT('Ctrl Pts',(-0.763132003836783,-1.,1.81532118405566));
#32161=CARTESIAN_POINT('Ctrl Pts',(-0.763132003836783,1.,1.81532118405566));
#32162=CARTESIAN_POINT('Ctrl Pts',(-0.763673465462854,-1.,1.82131873145297));
#32163=CARTESIAN_POINT('Ctrl Pts',(-0.763673465462854,1.,1.82131873145297));
#32164=CARTESIAN_POINT('Ctrl Pts',(-0.764165902606055,-1.,1.8273599120008));
#32165=CARTESIAN_POINT('Ctrl Pts',(-0.764165902606055,1.,1.8273599120008));
#32166=CARTESIAN_POINT('Ctrl Pts',(-0.764602549687845,-1.,1.8334207722714));
#32167=CARTESIAN_POINT('Ctrl Pts',(-0.764602549687845,1.,1.8334207722714));
#32168=CARTESIAN_POINT('Ctrl Pts',(-0.764978057881687,-1.,1.83948181064823));
#32169=CARTESIAN_POINT('Ctrl Pts',(-0.764978057881687,1.,1.83948181064823));
#32170=CARTESIAN_POINT('Ctrl Pts',(-0.765291664861971,-1.,1.8455369887591));
#32171=CARTESIAN_POINT('Ctrl Pts',(-0.765291664861971,1.,1.8455369887591));
#32172=CARTESIAN_POINT('Ctrl Pts',(-0.765545710619023,-1.,1.85158945130054));
#32173=CARTESIAN_POINT('Ctrl Pts',(-0.765545710619023,1.,1.85158945130054));
#32174=CARTESIAN_POINT('Ctrl Pts',(-0.765744212909305,-1.,1.85764741390391));
#32175=CARTESIAN_POINT('Ctrl Pts',(-0.765744212909305,1.,1.85764741390391));
#32176=CARTESIAN_POINT('Ctrl Pts',(-0.765891519092557,-1.,1.86372027063314));
#32177=CARTESIAN_POINT('Ctrl Pts',(-0.765891519092557,1.,1.86372027063314));
#32178=CARTESIAN_POINT('Ctrl Pts',(-0.765990708546111,-1.,1.86981398314345));
#32179=CARTESIAN_POINT('Ctrl Pts',(-0.765990708546111,1.,1.86981398314345));
#32180=CARTESIAN_POINT('Ctrl Pts',(-0.766042837036759,-1.,1.87592888967886));
#32181=CARTESIAN_POINT('Ctrl Pts',(-0.766042837036759,1.,1.87592888967886));
#32182=CARTESIAN_POINT('Ctrl Pts',(-0.766047794851869,-1.,1.88206215302561));
#32183=CARTESIAN_POINT('Ctrl Pts',(-0.766047794851869,1.,1.88206215302561));
#32184=CARTESIAN_POINT('Ctrl Pts',(-0.76600483706209,-1.,1.88820926433409));
#32185=CARTESIAN_POINT('Ctrl Pts',(-0.76600483706209,1.,1.88820926433409));
#32186=CARTESIAN_POINT('Ctrl Pts',(-0.765913193856979,-1.,1.89436577771389));
#32187=CARTESIAN_POINT('Ctrl Pts',(-0.765913193856979,1.,1.89436577771389));
#32188=CARTESIAN_POINT('Ctrl Pts',(-0.765772772593395,-1.,1.90052930393599));
#32189=CARTESIAN_POINT('Ctrl Pts',(-0.765772772593395,1.,1.90052930393599));
#32190=CARTESIAN_POINT('Ctrl Pts',(-0.765584196937936,-1.,1.90669961402362));
#32191=CARTESIAN_POINT('Ctrl Pts',(-0.765584196937936,1.,1.90669961402362));
#32192=CARTESIAN_POINT('Ctrl Pts',(-0.765348465884739,-1.,1.91287765805174));
#32193=CARTESIAN_POINT('Ctrl Pts',(-0.765348465884739,1.,1.91287765805174));
#32194=CARTESIAN_POINT('Ctrl Pts',(-0.765066729667095,-1.,1.91906491634197));
#32195=CARTESIAN_POINT('Ctrl Pts',(-0.765066729667095,1.,1.91906491634197));
#32196=CARTESIAN_POINT('Ctrl Pts',(-0.764740025488189,-1.,1.92526263537041));
#32197=CARTESIAN_POINT('Ctrl Pts',(-0.764740025488189,1.,1.92526263537041));
#32198=CARTESIAN_POINT('Ctrl Pts',(-0.764369010673889,-1.,1.93147105496367));
#32199=CARTESIAN_POINT('Ctrl Pts',(-0.764369010673889,1.,1.93147105496367));
#32200=CARTESIAN_POINT('Ctrl Pts',(-0.763954049121393,-1.,1.93768964875867));
#32201=CARTESIAN_POINT('Ctrl Pts',(-0.763954049121393,1.,1.93768964875867));
#32202=CARTESIAN_POINT('Ctrl Pts',(-0.76349533353858,-1.,1.94391746617626));
#32203=CARTESIAN_POINT('Ctrl Pts',(-0.76349533353858,1.,1.94391746617626));
#32204=CARTESIAN_POINT('Ctrl Pts',(-0.762992990878774,-1.,1.95015342590025));
#32205=CARTESIAN_POINT('Ctrl Pts',(-0.762992990878774,1.,1.95015342590025));
#32206=CARTESIAN_POINT('Ctrl Pts',(-0.762447203806263,-1.,1.95639665309893));
#32207=CARTESIAN_POINT('Ctrl Pts',(-0.762447203806263,1.,1.95639665309893));
#32208=CARTESIAN_POINT('Ctrl Pts',(-0.761858300014575,-1.,1.96264672744229));
#32209=CARTESIAN_POINT('Ctrl Pts',(-0.761858300014575,1.,1.96264672744229));
#32210=CARTESIAN_POINT('Ctrl Pts',(-0.761226690483986,-1.,1.96890351582545));
#32211=CARTESIAN_POINT('Ctrl Pts',(-0.761226690483986,1.,1.96890351582545));
#32212=CARTESIAN_POINT('Ctrl Pts',(-0.760552825409855,-1.,1.97516705321521));
#32213=CARTESIAN_POINT('Ctrl Pts',(-0.760552825409855,1.,1.97516705321521));
#32214=CARTESIAN_POINT('Ctrl Pts',(-0.759837147452135,-1.,1.98143741418156));
#32215=CARTESIAN_POINT('Ctrl Pts',(-0.759837147452135,1.,1.98143741418156));
#32216=CARTESIAN_POINT('Ctrl Pts',(-0.759080037802243,-1.,1.98771456680806));
#32217=CARTESIAN_POINT('Ctrl Pts',(-0.759080037802243,1.,1.98771456680806));
#32218=CARTESIAN_POINT('Ctrl Pts',(-0.758281796766377,-1.,1.9939983109871));
#32219=CARTESIAN_POINT('Ctrl Pts',(-0.758281796766377,1.,1.9939983109871));
#32220=CARTESIAN_POINT('Ctrl Pts',(-0.757442676862341,-1.,2.00028834739072));
#32221=CARTESIAN_POINT('Ctrl Pts',(-0.757442676862341,1.,2.00028834739072));
#32222=CARTESIAN_POINT('Ctrl Pts',(-0.756562904646496,-1.,2.00658431587682));
#32223=CARTESIAN_POINT('Ctrl Pts',(-0.756562904646496,1.,2.00658431587682));
#32224=CARTESIAN_POINT('Ctrl Pts',(-0.7556427049581,-1.,2.01288584328149));
#32225=CARTESIAN_POINT('Ctrl Pts',(-0.7556427049581,1.,2.01288584328149));
#32226=CARTESIAN_POINT('Ctrl Pts',(-0.75468233072352,-1.,2.01919259406003));
#32227=CARTESIAN_POINT('Ctrl Pts',(-0.75468233072352,1.,2.01919259406003));
#32228=CARTESIAN_POINT('Ctrl Pts',(-0.753682061113766,-1.,2.02550428623587));
#32229=CARTESIAN_POINT('Ctrl Pts',(-0.753682061113766,1.,2.02550428623587));
#32230=CARTESIAN_POINT('Ctrl Pts',(-0.752642180488104,-1.,2.03182068456467));
#32231=CARTESIAN_POINT('Ctrl Pts',(-0.752642180488104,1.,2.03182068456467));
#32232=CARTESIAN_POINT('Ctrl Pts',(-0.751562963361384,-1.,2.03814160092173));
#32233=CARTESIAN_POINT('Ctrl Pts',(-0.751562963361384,1.,2.03814160092173));
#32234=CARTESIAN_POINT('Ctrl Pts',(-0.750444657874758,-1.,2.04446689147754));
#32235=CARTESIAN_POINT('Ctrl Pts',(-0.750444657874758,1.,2.04446689147754));
#32236=CARTESIAN_POINT('Ctrl Pts',(-0.749287468663053,-1.,2.05079645591606));
#32237=CARTESIAN_POINT('Ctrl Pts',(-0.749287468663053,1.,2.05079645591606));
#32238=CARTESIAN_POINT('Ctrl Pts',(-0.748091554181101,-1.,2.05713023030263));
#32239=CARTESIAN_POINT('Ctrl Pts',(-0.748091554181101,1.,2.05713023030263));
#32240=CARTESIAN_POINT('Ctrl Pts',(-0.747103932785504,-1.,2.06220058927162));
#32241=CARTESIAN_POINT('Ctrl Pts',(-0.747103932785504,1.,2.06220058927162));
#32242=CARTESIAN_POINT('Ctrl Pts',(-0.746345871542696,-1.,2.06600523016401));
#32243=CARTESIAN_POINT('Ctrl Pts',(-0.746345871542696,1.,2.06600523016401));
#32244=CARTESIAN_POINT('Ctrl Pts',(-0.74583279137781,-1.,2.06854248895575));
#32245=CARTESIAN_POINT('Ctrl Pts',(-0.74583279137781,1.,2.06854248895575));
#32246=CARTESIAN_POINT('Ctrl Pts',(-0.745574324794401,-1.,2.0698113262342));
#32247=CARTESIAN_POINT('Ctrl Pts',(-0.745574324794401,1.,2.0698113262342));
#32248=CARTESIAN_POINT('',(-0.693717979106306,1.,1.60662857109684));
#32249=CARTESIAN_POINT('Ctrl Pts',(-0.693717979106306,1.,1.60662857109684));
#32250=CARTESIAN_POINT('Ctrl Pts',(-0.695712097881194,1.,1.61106790958151));
#32251=CARTESIAN_POINT('Ctrl Pts',(-0.699605146405088,1.,1.61974673472612));
#32252=CARTESIAN_POINT('Ctrl Pts',(-0.705159151988319,1.,1.63216541664676));
#32253=CARTESIAN_POINT('Ctrl Pts',(-0.711993139355394,1.,1.64752408832016));
#32254=CARTESIAN_POINT('Ctrl Pts',(-0.719585433804282,1.,1.6647288055568));
#32255=CARTESIAN_POINT('Ctrl Pts',(-0.726235967997433,1.,1.67996158455503));
#32256=CARTESIAN_POINT('Ctrl Pts',(-0.731963238697195,1.,1.69326921975743));
#32257=CARTESIAN_POINT('Ctrl Pts',(-0.736799665724771,1.,1.70473309006121));
#32258=CARTESIAN_POINT('Ctrl Pts',(-0.740795162032088,1.,1.71447789751927));
#32259=CARTESIAN_POINT('Ctrl Pts',(-0.744021445433764,1.,1.7226822991693));
#32260=CARTESIAN_POINT('Ctrl Pts',(-0.746574710096436,1.,1.72958533647399));
#32261=CARTESIAN_POINT('Ctrl Pts',(-0.748582462954855,1.,1.73550351679848));
#32262=CARTESIAN_POINT('Ctrl Pts',(-0.75019343597954,1.,1.74080458266705));
#32263=CARTESIAN_POINT('Ctrl Pts',(-0.751555614163629,1.,1.74585086852298));
#32264=CARTESIAN_POINT('Ctrl Pts',(-0.752797683531377,1.,1.75095139468809));
#32265=CARTESIAN_POINT('Ctrl Pts',(-0.75400925402848,1.,1.75631083600175));
#32266=CARTESIAN_POINT('Ctrl Pts',(-0.755220979975262,1.,1.7619781724032));
#32267=CARTESIAN_POINT('Ctrl Pts',(-0.756421896028403,1.,1.76789396003141));
#32268=CARTESIAN_POINT('Ctrl Pts',(-0.757578264077238,1.,1.77394167108342));
#32269=CARTESIAN_POINT('Ctrl Pts',(-0.75865062667738,1.,1.77999411220912));
#32270=CARTESIAN_POINT('Ctrl Pts',(-0.759614401109868,1.,1.78596964884526));
#32271=CARTESIAN_POINT('Ctrl Pts',(-0.760469555880425,1.,1.79185815610802));
#32272=CARTESIAN_POINT('Ctrl Pts',(-0.761229695230359,1.,1.79768986997735));
#32273=CARTESIAN_POINT('Ctrl Pts',(-0.761915336443516,1.,1.80351583877334));
#32274=CARTESIAN_POINT('Ctrl Pts',(-0.762546129464036,1.,1.80938551463989));
#32275=CARTESIAN_POINT('Ctrl Pts',(-0.763132003836783,1.,1.81532118405566));
#32276=CARTESIAN_POINT('Ctrl Pts',(-0.763673465462854,1.,1.82131873145297));
#32277=CARTESIAN_POINT('Ctrl Pts',(-0.764165902606055,1.,1.8273599120008));
#32278=CARTESIAN_POINT('Ctrl Pts',(-0.764602549687845,1.,1.8334207722714));
#32279=CARTESIAN_POINT('Ctrl Pts',(-0.764978057881687,1.,1.83948181064823));
#32280=CARTESIAN_POINT('Ctrl Pts',(-0.765291664861971,1.,1.8455369887591));
#32281=CARTESIAN_POINT('Ctrl Pts',(-0.765545710619023,1.,1.85158945130054));
#32282=CARTESIAN_POINT('Ctrl Pts',(-0.765744212909305,1.,1.85764741390391));
#32283=CARTESIAN_POINT('Ctrl Pts',(-0.765891519092557,1.,1.86372027063314));
#32284=CARTESIAN_POINT('Ctrl Pts',(-0.765990708546111,1.,1.86981398314345));
#32285=CARTESIAN_POINT('Ctrl Pts',(-0.766042837036759,1.,1.87592888967886));
#32286=CARTESIAN_POINT('Ctrl Pts',(-0.766047794851869,1.,1.88206215302561));
#32287=CARTESIAN_POINT('Ctrl Pts',(-0.76600483706209,1.,1.88820926433409));
#32288=CARTESIAN_POINT('Ctrl Pts',(-0.765913193856979,1.,1.89436577771389));
#32289=CARTESIAN_POINT('Ctrl Pts',(-0.765772772593395,1.,1.90052930393599));
#32290=CARTESIAN_POINT('Ctrl Pts',(-0.765584196937936,1.,1.90669961402362));
#32291=CARTESIAN_POINT('Ctrl Pts',(-0.765348465884739,1.,1.91287765805174));
#32292=CARTESIAN_POINT('Ctrl Pts',(-0.765066729667095,1.,1.91906491634197));
#32293=CARTESIAN_POINT('Ctrl Pts',(-0.764740025488189,1.,1.92526263537041));
#32294=CARTESIAN_POINT('Ctrl Pts',(-0.764369010673889,1.,1.93147105496367));
#32295=CARTESIAN_POINT('Ctrl Pts',(-0.763954049121393,1.,1.93768964875867));
#32296=CARTESIAN_POINT('Ctrl Pts',(-0.76349533353858,1.,1.94391746617626));
#32297=CARTESIAN_POINT('Ctrl Pts',(-0.762992990878774,1.,1.95015342590025));
#32298=CARTESIAN_POINT('Ctrl Pts',(-0.762447203806263,1.,1.95639665309893));
#32299=CARTESIAN_POINT('Ctrl Pts',(-0.761858300014575,1.,1.96264672744229));
#32300=CARTESIAN_POINT('Ctrl Pts',(-0.761226690483986,1.,1.96890351582545));
#32301=CARTESIAN_POINT('Ctrl Pts',(-0.760552825409855,1.,1.97516705321521));
#32302=CARTESIAN_POINT('Ctrl Pts',(-0.759837147452135,1.,1.98143741418156));
#32303=CARTESIAN_POINT('Ctrl Pts',(-0.759080037802243,1.,1.98771456680806));
#32304=CARTESIAN_POINT('Ctrl Pts',(-0.758281796766377,1.,1.9939983109871));
#32305=CARTESIAN_POINT('Ctrl Pts',(-0.757442676862341,1.,2.00028834739072));
#32306=CARTESIAN_POINT('Ctrl Pts',(-0.756562904646496,1.,2.00658431587682));
#32307=CARTESIAN_POINT('Ctrl Pts',(-0.7556427049581,1.,2.01288584328149));
#32308=CARTESIAN_POINT('Ctrl Pts',(-0.75468233072352,1.,2.01919259406003));
#32309=CARTESIAN_POINT('Ctrl Pts',(-0.753682061113766,1.,2.02550428623587));
#32310=CARTESIAN_POINT('Ctrl Pts',(-0.752642180488104,1.,2.03182068456467));
#32311=CARTESIAN_POINT('Ctrl Pts',(-0.751562963361384,1.,2.03814160092173));
#32312=CARTESIAN_POINT('Ctrl Pts',(-0.750444657874758,1.,2.04446689147754));
#32313=CARTESIAN_POINT('Ctrl Pts',(-0.749287468663053,1.,2.05079645591606));
#32314=CARTESIAN_POINT('Ctrl Pts',(-0.748091554181101,1.,2.05713023030263));
#32315=CARTESIAN_POINT('Ctrl Pts',(-0.747103932785504,1.,2.06220058927162));
#32316=CARTESIAN_POINT('Ctrl Pts',(-0.746345871542696,1.,2.06600523016401));
#32317=CARTESIAN_POINT('Ctrl Pts',(-0.74583279137781,1.,2.06854248895575));
#32318=CARTESIAN_POINT('Ctrl Pts',(-0.745574324794401,1.,2.0698113262342));
#32319=CARTESIAN_POINT('',(-0.693717979106306,0.,1.60662857109684));
#32320=CARTESIAN_POINT('Origin',(0.,0.,0.));
#32321=CARTESIAN_POINT('',(-0.892032620296855,1.,1.5055822144029));
#32322=CARTESIAN_POINT('Origin',(0.,1.,0.));
#32323=CARTESIAN_POINT('',(-0.892032620296855,0.,1.5055822144029));
#32324=CARTESIAN_POINT('Ctrl Pts',(-1.23627494547115,-1.,1.81978687191668));
#32325=CARTESIAN_POINT('Ctrl Pts',(-1.23627494547115,1.,1.81978687191668));
#32326=CARTESIAN_POINT('Ctrl Pts',(-1.23509651170476,-1.,1.81925017193666));
#32327=CARTESIAN_POINT('Ctrl Pts',(-1.23509651170476,1.,1.81925017193666));
#32328=CARTESIAN_POINT('Ctrl Pts',(-1.2327422452705,-1.,1.81817389921279));
#32329=CARTESIAN_POINT('Ctrl Pts',(-1.2327422452705,1.,1.81817389921279));
#32330=CARTESIAN_POINT('Ctrl Pts',(-1.2292186489137,-1.,1.8165508718364));
#32331=CARTESIAN_POINT('Ctrl Pts',(-1.2292186489137,1.,1.8165508718364));
#32332=CARTESIAN_POINT('Ctrl Pts',(-1.2245361330495,-1.,1.81436959210434));
#32333=CARTESIAN_POINT('Ctrl Pts',(-1.2245361330495,1.,1.81436959210434));
#32334=CARTESIAN_POINT('Ctrl Pts',(-1.21870906103557,-1.,1.81161420806656));
#32335=CARTESIAN_POINT('Ctrl Pts',(-1.21870906103557,1.,1.81161420806656));
#32336=CARTESIAN_POINT('Ctrl Pts',(-1.21290815708314,-1.,1.80882996917129));
#32337=CARTESIAN_POINT('Ctrl Pts',(-1.21290815708314,1.,1.80882996917129));
#32338=CARTESIAN_POINT('Ctrl Pts',(-1.20713356605475,-1.,1.80601678480707));
#32339=CARTESIAN_POINT('Ctrl Pts',(-1.20713356605475,1.,1.80601678480707));
#32340=CARTESIAN_POINT('Ctrl Pts',(-1.20138548938974,-1.,1.80317454838603));
#32341=CARTESIAN_POINT('Ctrl Pts',(-1.20138548938974,1.,1.80317454838603));
#32342=CARTESIAN_POINT('Ctrl Pts',(-1.19566418930242,-1.,1.80030314369879));
#32343=CARTESIAN_POINT('Ctrl Pts',(-1.19566418930242,1.,1.80030314369879));
#32344=CARTESIAN_POINT('Ctrl Pts',(-1.18996997934445,-1.,1.79740245923478));
#32345=CARTESIAN_POINT('Ctrl Pts',(-1.18996997934445,1.,1.79740245923478));
#32346=CARTESIAN_POINT('Ctrl Pts',(-1.18430321697432,-1.,1.79447240321515));
#32347=CARTESIAN_POINT('Ctrl Pts',(-1.18430321697432,1.,1.79447240321515));
#32348=CARTESIAN_POINT('Ctrl Pts',(-1.17866429440809,-1.,1.79151291552689));
#32349=CARTESIAN_POINT('Ctrl Pts',(-1.17866429440809,1.,1.79151291552689));
#32350=CARTESIAN_POINT('Ctrl Pts',(-1.17305363177328,-1.,1.78852398877616));
#32351=CARTESIAN_POINT('Ctrl Pts',(-1.17305363177328,1.,1.78852398877616));
#32352=CARTESIAN_POINT('Ctrl Pts',(-1.16747166312303,-1.,1.78550566040443));
#32353=CARTESIAN_POINT('Ctrl Pts',(-1.16747166312303,1.,1.78550566040443));
#32354=CARTESIAN_POINT('Ctrl Pts',(-1.16191881298499,-1.,1.78245795881009));
#32355=CARTESIAN_POINT('Ctrl Pts',(-1.16191881298499,1.,1.78245795881009));
#32356=CARTESIAN_POINT('Ctrl Pts',(-1.15639547194698,-1.,1.77938085564275));
#32357=CARTESIAN_POINT('Ctrl Pts',(-1.15639547194698,1.,1.77938085564275));
#32358=CARTESIAN_POINT('Ctrl Pts',(-1.15090197841515,-1.,1.7762742255701));
#32359=CARTESIAN_POINT('Ctrl Pts',(-1.15090197841515,1.,1.7762742255701));
#32360=CARTESIAN_POINT('Ctrl Pts',(-1.1454385822692,-1.,1.77313777896194));
#32361=CARTESIAN_POINT('Ctrl Pts',(-1.1454385822692,1.,1.77313777896194));
#32362=CARTESIAN_POINT('Ctrl Pts',(-1.14000548336975,-1.,1.76997111386769));
#32363=CARTESIAN_POINT('Ctrl Pts',(-1.14000548336975,1.,1.76997111386769));
#32364=CARTESIAN_POINT('Ctrl Pts',(-1.1346029180462,-1.,1.76677384551862));
#32365=CARTESIAN_POINT('Ctrl Pts',(-1.1346029180462,1.,1.76677384551862));
#32366=CARTESIAN_POINT('Ctrl Pts',(-1.12923123555075,-1.,1.7635457196617));
#32367=CARTESIAN_POINT('Ctrl Pts',(-1.12923123555075,1.,1.7635457196617));
#32368=CARTESIAN_POINT('Ctrl Pts',(-1.12389096855086,-1.,1.76028671825096));
#32369=CARTESIAN_POINT('Ctrl Pts',(-1.12389096855086,1.,1.76028671825096));
#32370=CARTESIAN_POINT('Ctrl Pts',(-1.11858293216763,-1.,1.75699720772105));
#32371=CARTESIAN_POINT('Ctrl Pts',(-1.11858293216763,1.,1.75699720772105));
#32372=CARTESIAN_POINT('Ctrl Pts',(-1.11330807582551,-1.,1.7536777209463));
#32373=CARTESIAN_POINT('Ctrl Pts',(-1.11330807582551,1.,1.7536777209463));
#32374=CARTESIAN_POINT('Ctrl Pts',(-1.10806728183007,-1.,1.7503286607592));
#32375=CARTESIAN_POINT('Ctrl Pts',(-1.10806728183007,1.,1.7503286607592));
#32376=CARTESIAN_POINT('Ctrl Pts',(-1.10286118991143,-1.,1.74695004214923));
#32377=CARTESIAN_POINT('Ctrl Pts',(-1.10286118991143,1.,1.74695004214923));
#32378=CARTESIAN_POINT('Ctrl Pts',(-1.09768999241225,-1.,1.74354119236208));
#32379=CARTESIAN_POINT('Ctrl Pts',(-1.09768999241225,1.,1.74354119236208));
#32380=CARTESIAN_POINT('Ctrl Pts',(-1.09255329056493,-1.,1.74010053962247));
#32381=CARTESIAN_POINT('Ctrl Pts',(-1.09255329056493,1.,1.74010053962247));
#32382=CARTESIAN_POINT('Ctrl Pts',(-1.08745056285427,-1.,1.73662628326091));
#32383=CARTESIAN_POINT('Ctrl Pts',(-1.08745056285427,1.,1.73662628326091));
#32384=CARTESIAN_POINT('Ctrl Pts',(-1.08238162784749,-1.,1.73311705663407));
#32385=CARTESIAN_POINT('Ctrl Pts',(-1.08238162784749,1.,1.73311705663407));
#32386=CARTESIAN_POINT('Ctrl Pts',(-1.0773470373727,-1.,1.72957248977424));
#32387=CARTESIAN_POINT('Ctrl Pts',(-1.0773470373727,1.,1.72957248977424));
#32388=CARTESIAN_POINT('Ctrl Pts',(-1.07234866990252,-1.,1.72599406198488));
#32389=CARTESIAN_POINT('Ctrl Pts',(-1.07234866990252,1.,1.72599406198488));
#32390=CARTESIAN_POINT('Ctrl Pts',(-1.06738966975462,-1.,1.72238500928453));
#32391=CARTESIAN_POINT('Ctrl Pts',(-1.06738966975462,1.,1.72238500928453));
#32392=CARTESIAN_POINT('Ctrl Pts',(-1.06247324680647,-1.,1.71874858456904));
#32393=CARTESIAN_POINT('Ctrl Pts',(-1.06247324680647,1.,1.71874858456904));
#32394=CARTESIAN_POINT('Ctrl Pts',(-1.05760163192479,-1.,1.7150865442702));
#32395=CARTESIAN_POINT('Ctrl Pts',(-1.05760163192479,1.,1.7150865442702));
#32396=CARTESIAN_POINT('Ctrl Pts',(-1.05277517202855,-1.,1.71139783543989));
#32397=CARTESIAN_POINT('Ctrl Pts',(-1.05277517202855,1.,1.71139783543989));
#32398=CARTESIAN_POINT('Ctrl Pts',(-1.04799085404995,-1.,1.70767646263649));
#32399=CARTESIAN_POINT('Ctrl Pts',(-1.04799085404995,1.,1.70767646263649));
#32400=CARTESIAN_POINT('Ctrl Pts',(-1.04324363334554,-1.,1.70391338707982));
#32401=CARTESIAN_POINT('Ctrl Pts',(-1.04324363334554,1.,1.70391338707982));
#32402=CARTESIAN_POINT('Ctrl Pts',(-1.03852922490789,-1.,1.70010052930962));
#32403=CARTESIAN_POINT('Ctrl Pts',(-1.03852922490789,1.,1.70010052930962));
#32404=CARTESIAN_POINT('Ctrl Pts',(-1.03384646003588,-1.,1.69623414782771));
#32405=CARTESIAN_POINT('Ctrl Pts',(-1.03384646003588,1.,1.69623414782771));
#32406=CARTESIAN_POINT('Ctrl Pts',(-1.02919977579147,-1.,1.69231840863458));
#32407=CARTESIAN_POINT('Ctrl Pts',(-1.02919977579147,1.,1.69231840863458));
#32408=CARTESIAN_POINT('Ctrl Pts',(-1.02460180535255,-1.,1.68836910178447));
#32409=CARTESIAN_POINT('Ctrl Pts',(-1.02460180535255,1.,1.68836910178447));
#32410=CARTESIAN_POINT('Ctrl Pts',(-1.02006795074201,-1.,1.68440578021706));
#32411=CARTESIAN_POINT('Ctrl Pts',(-1.02006795074201,1.,1.68440578021706));
#32412=CARTESIAN_POINT('Ctrl Pts',(-1.01561026162773,-1.,1.68044289894798));
#32413=CARTESIAN_POINT('Ctrl Pts',(-1.01561026162773,1.,1.68044289894798));
#32414=CARTESIAN_POINT('Ctrl Pts',(-1.01123236493511,-1.,1.67648246776464));
#32415=CARTESIAN_POINT('Ctrl Pts',(-1.01123236493511,1.,1.67648246776464));
#32416=CARTESIAN_POINT('Ctrl Pts',(-1.00692206696414,-1.,1.67250335383293));
#32417=CARTESIAN_POINT('Ctrl Pts',(-1.00692206696414,1.,1.67250335383293));
#32418=CARTESIAN_POINT('Ctrl Pts',(-1.00265091003727,-1.,1.66846059277303));
#32419=CARTESIAN_POINT('Ctrl Pts',(-1.00265091003727,1.,1.66846059277303));
#32420=CARTESIAN_POINT('Ctrl Pts',(-0.998389654952758,-1.,1.66430758030376));
#32421=CARTESIAN_POINT('Ctrl Pts',(-0.998389654952758,1.,1.66430758030376));
#32422=CARTESIAN_POINT('Ctrl Pts',(-0.994121836661306,-1.,1.66001553809947));
#32423=CARTESIAN_POINT('Ctrl Pts',(-0.994121836661306,1.,1.66001553809947));
#32424=CARTESIAN_POINT('Ctrl Pts',(-0.989855627854165,-1.,1.65559044289699));
#32425=CARTESIAN_POINT('Ctrl Pts',(-0.989855627854165,1.,1.65559044289699));
#32426=CARTESIAN_POINT('Ctrl Pts',(-0.985642622920821,-1.,1.65110016612638));
#32427=CARTESIAN_POINT('Ctrl Pts',(-0.985642622920821,1.,1.65110016612638));
#32428=CARTESIAN_POINT('Ctrl Pts',(-0.981562530939489,-1.,1.64665139190656));
#32429=CARTESIAN_POINT('Ctrl Pts',(-0.981562530939489,1.,1.64665139190656));
#32430=CARTESIAN_POINT('Ctrl Pts',(-0.977689794119416,-1.,1.64233990826687));
#32431=CARTESIAN_POINT('Ctrl Pts',(-0.977689794119416,1.,1.64233990826687));
#32432=CARTESIAN_POINT('Ctrl Pts',(-0.974066058287418,-1.,1.63820952658144));
#32433=CARTESIAN_POINT('Ctrl Pts',(-0.974066058287418,1.,1.63820952658144));
#32434=CARTESIAN_POINT('Ctrl Pts',(-0.970669715997509,-1.,1.63420665729798));
#32435=CARTESIAN_POINT('Ctrl Pts',(-0.970669715997509,1.,1.63420665729798));
#32436=CARTESIAN_POINT('Ctrl Pts',(-0.967387853230345,-1.,1.63013849959461));
#32437=CARTESIAN_POINT('Ctrl Pts',(-0.967387853230345,1.,1.63013849959461));
#32438=CARTESIAN_POINT('Ctrl Pts',(-0.964046107040536,-1.,1.62571930670187));
#32439=CARTESIAN_POINT('Ctrl Pts',(-0.964046107040536,1.,1.62571930670187));
#32440=CARTESIAN_POINT('Ctrl Pts',(-0.960438326101729,-1.,1.62061638140221));
#32441=CARTESIAN_POINT('Ctrl Pts',(-0.960438326101729,1.,1.62061638140221));
#32442=CARTESIAN_POINT('Ctrl Pts',(-0.956354422920671,-1.,1.61449324337085));
#32443=CARTESIAN_POINT('Ctrl Pts',(-0.956354422920671,1.,1.61449324337085));
#32444=CARTESIAN_POINT('Ctrl Pts',(-0.951613284356035,-1.,1.60706069896936));
#32445=CARTESIAN_POINT('Ctrl Pts',(-0.951613284356035,1.,1.60706069896936));
#32446=CARTESIAN_POINT('Ctrl Pts',(-0.946078063315257,-1.,1.59810042043673));
#32447=CARTESIAN_POINT('Ctrl Pts',(-0.946078063315257,1.,1.59810042043673));
#32448=CARTESIAN_POINT('Ctrl Pts',(-0.939646377893399,-1.,1.58744937487176));
#32449=CARTESIAN_POINT('Ctrl Pts',(-0.939646377893399,1.,1.58744937487176));
#32450=CARTESIAN_POINT('Ctrl Pts',(-0.932246680108685,-1.,1.57499388382243));
#32451=CARTESIAN_POINT('Ctrl Pts',(-0.932246680108685,1.,1.57499388382243));
#32452=CARTESIAN_POINT('Ctrl Pts',(-0.923832188944341,-1.,1.56065988578893));
#32453=CARTESIAN_POINT('Ctrl Pts',(-0.923832188944341,1.,1.56065988578893));
#32454=CARTESIAN_POINT('Ctrl Pts',(-0.914375919026456,-1.,1.54440491149498));
#32455=CARTESIAN_POINT('Ctrl Pts',(-0.914375919026456,1.,1.54440491149498));
#32456=CARTESIAN_POINT('Ctrl Pts',(-0.905967409625651,-1.,1.52984849887993));
#32457=CARTESIAN_POINT('Ctrl Pts',(-0.905967409625651,1.,1.52984849887993));
#32458=CARTESIAN_POINT('Ctrl Pts',(-0.899185047483511,-1.,1.51805569590094));
#32459=CARTESIAN_POINT('Ctrl Pts',(-0.899185047483511,1.,1.51805569590094));
#32460=CARTESIAN_POINT('Ctrl Pts',(-0.894452006964543,-1.,1.50980486806688));
#32461=CARTESIAN_POINT('Ctrl Pts',(-0.894452006964543,1.,1.50980486806688));
#32462=CARTESIAN_POINT('Ctrl Pts',(-0.892032620296855,-1.,1.5055822144029));
#32463=CARTESIAN_POINT('Ctrl Pts',(-0.892032620296855,1.,1.5055822144029));
#32464=CARTESIAN_POINT('',(-1.23627494547115,1.,1.81978687191668));
#32465=CARTESIAN_POINT('Ctrl Pts',(-1.23627494547115,1.,1.81978687191668));
#32466=CARTESIAN_POINT('Ctrl Pts',(-1.23509651170476,1.,1.81925017193666));
#32467=CARTESIAN_POINT('Ctrl Pts',(-1.2327422452705,1.,1.81817389921279));
#32468=CARTESIAN_POINT('Ctrl Pts',(-1.2292186489137,1.,1.8165508718364));
#32469=CARTESIAN_POINT('Ctrl Pts',(-1.2245361330495,1.,1.81436959210434));
#32470=CARTESIAN_POINT('Ctrl Pts',(-1.21870906103557,1.,1.81161420806656));
#32471=CARTESIAN_POINT('Ctrl Pts',(-1.21290815708314,1.,1.80882996917129));
#32472=CARTESIAN_POINT('Ctrl Pts',(-1.20713356605475,1.,1.80601678480707));
#32473=CARTESIAN_POINT('Ctrl Pts',(-1.20138548938974,1.,1.80317454838603));
#32474=CARTESIAN_POINT('Ctrl Pts',(-1.19566418930242,1.,1.80030314369879));
#32475=CARTESIAN_POINT('Ctrl Pts',(-1.18996997934445,1.,1.79740245923478));
#32476=CARTESIAN_POINT('Ctrl Pts',(-1.18430321697432,1.,1.79447240321515));
#32477=CARTESIAN_POINT('Ctrl Pts',(-1.17866429440809,1.,1.79151291552689));
#32478=CARTESIAN_POINT('Ctrl Pts',(-1.17305363177328,1.,1.78852398877616));
#32479=CARTESIAN_POINT('Ctrl Pts',(-1.16747166312303,1.,1.78550566040443));
#32480=CARTESIAN_POINT('Ctrl Pts',(-1.16191881298499,1.,1.78245795881009));
#32481=CARTESIAN_POINT('Ctrl Pts',(-1.15639547194698,1.,1.77938085564275));
#32482=CARTESIAN_POINT('Ctrl Pts',(-1.15090197841515,1.,1.7762742255701));
#32483=CARTESIAN_POINT('Ctrl Pts',(-1.1454385822692,1.,1.77313777896194));
#32484=CARTESIAN_POINT('Ctrl Pts',(-1.14000548336975,1.,1.76997111386769));
#32485=CARTESIAN_POINT('Ctrl Pts',(-1.1346029180462,1.,1.76677384551862));
#32486=CARTESIAN_POINT('Ctrl Pts',(-1.12923123555075,1.,1.7635457196617));
#32487=CARTESIAN_POINT('Ctrl Pts',(-1.12389096855086,1.,1.76028671825096));
#32488=CARTESIAN_POINT('Ctrl Pts',(-1.11858293216763,1.,1.75699720772105));
#32489=CARTESIAN_POINT('Ctrl Pts',(-1.11330807582551,1.,1.7536777209463));
#32490=CARTESIAN_POINT('Ctrl Pts',(-1.10806728183007,1.,1.7503286607592));
#32491=CARTESIAN_POINT('Ctrl Pts',(-1.10286118991143,1.,1.74695004214923));
#32492=CARTESIAN_POINT('Ctrl Pts',(-1.09768999241225,1.,1.74354119236208));
#32493=CARTESIAN_POINT('Ctrl Pts',(-1.09255329056493,1.,1.74010053962247));
#32494=CARTESIAN_POINT('Ctrl Pts',(-1.08745056285427,1.,1.73662628326091));
#32495=CARTESIAN_POINT('Ctrl Pts',(-1.08238162784749,1.,1.73311705663407));
#32496=CARTESIAN_POINT('Ctrl Pts',(-1.0773470373727,1.,1.72957248977424));
#32497=CARTESIAN_POINT('Ctrl Pts',(-1.07234866990252,1.,1.72599406198488));
#32498=CARTESIAN_POINT('Ctrl Pts',(-1.06738966975462,1.,1.72238500928453));
#32499=CARTESIAN_POINT('Ctrl Pts',(-1.06247324680647,1.,1.71874858456904));
#32500=CARTESIAN_POINT('Ctrl Pts',(-1.05760163192479,1.,1.7150865442702));
#32501=CARTESIAN_POINT('Ctrl Pts',(-1.05277517202855,1.,1.71139783543989));
#32502=CARTESIAN_POINT('Ctrl Pts',(-1.04799085404995,1.,1.70767646263649));
#32503=CARTESIAN_POINT('Ctrl Pts',(-1.04324363334554,1.,1.70391338707982));
#32504=CARTESIAN_POINT('Ctrl Pts',(-1.03852922490789,1.,1.70010052930962));
#32505=CARTESIAN_POINT('Ctrl Pts',(-1.03384646003588,1.,1.69623414782771));
#32506=CARTESIAN_POINT('Ctrl Pts',(-1.02919977579147,1.,1.69231840863458));
#32507=CARTESIAN_POINT('Ctrl Pts',(-1.02460180535255,1.,1.68836910178447));
#32508=CARTESIAN_POINT('Ctrl Pts',(-1.02006795074201,1.,1.68440578021706));
#32509=CARTESIAN_POINT('Ctrl Pts',(-1.01561026162773,1.,1.68044289894798));
#32510=CARTESIAN_POINT('Ctrl Pts',(-1.01123236493511,1.,1.67648246776464));
#32511=CARTESIAN_POINT('Ctrl Pts',(-1.00692206696414,1.,1.67250335383293));
#32512=CARTESIAN_POINT('Ctrl Pts',(-1.00265091003727,1.,1.66846059277303));
#32513=CARTESIAN_POINT('Ctrl Pts',(-0.998389654952758,1.,1.66430758030376));
#32514=CARTESIAN_POINT('Ctrl Pts',(-0.994121836661306,1.,1.66001553809947));
#32515=CARTESIAN_POINT('Ctrl Pts',(-0.989855627854165,1.,1.65559044289699));
#32516=CARTESIAN_POINT('Ctrl Pts',(-0.985642622920821,1.,1.65110016612638));
#32517=CARTESIAN_POINT('Ctrl Pts',(-0.981562530939489,1.,1.64665139190656));
#32518=CARTESIAN_POINT('Ctrl Pts',(-0.977689794119416,1.,1.64233990826687));
#32519=CARTESIAN_POINT('Ctrl Pts',(-0.974066058287418,1.,1.63820952658144));
#32520=CARTESIAN_POINT('Ctrl Pts',(-0.970669715997509,1.,1.63420665729798));
#32521=CARTESIAN_POINT('Ctrl Pts',(-0.967387853230345,1.,1.63013849959461));
#32522=CARTESIAN_POINT('Ctrl Pts',(-0.964046107040536,1.,1.62571930670187));
#32523=CARTESIAN_POINT('Ctrl Pts',(-0.960438326101729,1.,1.62061638140221));
#32524=CARTESIAN_POINT('Ctrl Pts',(-0.956354422920671,1.,1.61449324337085));
#32525=CARTESIAN_POINT('Ctrl Pts',(-0.951613284356035,1.,1.60706069896936));
#32526=CARTESIAN_POINT('Ctrl Pts',(-0.946078063315257,1.,1.59810042043673));
#32527=CARTESIAN_POINT('Ctrl Pts',(-0.939646377893399,1.,1.58744937487176));
#32528=CARTESIAN_POINT('Ctrl Pts',(-0.932246680108685,1.,1.57499388382243));
#32529=CARTESIAN_POINT('Ctrl Pts',(-0.923832188944341,1.,1.56065988578893));
#32530=CARTESIAN_POINT('Ctrl Pts',(-0.914375919026456,1.,1.54440491149498));
#32531=CARTESIAN_POINT('Ctrl Pts',(-0.905967409625651,1.,1.52984849887993));
#32532=CARTESIAN_POINT('Ctrl Pts',(-0.899185047483511,1.,1.51805569590094));
#32533=CARTESIAN_POINT('Ctrl Pts',(-0.894452006964543,1.,1.50980486806688));
#32534=CARTESIAN_POINT('Ctrl Pts',(-0.892032620296855,1.,1.5055822144029));
#32535=CARTESIAN_POINT('',(-1.23627494547115,0.,1.81978687191668));
#32536=CARTESIAN_POINT('Origin',(-1.34869019493419,0.,1.73811241238545));
#32537=CARTESIAN_POINT('',(-1.34869019493419,1.,1.73811241238545));
#32538=CARTESIAN_POINT('',(-1.23627494547115,1.,1.81978687191668));
#32539=CARTESIAN_POINT('',(-1.34869019493419,0.,1.73811241238545));
#32540=CARTESIAN_POINT('Ctrl Pts',(-1.15624053661742,-1.,1.31362392696032));
#32541=CARTESIAN_POINT('Ctrl Pts',(-1.15624053661742,1.,1.31362392696032));
#32542=CARTESIAN_POINT('Ctrl Pts',(-1.15950888730809,-1.,1.31722977216397));
#32543=CARTESIAN_POINT('Ctrl Pts',(-1.15950888730809,1.,1.31722977216397));
#32544=CARTESIAN_POINT('Ctrl Pts',(-1.16589330093588,-1.,1.32428080721772));
#32545=CARTESIAN_POINT('Ctrl Pts',(-1.16589330093588,1.,1.32428080721772));
#32546=CARTESIAN_POINT('Ctrl Pts',(-1.17501305789857,-1.,1.33437539347008));
#32547=CARTESIAN_POINT('Ctrl Pts',(-1.17501305789857,1.,1.33437539347008));
#32548=CARTESIAN_POINT('Ctrl Pts',(-1.18625865667441,-1.,1.34687054001093));
#32549=CARTESIAN_POINT('Ctrl Pts',(-1.18625865667441,1.,1.34687054001093));
#32550=CARTESIAN_POINT('Ctrl Pts',(-1.1987959077932,-1.,1.36088705043885));
#32551=CARTESIAN_POINT('Ctrl Pts',(-1.1987959077932,1.,1.36088705043885));
#32552=CARTESIAN_POINT('Ctrl Pts',(-1.20982812925645,-1.,1.37331915607905));
#32553=CARTESIAN_POINT('Ctrl Pts',(-1.20982812925645,1.,1.37331915607905));
#32554=CARTESIAN_POINT('Ctrl Pts',(-1.21938737280852,-1.,1.38420564527715));
#32555=CARTESIAN_POINT('Ctrl Pts',(-1.21938737280852,1.,1.38420564527715));
#32556=CARTESIAN_POINT('Ctrl Pts',(-1.22752961899387,-1.,1.39361389568796));
#32557=CARTESIAN_POINT('Ctrl Pts',(-1.22752961899387,1.,1.39361389568796));
#32558=CARTESIAN_POINT('Ctrl Pts',(-1.23434087290423,-1.,1.40164708206106));
#32559=CARTESIAN_POINT('Ctrl Pts',(-1.23434087290423,1.,1.40164708206106));
#32560=CARTESIAN_POINT('Ctrl Pts',(-1.23994455029534,-1.,1.40845295531283));
#32561=CARTESIAN_POINT('Ctrl Pts',(-1.23994455029534,1.,1.40845295531283));
#32562=CARTESIAN_POINT('Ctrl Pts',(-1.24450600513056,-1.,1.41422913175179));
#32563=CARTESIAN_POINT('Ctrl Pts',(-1.24450600513056,1.,1.41422913175179));
#32564=CARTESIAN_POINT('Ctrl Pts',(-1.24824430986571,-1.,1.41923722596025));
#32565=CARTESIAN_POINT('Ctrl Pts',(-1.24824430986571,1.,1.41923722596025));
#32566=CARTESIAN_POINT('Ctrl Pts',(-1.2514145557001,-1.,1.42378102115575));
#32567=CARTESIAN_POINT('Ctrl Pts',(-1.2514145557001,1.,1.42378102115575));
#32568=CARTESIAN_POINT('Ctrl Pts',(-1.25426945222639,-1.,1.42815938799387));
#32569=CARTESIAN_POINT('Ctrl Pts',(-1.25426945222639,1.,1.42815938799387));
#32570=CARTESIAN_POINT('Ctrl Pts',(-1.25702687965755,-1.,1.43262645609691));
#32571=CARTESIAN_POINT('Ctrl Pts',(-1.25702687965755,1.,1.43262645609691));
#32572=CARTESIAN_POINT('Ctrl Pts',(-1.25983531012005,-1.,1.43734919180848));
#32573=CARTESIAN_POINT('Ctrl Pts',(-1.25983531012005,1.,1.43734919180848));
#32574=CARTESIAN_POINT('Ctrl Pts',(-1.26273903323859,-1.,1.44236470511303));
#32575=CARTESIAN_POINT('Ctrl Pts',(-1.26273903323859,1.,1.44236470511303));
#32576=CARTESIAN_POINT('Ctrl Pts',(-1.26570925118868,-1.,1.44761985001662));
#32577=CARTESIAN_POINT('Ctrl Pts',(-1.26570925118868,1.,1.44761985001662));
#32578=CARTESIAN_POINT('Ctrl Pts',(-1.2686778680489,-1.,1.45301422764247));
#32579=CARTESIAN_POINT('Ctrl Pts',(-1.2686778680489,1.,1.45301422764247));
#32580=CARTESIAN_POINT('Ctrl Pts',(-1.27156805265289,-1.,1.45843906294697));
#32581=CARTESIAN_POINT('Ctrl Pts',(-1.27156805265289,1.,1.45843906294697));
#32582=CARTESIAN_POINT('Ctrl Pts',(-1.27433119897822,-1.,1.46382431332476));
#32583=CARTESIAN_POINT('Ctrl Pts',(-1.27433119897822,1.,1.46382431332476));
#32584=CARTESIAN_POINT('Ctrl Pts',(-1.27696414831089,-1.,1.46916035917133));
#32585=CARTESIAN_POINT('Ctrl Pts',(-1.27696414831089,1.,1.46916035917133));
#32586=CARTESIAN_POINT('Ctrl Pts',(-1.2794891824849,-1.,1.4744717526707));
#32587=CARTESIAN_POINT('Ctrl Pts',(-1.2794891824849,1.,1.4744717526707));
#32588=CARTESIAN_POINT('Ctrl Pts',(-1.28194158939517,-1.,1.47980070347095));
#32589=CARTESIAN_POINT('Ctrl Pts',(-1.28194158939517,1.,1.47980070347095));
#32590=CARTESIAN_POINT('Ctrl Pts',(-1.28435533880201,-1.,1.4851881711891));
#32591=CARTESIAN_POINT('Ctrl Pts',(-1.28435533880201,1.,1.4851881711891));
#32592=CARTESIAN_POINT('Ctrl Pts',(-1.2867467611644,-1.,1.4906522831278));
#32593=CARTESIAN_POINT('Ctrl Pts',(-1.2867467611644,1.,1.4906522831278));
#32594=CARTESIAN_POINT('Ctrl Pts',(-1.28911506584254,-1.,1.49618896881754));
#32595=CARTESIAN_POINT('Ctrl Pts',(-1.28911506584254,1.,1.49618896881754));
#32596=CARTESIAN_POINT('Ctrl Pts',(-1.29145022885181,-1.,1.50178230149776));
#32597=CARTESIAN_POINT('Ctrl Pts',(-1.29145022885181,1.,1.50178230149776));
#32598=CARTESIAN_POINT('Ctrl Pts',(-1.29373841372842,-1.,1.50741159078365));
#32599=CARTESIAN_POINT('Ctrl Pts',(-1.29373841372842,1.,1.50741159078365));
#32600=CARTESIAN_POINT('Ctrl Pts',(-1.29596850710509,-1.,1.51305994241402));
#32601=CARTESIAN_POINT('Ctrl Pts',(-1.29596850710509,1.,1.51305994241402));
#32602=CARTESIAN_POINT('Ctrl Pts',(-1.29813791800747,-1.,1.51872184912724));
#32603=CARTESIAN_POINT('Ctrl Pts',(-1.29813791800747,1.,1.51872184912724));
#32604=CARTESIAN_POINT('Ctrl Pts',(-1.30024984366328,-1.,1.52439957861062));
#32605=CARTESIAN_POINT('Ctrl Pts',(-1.30024984366328,1.,1.52439957861062));
#32606=CARTESIAN_POINT('Ctrl Pts',(-1.30231064395568,-1.,1.53009970283891));
#32607=CARTESIAN_POINT('Ctrl Pts',(-1.30231064395568,1.,1.53009970283891));
#32608=CARTESIAN_POINT('Ctrl Pts',(-1.30432735639489,-1.,1.53582981268977));
#32609=CARTESIAN_POINT('Ctrl Pts',(-1.30432735639489,1.,1.53582981268977));
#32610=CARTESIAN_POINT('Ctrl Pts',(-1.30630475189556,-1.,1.54159462645432));
#32611=CARTESIAN_POINT('Ctrl Pts',(-1.30630475189556,1.,1.54159462645432));
#32612=CARTESIAN_POINT('Ctrl Pts',(-1.30824393907473,-1.,1.54739413957185));
#32613=CARTESIAN_POINT('Ctrl Pts',(-1.30824393907473,1.,1.54739413957185));
#32614=CARTESIAN_POINT('Ctrl Pts',(-1.31014393684222,-1.,1.55322568759481));
#32615=CARTESIAN_POINT('Ctrl Pts',(-1.31014393684222,1.,1.55322568759481));
#32616=CARTESIAN_POINT('Ctrl Pts',(-1.31200264341696,-1.,1.55908521254821));
#32617=CARTESIAN_POINT('Ctrl Pts',(-1.31200264341696,1.,1.55908521254821));
#32618=CARTESIAN_POINT('Ctrl Pts',(-1.31381795281002,-1.,1.56496872402353));
#32619=CARTESIAN_POINT('Ctrl Pts',(-1.31381795281002,1.,1.56496872402353));
#32620=CARTESIAN_POINT('Ctrl Pts',(-1.31558903860016,-1.,1.57087397835723));
#32621=CARTESIAN_POINT('Ctrl Pts',(-1.31558903860016,1.,1.57087397835723));
#32622=CARTESIAN_POINT('Ctrl Pts',(-1.31731642317187,-1.,1.5768005650559));
#32623=CARTESIAN_POINT('Ctrl Pts',(-1.31731642317187,1.,1.5768005650559));
#32624=CARTESIAN_POINT('Ctrl Pts',(-1.31900135021432,-1.,1.58274907898834));
#32625=CARTESIAN_POINT('Ctrl Pts',(-1.31900135021432,1.,1.58274907898834));
#32626=CARTESIAN_POINT('Ctrl Pts',(-1.32064537110892,-1.,1.58872057258245));
#32627=CARTESIAN_POINT('Ctrl Pts',(-1.32064537110892,1.,1.58872057258245));
#32628=CARTESIAN_POINT('Ctrl Pts',(-1.32224985747682,-1.,1.59471591079403));
#32629=CARTESIAN_POINT('Ctrl Pts',(-1.32224985747682,1.,1.59471591079403));
#32630=CARTESIAN_POINT('Ctrl Pts',(-1.32381550858256,-1.,1.60073511858687));
#32631=CARTESIAN_POINT('Ctrl Pts',(-1.32381550858256,1.,1.60073511858687));
#32632=CARTESIAN_POINT('Ctrl Pts',(-1.32534250785782,-1.,1.60677758290954));
#32633=CARTESIAN_POINT('Ctrl Pts',(-1.32534250785782,1.,1.60677758290954));
#32634=CARTESIAN_POINT('Ctrl Pts',(-1.32683074483356,-1.,1.6128423401575));
#32635=CARTESIAN_POINT('Ctrl Pts',(-1.32683074483356,1.,1.6128423401575));
#32636=CARTESIAN_POINT('Ctrl Pts',(-1.32828000610449,-1.,1.61892832270724));
#32637=CARTESIAN_POINT('Ctrl Pts',(-1.32828000610449,1.,1.61892832270724));
#32638=CARTESIAN_POINT('Ctrl Pts',(-1.3296901950568,-1.,1.62503464209797));
#32639=CARTESIAN_POINT('Ctrl Pts',(-1.3296901950568,1.,1.62503464209797));
#32640=CARTESIAN_POINT('Ctrl Pts',(-1.33106149345645,-1.,1.63116079730923));
#32641=CARTESIAN_POINT('Ctrl Pts',(-1.33106149345645,1.,1.63116079730923));
#32642=CARTESIAN_POINT('Ctrl Pts',(-1.33239425103724,-1.,1.63730653475089));
#32643=CARTESIAN_POINT('Ctrl Pts',(-1.33239425103724,1.,1.63730653475089));
#32644=CARTESIAN_POINT('Ctrl Pts',(-1.33368890676572,-1.,1.6434717485603));
#32645=CARTESIAN_POINT('Ctrl Pts',(-1.33368890676572,1.,1.6434717485603));
#32646=CARTESIAN_POINT('Ctrl Pts',(-1.33494590467993,-1.,1.6496563728683));
#32647=CARTESIAN_POINT('Ctrl Pts',(-1.33494590467993,1.,1.6496563728683));
#32648=CARTESIAN_POINT('Ctrl Pts',(-1.33616559745172,-1.,1.65586025952593));
#32649=CARTESIAN_POINT('Ctrl Pts',(-1.33616559745172,1.,1.65586025952593));
#32650=CARTESIAN_POINT('Ctrl Pts',(-1.33734820885262,-1.,1.66208312541983));
#32651=CARTESIAN_POINT('Ctrl Pts',(-1.33734820885262,1.,1.66208312541983));
#32652=CARTESIAN_POINT('Ctrl Pts',(-1.33849388654388,-1.,1.66832460783989));
#32653=CARTESIAN_POINT('Ctrl Pts',(-1.33849388654388,1.,1.66832460783989));
#32654=CARTESIAN_POINT('Ctrl Pts',(-1.3396027347034,-1.,1.67458429426086));
#32655=CARTESIAN_POINT('Ctrl Pts',(-1.3396027347034,1.,1.67458429426086));
#32656=CARTESIAN_POINT('Ctrl Pts',(-1.34067485185203,-1.,1.68086176030362));
#32657=CARTESIAN_POINT('Ctrl Pts',(-1.34067485185203,1.,1.68086176030362));
#32658=CARTESIAN_POINT('Ctrl Pts',(-1.341710374848,-1.,1.68715660868764));
#32659=CARTESIAN_POINT('Ctrl Pts',(-1.341710374848,1.,1.68715660868764));
#32660=CARTESIAN_POINT('Ctrl Pts',(-1.34270948206319,-1.,1.6934684849687));
#32661=CARTESIAN_POINT('Ctrl Pts',(-1.34270948206319,1.,1.6934684849687));
#32662=CARTESIAN_POINT('Ctrl Pts',(-1.34367237124483,-1.,1.69979707754427));
#32663=CARTESIAN_POINT('Ctrl Pts',(-1.34367237124483,1.,1.69979707754427));
#32664=CARTESIAN_POINT('Ctrl Pts',(-1.34459924533831,-1.,1.70614212266738));
#32665=CARTESIAN_POINT('Ctrl Pts',(-1.34459924533831,1.,1.70614212266738));
#32666=CARTESIAN_POINT('Ctrl Pts',(-1.34549029589416,-1.,1.71250340686822));
#32667=CARTESIAN_POINT('Ctrl Pts',(-1.34549029589416,1.,1.71250340686822));
#32668=CARTESIAN_POINT('Ctrl Pts',(-1.34634568653227,-1.,1.7188807715049));
#32669=CARTESIAN_POINT('Ctrl Pts',(-1.34634568653227,1.,1.7188807715049));
#32670=CARTESIAN_POINT('Ctrl Pts',(-1.34716554819527,-1.,1.72527410680674));
#32671=CARTESIAN_POINT('Ctrl Pts',(-1.34716554819527,1.,1.72527410680674));
#32672=CARTESIAN_POINT('Ctrl Pts',(-1.34779309152035,-1.,1.7304014965394));
#32673=CARTESIAN_POINT('Ctrl Pts',(-1.34779309152035,1.,1.7304014965394));
#32674=CARTESIAN_POINT('Ctrl Pts',(-1.34824783112887,-1.,1.73425417885907));
#32675=CARTESIAN_POINT('Ctrl Pts',(-1.34824783112887,1.,1.73425417885907));
#32676=CARTESIAN_POINT('Ctrl Pts',(-1.34854391898045,-1.,1.73682580585691));
#32677=CARTESIAN_POINT('Ctrl Pts',(-1.34854391898045,1.,1.73682580585691));
#32678=CARTESIAN_POINT('Ctrl Pts',(-1.34869019493419,-1.,1.73811241238545));
#32679=CARTESIAN_POINT('Ctrl Pts',(-1.34869019493419,1.,1.73811241238545));
#32680=CARTESIAN_POINT('',(-1.15624053661742,1.,1.31362392696032));
#32681=CARTESIAN_POINT('Ctrl Pts',(-1.15624053661742,1.,1.31362392696032));
#32682=CARTESIAN_POINT('Ctrl Pts',(-1.15950888730809,1.,1.31722977216397));
#32683=CARTESIAN_POINT('Ctrl Pts',(-1.16589330093588,1.,1.32428080721772));
#32684=CARTESIAN_POINT('Ctrl Pts',(-1.17501305789857,1.,1.33437539347008));
#32685=CARTESIAN_POINT('Ctrl Pts',(-1.18625865667441,1.,1.34687054001093));
#32686=CARTESIAN_POINT('Ctrl Pts',(-1.1987959077932,1.,1.36088705043885));
#32687=CARTESIAN_POINT('Ctrl Pts',(-1.20982812925645,1.,1.37331915607905));
#32688=CARTESIAN_POINT('Ctrl Pts',(-1.21938737280852,1.,1.38420564527715));
#32689=CARTESIAN_POINT('Ctrl Pts',(-1.22752961899387,1.,1.39361389568796));
#32690=CARTESIAN_POINT('Ctrl Pts',(-1.23434087290423,1.,1.40164708206106));
#32691=CARTESIAN_POINT('Ctrl Pts',(-1.23994455029534,1.,1.40845295531283));
#32692=CARTESIAN_POINT('Ctrl Pts',(-1.24450600513056,1.,1.41422913175179));
#32693=CARTESIAN_POINT('Ctrl Pts',(-1.24824430986571,1.,1.41923722596025));
#32694=CARTESIAN_POINT('Ctrl Pts',(-1.2514145557001,1.,1.42378102115575));
#32695=CARTESIAN_POINT('Ctrl Pts',(-1.25426945222639,1.,1.42815938799387));
#32696=CARTESIAN_POINT('Ctrl Pts',(-1.25702687965755,1.,1.43262645609691));
#32697=CARTESIAN_POINT('Ctrl Pts',(-1.25983531012005,1.,1.43734919180848));
#32698=CARTESIAN_POINT('Ctrl Pts',(-1.26273903323859,1.,1.44236470511303));
#32699=CARTESIAN_POINT('Ctrl Pts',(-1.26570925118868,1.,1.44761985001662));
#32700=CARTESIAN_POINT('Ctrl Pts',(-1.2686778680489,1.,1.45301422764247));
#32701=CARTESIAN_POINT('Ctrl Pts',(-1.27156805265289,1.,1.45843906294697));
#32702=CARTESIAN_POINT('Ctrl Pts',(-1.27433119897822,1.,1.46382431332476));
#32703=CARTESIAN_POINT('Ctrl Pts',(-1.27696414831089,1.,1.46916035917133));
#32704=CARTESIAN_POINT('Ctrl Pts',(-1.2794891824849,1.,1.4744717526707));
#32705=CARTESIAN_POINT('Ctrl Pts',(-1.28194158939517,1.,1.47980070347095));
#32706=CARTESIAN_POINT('Ctrl Pts',(-1.28435533880201,1.,1.4851881711891));
#32707=CARTESIAN_POINT('Ctrl Pts',(-1.2867467611644,1.,1.4906522831278));
#32708=CARTESIAN_POINT('Ctrl Pts',(-1.28911506584254,1.,1.49618896881754));
#32709=CARTESIAN_POINT('Ctrl Pts',(-1.29145022885181,1.,1.50178230149776));
#32710=CARTESIAN_POINT('Ctrl Pts',(-1.29373841372842,1.,1.50741159078365));
#32711=CARTESIAN_POINT('Ctrl Pts',(-1.29596850710509,1.,1.51305994241402));
#32712=CARTESIAN_POINT('Ctrl Pts',(-1.29813791800747,1.,1.51872184912724));
#32713=CARTESIAN_POINT('Ctrl Pts',(-1.30024984366328,1.,1.52439957861062));
#32714=CARTESIAN_POINT('Ctrl Pts',(-1.30231064395568,1.,1.53009970283891));
#32715=CARTESIAN_POINT('Ctrl Pts',(-1.30432735639489,1.,1.53582981268977));
#32716=CARTESIAN_POINT('Ctrl Pts',(-1.30630475189556,1.,1.54159462645432));
#32717=CARTESIAN_POINT('Ctrl Pts',(-1.30824393907473,1.,1.54739413957185));
#32718=CARTESIAN_POINT('Ctrl Pts',(-1.31014393684222,1.,1.55322568759481));
#32719=CARTESIAN_POINT('Ctrl Pts',(-1.31200264341696,1.,1.55908521254821));
#32720=CARTESIAN_POINT('Ctrl Pts',(-1.31381795281002,1.,1.56496872402353));
#32721=CARTESIAN_POINT('Ctrl Pts',(-1.31558903860016,1.,1.57087397835723));
#32722=CARTESIAN_POINT('Ctrl Pts',(-1.31731642317187,1.,1.5768005650559));
#32723=CARTESIAN_POINT('Ctrl Pts',(-1.31900135021432,1.,1.58274907898834));
#32724=CARTESIAN_POINT('Ctrl Pts',(-1.32064537110892,1.,1.58872057258245));
#32725=CARTESIAN_POINT('Ctrl Pts',(-1.32224985747682,1.,1.59471591079403));
#32726=CARTESIAN_POINT('Ctrl Pts',(-1.32381550858256,1.,1.60073511858687));
#32727=CARTESIAN_POINT('Ctrl Pts',(-1.32534250785782,1.,1.60677758290954));
#32728=CARTESIAN_POINT('Ctrl Pts',(-1.32683074483356,1.,1.6128423401575));
#32729=CARTESIAN_POINT('Ctrl Pts',(-1.32828000610449,1.,1.61892832270724));
#32730=CARTESIAN_POINT('Ctrl Pts',(-1.3296901950568,1.,1.62503464209797));
#32731=CARTESIAN_POINT('Ctrl Pts',(-1.33106149345645,1.,1.63116079730923));
#32732=CARTESIAN_POINT('Ctrl Pts',(-1.33239425103724,1.,1.63730653475089));
#32733=CARTESIAN_POINT('Ctrl Pts',(-1.33368890676572,1.,1.6434717485603));
#32734=CARTESIAN_POINT('Ctrl Pts',(-1.33494590467993,1.,1.6496563728683));
#32735=CARTESIAN_POINT('Ctrl Pts',(-1.33616559745172,1.,1.65586025952593));
#32736=CARTESIAN_POINT('Ctrl Pts',(-1.33734820885262,1.,1.66208312541983));
#32737=CARTESIAN_POINT('Ctrl Pts',(-1.33849388654388,1.,1.66832460783989));
#32738=CARTESIAN_POINT('Ctrl Pts',(-1.3396027347034,1.,1.67458429426086));
#32739=CARTESIAN_POINT('Ctrl Pts',(-1.34067485185203,1.,1.68086176030362));
#32740=CARTESIAN_POINT('Ctrl Pts',(-1.341710374848,1.,1.68715660868764));
#32741=CARTESIAN_POINT('Ctrl Pts',(-1.34270948206319,1.,1.6934684849687));
#32742=CARTESIAN_POINT('Ctrl Pts',(-1.34367237124483,1.,1.69979707754427));
#32743=CARTESIAN_POINT('Ctrl Pts',(-1.34459924533831,1.,1.70614212266738));
#32744=CARTESIAN_POINT('Ctrl Pts',(-1.34549029589416,1.,1.71250340686822));
#32745=CARTESIAN_POINT('Ctrl Pts',(-1.34634568653227,1.,1.7188807715049));
#32746=CARTESIAN_POINT('Ctrl Pts',(-1.34716554819527,1.,1.72527410680674));
#32747=CARTESIAN_POINT('Ctrl Pts',(-1.34779309152035,1.,1.7304014965394));
#32748=CARTESIAN_POINT('Ctrl Pts',(-1.34824783112887,1.,1.73425417885907));
#32749=CARTESIAN_POINT('Ctrl Pts',(-1.34854391898045,1.,1.73682580585691));
#32750=CARTESIAN_POINT('Ctrl Pts',(-1.34869019493419,1.,1.73811241238545));
#32751=CARTESIAN_POINT('',(-1.15624053661742,0.,1.31362392696032));
#32752=CARTESIAN_POINT('Origin',(0.,0.,0.));
#32753=CARTESIAN_POINT('',(-1.31362392696033,1.,1.15624053661742));
#32754=CARTESIAN_POINT('Origin',(0.,1.,0.));
#32755=CARTESIAN_POINT('',(-1.31362392696033,0.,1.15624053661742));
#32756=CARTESIAN_POINT('Ctrl Pts',(-1.73811241238545,-1.,1.34869019493419));
#32757=CARTESIAN_POINT('Ctrl Pts',(-1.73811241238545,1.,1.34869019493419));
#32758=CARTESIAN_POINT('Ctrl Pts',(-1.73682580585819,-1.,1.34854391898145));
#32759=CARTESIAN_POINT('Ctrl Pts',(-1.73682580585819,1.,1.34854391898145));
#32760=CARTESIAN_POINT('Ctrl Pts',(-1.73425417886255,-1.,1.34824783113158));
#32761=CARTESIAN_POINT('Ctrl Pts',(-1.73425417886255,1.,1.34824783113158));
#32762=CARTESIAN_POINT('Ctrl Pts',(-1.73040149654497,-1.,1.3477930915247));
#32763=CARTESIAN_POINT('Ctrl Pts',(-1.73040149654497,1.,1.3477930915247));
#32764=CARTESIAN_POINT('Ctrl Pts',(-1.72527410681298,-1.,1.34716554820013));
#32765=CARTESIAN_POINT('Ctrl Pts',(-1.72527410681298,1.,1.34716554820013));
#32766=CARTESIAN_POINT('Ctrl Pts',(-1.7188807715095,-1.,1.34634568653586));
#32767=CARTESIAN_POINT('Ctrl Pts',(-1.7188807715095,1.,1.34634568653586));
#32768=CARTESIAN_POINT('Ctrl Pts',(-1.71250340687011,-1.,1.34549029589563));
#32769=CARTESIAN_POINT('Ctrl Pts',(-1.71250340687011,1.,1.34549029589563));
#32770=CARTESIAN_POINT('Ctrl Pts',(-1.70614212266676,-1.,1.34459924533783));
#32771=CARTESIAN_POINT('Ctrl Pts',(-1.70614212266676,1.,1.34459924533783));
#32772=CARTESIAN_POINT('Ctrl Pts',(-1.69979707754221,-1.,1.34367237124322));
#32773=CARTESIAN_POINT('Ctrl Pts',(-1.69979707754221,1.,1.34367237124322));
#32774=CARTESIAN_POINT('Ctrl Pts',(-1.6934684849664,-1.,1.34270948206139));
#32775=CARTESIAN_POINT('Ctrl Pts',(-1.6934684849664,1.,1.34270948206139));
#32776=CARTESIAN_POINT('Ctrl Pts',(-1.68715660868602,-1.,1.34171037484673));
#32777=CARTESIAN_POINT('Ctrl Pts',(-1.68715660868602,1.,1.34171037484673));
#32778=CARTESIAN_POINT('Ctrl Pts',(-1.68086176030308,-1.,1.3406748518516));
#32779=CARTESIAN_POINT('Ctrl Pts',(-1.68086176030308,1.,1.3406748518516));
#32780=CARTESIAN_POINT('Ctrl Pts',(-1.67458429426126,-1.,1.33960273470372));
#32781=CARTESIAN_POINT('Ctrl Pts',(-1.67458429426126,1.,1.33960273470372));
#32782=CARTESIAN_POINT('Ctrl Pts',(-1.66832460784078,-1.,1.33849388654458));
#32783=CARTESIAN_POINT('Ctrl Pts',(-1.66832460784078,1.,1.33849388654458));
#32784=CARTESIAN_POINT('Ctrl Pts',(-1.66208312542073,-1.,1.33734820885331));
#32785=CARTESIAN_POINT('Ctrl Pts',(-1.66208312542073,1.,1.33734820885331));
#32786=CARTESIAN_POINT('Ctrl Pts',(-1.65586025952651,-1.,1.33616559745217));
#32787=CARTESIAN_POINT('Ctrl Pts',(-1.65586025952651,1.,1.33616559745217));
#32788=CARTESIAN_POINT('Ctrl Pts',(-1.64965637286843,-1.,1.33494590468003));
#32789=CARTESIAN_POINT('Ctrl Pts',(-1.64965637286843,1.,1.33494590468003));
#32790=CARTESIAN_POINT('Ctrl Pts',(-1.64347174856007,-1.,1.33368890676554));
#32791=CARTESIAN_POINT('Ctrl Pts',(-1.64347174856007,1.,1.33368890676554));
#32792=CARTESIAN_POINT('Ctrl Pts',(-1.6373065347505,-1.,1.33239425103694));
#32793=CARTESIAN_POINT('Ctrl Pts',(-1.6373065347505,1.,1.33239425103694));
#32794=CARTESIAN_POINT('Ctrl Pts',(-1.63116079730887,-1.,1.33106149345618));
#32795=CARTESIAN_POINT('Ctrl Pts',(-1.63116079730887,1.,1.33106149345618));
#32796=CARTESIAN_POINT('Ctrl Pts',(-1.62503464209777,-1.,1.32969019505665));
#32797=CARTESIAN_POINT('Ctrl Pts',(-1.62503464209777,1.,1.32969019505665));
#32798=CARTESIAN_POINT('Ctrl Pts',(-1.61892832270723,-1.,1.32828000610448));
#32799=CARTESIAN_POINT('Ctrl Pts',(-1.61892832270723,1.,1.32828000610448));
#32800=CARTESIAN_POINT('Ctrl Pts',(-1.61284234015762,-1.,1.32683074483365));
#32801=CARTESIAN_POINT('Ctrl Pts',(-1.61284234015762,1.,1.32683074483365));
#32802=CARTESIAN_POINT('Ctrl Pts',(-1.6067775829097,-1.,1.32534250785794));
#32803=CARTESIAN_POINT('Ctrl Pts',(-1.6067775829097,1.,1.32534250785794));
#32804=CARTESIAN_POINT('Ctrl Pts',(-1.600735118587,-1.,1.32381550858266));
#32805=CARTESIAN_POINT('Ctrl Pts',(-1.600735118587,1.,1.32381550858266));
#32806=CARTESIAN_POINT('Ctrl Pts',(-1.59471591079408,-1.,1.32224985747686));
#32807=CARTESIAN_POINT('Ctrl Pts',(-1.59471591079408,1.,1.32224985747686));
#32808=CARTESIAN_POINT('Ctrl Pts',(-1.58872057258244,-1.,1.32064537110891));
#32809=CARTESIAN_POINT('Ctrl Pts',(-1.58872057258244,1.,1.32064537110891));
#32810=CARTESIAN_POINT('Ctrl Pts',(-1.58274907898829,-1.,1.31900135021428));
#32811=CARTESIAN_POINT('Ctrl Pts',(-1.58274907898829,1.,1.31900135021428));
#32812=CARTESIAN_POINT('Ctrl Pts',(-1.57680056505585,-1.,1.31731642317183));
#32813=CARTESIAN_POINT('Ctrl Pts',(-1.57680056505585,1.,1.31731642317183));
#32814=CARTESIAN_POINT('Ctrl Pts',(-1.57087397835721,-1.,1.31558903860015));
#32815=CARTESIAN_POINT('Ctrl Pts',(-1.57087397835721,1.,1.31558903860015));
#32816=CARTESIAN_POINT('Ctrl Pts',(-1.56496872402352,-1.,1.31381795281002));
#32817=CARTESIAN_POINT('Ctrl Pts',(-1.56496872402352,1.,1.31381795281002));
#32818=CARTESIAN_POINT('Ctrl Pts',(-1.55908521254822,-1.,1.31200264341696));
#32819=CARTESIAN_POINT('Ctrl Pts',(-1.55908521254822,1.,1.31200264341696));
#32820=CARTESIAN_POINT('Ctrl Pts',(-1.55322568759481,-1.,1.31014393684221));
#32821=CARTESIAN_POINT('Ctrl Pts',(-1.55322568759481,1.,1.31014393684221));
#32822=CARTESIAN_POINT('Ctrl Pts',(-1.54739413957183,-1.,1.30824393907471));
#32823=CARTESIAN_POINT('Ctrl Pts',(-1.54739413957183,1.,1.30824393907471));
#32824=CARTESIAN_POINT('Ctrl Pts',(-1.54159462645428,-1.,1.30630475189553));
#32825=CARTESIAN_POINT('Ctrl Pts',(-1.54159462645428,1.,1.30630475189553));
#32826=CARTESIAN_POINT('Ctrl Pts',(-1.53582981268976,-1.,1.30432735639487));
#32827=CARTESIAN_POINT('Ctrl Pts',(-1.53582981268976,1.,1.30432735639487));
#32828=CARTESIAN_POINT('Ctrl Pts',(-1.53009970283893,-1.,1.3023106439557));
#32829=CARTESIAN_POINT('Ctrl Pts',(-1.53009970283893,1.,1.3023106439557));
#32830=CARTESIAN_POINT('Ctrl Pts',(-1.5243995786107,-1.,1.30024984366334));
#32831=CARTESIAN_POINT('Ctrl Pts',(-1.5243995786107,1.,1.30024984366334));
#32832=CARTESIAN_POINT('Ctrl Pts',(-1.51872184912735,-1.,1.29813791800757));
#32833=CARTESIAN_POINT('Ctrl Pts',(-1.51872184912735,1.,1.29813791800757));
#32834=CARTESIAN_POINT('Ctrl Pts',(-1.51305994241412,-1.,1.29596850710518));
#32835=CARTESIAN_POINT('Ctrl Pts',(-1.51305994241412,1.,1.29596850710518));
#32836=CARTESIAN_POINT('Ctrl Pts',(-1.50741159078367,-1.,1.29373841372843));
#32837=CARTESIAN_POINT('Ctrl Pts',(-1.50741159078367,1.,1.29373841372843));
#32838=CARTESIAN_POINT('Ctrl Pts',(-1.50178230149764,-1.,1.29145022885171));
#32839=CARTESIAN_POINT('Ctrl Pts',(-1.50178230149764,1.,1.29145022885171));
#32840=CARTESIAN_POINT('Ctrl Pts',(-1.49618896881729,-1.,1.28911506584232));
#32841=CARTESIAN_POINT('Ctrl Pts',(-1.49618896881729,1.,1.28911506584232));
#32842=CARTESIAN_POINT('Ctrl Pts',(-1.4906522831275,-1.,1.28674676116415));
#32843=CARTESIAN_POINT('Ctrl Pts',(-1.4906522831275,1.,1.28674676116415));
#32844=CARTESIAN_POINT('Ctrl Pts',(-1.48518817118891,-1.,1.28435533880184));
#32845=CARTESIAN_POINT('Ctrl Pts',(-1.48518817118891,1.,1.28435533880184));
#32846=CARTESIAN_POINT('Ctrl Pts',(-1.47980070347102,-1.,1.28194158939522));
#32847=CARTESIAN_POINT('Ctrl Pts',(-1.47980070347102,1.,1.28194158939522));
#32848=CARTESIAN_POINT('Ctrl Pts',(-1.4744717526711,-1.,1.27948918248524));
#32849=CARTESIAN_POINT('Ctrl Pts',(-1.4744717526711,1.,1.27948918248524));
#32850=CARTESIAN_POINT('Ctrl Pts',(-1.46916035917197,-1.,1.27696414831144));
#32851=CARTESIAN_POINT('Ctrl Pts',(-1.46916035917197,1.,1.27696414831144));
#32852=CARTESIAN_POINT('Ctrl Pts',(-1.4638243133254,-1.,1.27433119897877));
#32853=CARTESIAN_POINT('Ctrl Pts',(-1.4638243133254,1.,1.27433119897877));
#32854=CARTESIAN_POINT('Ctrl Pts',(-1.45843906294725,-1.,1.27156805265312));
#32855=CARTESIAN_POINT('Ctrl Pts',(-1.45843906294725,1.,1.27156805265312));
#32856=CARTESIAN_POINT('Ctrl Pts',(-1.45301422764205,-1.,1.26867786804854));
#32857=CARTESIAN_POINT('Ctrl Pts',(-1.45301422764205,1.,1.26867786804854));
#32858=CARTESIAN_POINT('Ctrl Pts',(-1.44761985001544,-1.,1.26570925118767));
#32859=CARTESIAN_POINT('Ctrl Pts',(-1.44761985001544,1.,1.26570925118767));
#32860=CARTESIAN_POINT('Ctrl Pts',(-1.44236470511145,-1.,1.26273903323723));
#32861=CARTESIAN_POINT('Ctrl Pts',(-1.44236470511145,1.,1.26273903323723));
#32862=CARTESIAN_POINT('Ctrl Pts',(-1.43734919180719,-1.,1.25983531011894));
#32863=CARTESIAN_POINT('Ctrl Pts',(-1.43734919180719,1.,1.25983531011894));
#32864=CARTESIAN_POINT('Ctrl Pts',(-1.43262645609679,-1.,1.25702687965744));
#32865=CARTESIAN_POINT('Ctrl Pts',(-1.43262645609679,1.,1.25702687965744));
#32866=CARTESIAN_POINT('Ctrl Pts',(-1.42815938799555,-1.,1.25426945222783));
#32867=CARTESIAN_POINT('Ctrl Pts',(-1.42815938799555,1.,1.25426945222783));
#32868=CARTESIAN_POINT('Ctrl Pts',(-1.42378102115911,-1.,1.25141455570299));
#32869=CARTESIAN_POINT('Ctrl Pts',(-1.42378102115911,1.,1.25141455570299));
#32870=CARTESIAN_POINT('Ctrl Pts',(-1.41923722596421,-1.,1.24824430986911));
#32871=CARTESIAN_POINT('Ctrl Pts',(-1.41923722596421,1.,1.24824430986911));
#32872=CARTESIAN_POINT('Ctrl Pts',(-1.41422913175437,-1.,1.24450600513278));
#32873=CARTESIAN_POINT('Ctrl Pts',(-1.41422913175437,1.,1.24450600513278));
#32874=CARTESIAN_POINT('Ctrl Pts',(-1.40845295531151,-1.,1.23994455029421));
#32875=CARTESIAN_POINT('Ctrl Pts',(-1.40845295531151,1.,1.23994455029421));
#32876=CARTESIAN_POINT('Ctrl Pts',(-1.40164708205345,-1.,1.23434087289768));
#32877=CARTESIAN_POINT('Ctrl Pts',(-1.40164708205345,1.,1.23434087289768));
#32878=CARTESIAN_POINT('Ctrl Pts',(-1.39361389567257,-1.,1.22752961898063));
#32879=CARTESIAN_POINT('Ctrl Pts',(-1.39361389567257,1.,1.22752961898063));
#32880=CARTESIAN_POINT('Ctrl Pts',(-1.38420564525391,-1.,1.21938737278853));
#32881=CARTESIAN_POINT('Ctrl Pts',(-1.38420564525391,1.,1.21938737278853));
#32882=CARTESIAN_POINT('Ctrl Pts',(-1.37331915604962,-1.,1.20982812923113));
#32883=CARTESIAN_POINT('Ctrl Pts',(-1.37331915604962,1.,1.20982812923113));
#32884=CARTESIAN_POINT('Ctrl Pts',(-1.36088705040677,-1.,1.1987959077656));
#32885=CARTESIAN_POINT('Ctrl Pts',(-1.36088705040677,1.,1.1987959077656));
#32886=CARTESIAN_POINT('Ctrl Pts',(-1.34687053998157,-1.,1.18625865664915));
#32887=CARTESIAN_POINT('Ctrl Pts',(-1.34687053998157,1.,1.18625865664915));
#32888=CARTESIAN_POINT('Ctrl Pts',(-1.33437539344842,-1.,1.17501305787994));
#32889=CARTESIAN_POINT('Ctrl Pts',(-1.33437539344842,1.,1.17501305787994));
#32890=CARTESIAN_POINT('Ctrl Pts',(-1.32428080720544,-1.,1.16589330092532));
#32891=CARTESIAN_POINT('Ctrl Pts',(-1.32428080720544,1.,1.16589330092532));
#32892=CARTESIAN_POINT('Ctrl Pts',(-1.3172297721596,-1.,1.15950888730433));
#32893=CARTESIAN_POINT('Ctrl Pts',(-1.3172297721596,1.,1.15950888730433));
#32894=CARTESIAN_POINT('Ctrl Pts',(-1.31362392696033,-1.,1.15624053661742));
#32895=CARTESIAN_POINT('Ctrl Pts',(-1.31362392696033,1.,1.15624053661742));
#32896=CARTESIAN_POINT('',(-1.73811241238545,1.,1.34869019493419));
#32897=CARTESIAN_POINT('Ctrl Pts',(-1.73811241238545,1.,1.34869019493419));
#32898=CARTESIAN_POINT('Ctrl Pts',(-1.73682580585819,1.,1.34854391898145));
#32899=CARTESIAN_POINT('Ctrl Pts',(-1.73425417886255,1.,1.34824783113158));
#32900=CARTESIAN_POINT('Ctrl Pts',(-1.73040149654497,1.,1.3477930915247));
#32901=CARTESIAN_POINT('Ctrl Pts',(-1.72527410681298,1.,1.34716554820013));
#32902=CARTESIAN_POINT('Ctrl Pts',(-1.7188807715095,1.,1.34634568653586));
#32903=CARTESIAN_POINT('Ctrl Pts',(-1.71250340687011,1.,1.34549029589563));
#32904=CARTESIAN_POINT('Ctrl Pts',(-1.70614212266676,1.,1.34459924533783));
#32905=CARTESIAN_POINT('Ctrl Pts',(-1.69979707754221,1.,1.34367237124322));
#32906=CARTESIAN_POINT('Ctrl Pts',(-1.6934684849664,1.,1.34270948206139));
#32907=CARTESIAN_POINT('Ctrl Pts',(-1.68715660868602,1.,1.34171037484673));
#32908=CARTESIAN_POINT('Ctrl Pts',(-1.68086176030308,1.,1.3406748518516));
#32909=CARTESIAN_POINT('Ctrl Pts',(-1.67458429426126,1.,1.33960273470372));
#32910=CARTESIAN_POINT('Ctrl Pts',(-1.66832460784078,1.,1.33849388654458));
#32911=CARTESIAN_POINT('Ctrl Pts',(-1.66208312542073,1.,1.33734820885331));
#32912=CARTESIAN_POINT('Ctrl Pts',(-1.65586025952651,1.,1.33616559745217));
#32913=CARTESIAN_POINT('Ctrl Pts',(-1.64965637286843,1.,1.33494590468003));
#32914=CARTESIAN_POINT('Ctrl Pts',(-1.64347174856007,1.,1.33368890676554));
#32915=CARTESIAN_POINT('Ctrl Pts',(-1.6373065347505,1.,1.33239425103694));
#32916=CARTESIAN_POINT('Ctrl Pts',(-1.63116079730887,1.,1.33106149345618));
#32917=CARTESIAN_POINT('Ctrl Pts',(-1.62503464209777,1.,1.32969019505665));
#32918=CARTESIAN_POINT('Ctrl Pts',(-1.61892832270723,1.,1.32828000610448));
#32919=CARTESIAN_POINT('Ctrl Pts',(-1.61284234015762,1.,1.32683074483365));
#32920=CARTESIAN_POINT('Ctrl Pts',(-1.6067775829097,1.,1.32534250785794));
#32921=CARTESIAN_POINT('Ctrl Pts',(-1.600735118587,1.,1.32381550858266));
#32922=CARTESIAN_POINT('Ctrl Pts',(-1.59471591079408,1.,1.32224985747686));
#32923=CARTESIAN_POINT('Ctrl Pts',(-1.58872057258244,1.,1.32064537110891));
#32924=CARTESIAN_POINT('Ctrl Pts',(-1.58274907898829,1.,1.31900135021428));
#32925=CARTESIAN_POINT('Ctrl Pts',(-1.57680056505585,1.,1.31731642317183));
#32926=CARTESIAN_POINT('Ctrl Pts',(-1.57087397835721,1.,1.31558903860015));
#32927=CARTESIAN_POINT('Ctrl Pts',(-1.56496872402352,1.,1.31381795281002));
#32928=CARTESIAN_POINT('Ctrl Pts',(-1.55908521254822,1.,1.31200264341696));
#32929=CARTESIAN_POINT('Ctrl Pts',(-1.55322568759481,1.,1.31014393684221));
#32930=CARTESIAN_POINT('Ctrl Pts',(-1.54739413957183,1.,1.30824393907471));
#32931=CARTESIAN_POINT('Ctrl Pts',(-1.54159462645428,1.,1.30630475189553));
#32932=CARTESIAN_POINT('Ctrl Pts',(-1.53582981268976,1.,1.30432735639487));
#32933=CARTESIAN_POINT('Ctrl Pts',(-1.53009970283893,1.,1.3023106439557));
#32934=CARTESIAN_POINT('Ctrl Pts',(-1.5243995786107,1.,1.30024984366334));
#32935=CARTESIAN_POINT('Ctrl Pts',(-1.51872184912735,1.,1.29813791800757));
#32936=CARTESIAN_POINT('Ctrl Pts',(-1.51305994241412,1.,1.29596850710518));
#32937=CARTESIAN_POINT('Ctrl Pts',(-1.50741159078367,1.,1.29373841372843));
#32938=CARTESIAN_POINT('Ctrl Pts',(-1.50178230149764,1.,1.29145022885171));
#32939=CARTESIAN_POINT('Ctrl Pts',(-1.49618896881729,1.,1.28911506584232));
#32940=CARTESIAN_POINT('Ctrl Pts',(-1.4906522831275,1.,1.28674676116415));
#32941=CARTESIAN_POINT('Ctrl Pts',(-1.48518817118891,1.,1.28435533880184));
#32942=CARTESIAN_POINT('Ctrl Pts',(-1.47980070347102,1.,1.28194158939522));
#32943=CARTESIAN_POINT('Ctrl Pts',(-1.4744717526711,1.,1.27948918248524));
#32944=CARTESIAN_POINT('Ctrl Pts',(-1.46916035917197,1.,1.27696414831144));
#32945=CARTESIAN_POINT('Ctrl Pts',(-1.4638243133254,1.,1.27433119897877));
#32946=CARTESIAN_POINT('Ctrl Pts',(-1.45843906294725,1.,1.27156805265312));
#32947=CARTESIAN_POINT('Ctrl Pts',(-1.45301422764205,1.,1.26867786804854));
#32948=CARTESIAN_POINT('Ctrl Pts',(-1.44761985001544,1.,1.26570925118767));
#32949=CARTESIAN_POINT('Ctrl Pts',(-1.44236470511145,1.,1.26273903323723));
#32950=CARTESIAN_POINT('Ctrl Pts',(-1.43734919180719,1.,1.25983531011894));
#32951=CARTESIAN_POINT('Ctrl Pts',(-1.43262645609679,1.,1.25702687965744));
#32952=CARTESIAN_POINT('Ctrl Pts',(-1.42815938799555,1.,1.25426945222783));
#32953=CARTESIAN_POINT('Ctrl Pts',(-1.42378102115911,1.,1.25141455570299));
#32954=CARTESIAN_POINT('Ctrl Pts',(-1.41923722596421,1.,1.24824430986911));
#32955=CARTESIAN_POINT('Ctrl Pts',(-1.41422913175437,1.,1.24450600513278));
#32956=CARTESIAN_POINT('Ctrl Pts',(-1.40845295531151,1.,1.23994455029421));
#32957=CARTESIAN_POINT('Ctrl Pts',(-1.40164708205345,1.,1.23434087289768));
#32958=CARTESIAN_POINT('Ctrl Pts',(-1.39361389567257,1.,1.22752961898063));
#32959=CARTESIAN_POINT('Ctrl Pts',(-1.38420564525391,1.,1.21938737278853));
#32960=CARTESIAN_POINT('Ctrl Pts',(-1.37331915604962,1.,1.20982812923113));
#32961=CARTESIAN_POINT('Ctrl Pts',(-1.36088705040677,1.,1.1987959077656));
#32962=CARTESIAN_POINT('Ctrl Pts',(-1.34687053998157,1.,1.18625865664915));
#32963=CARTESIAN_POINT('Ctrl Pts',(-1.33437539344842,1.,1.17501305787994));
#32964=CARTESIAN_POINT('Ctrl Pts',(-1.32428080720544,1.,1.16589330092532));
#32965=CARTESIAN_POINT('Ctrl Pts',(-1.3172297721596,1.,1.15950888730433));
#32966=CARTESIAN_POINT('Ctrl Pts',(-1.31362392696033,1.,1.15624053661742));
#32967=CARTESIAN_POINT('',(-1.73811241238545,0.,1.34869019493419));
#32968=CARTESIAN_POINT('Origin',(-1.81978687191668,0.,1.23627494547115));
#32969=CARTESIAN_POINT('',(-1.81978687191668,1.,1.23627494547115));
#32970=CARTESIAN_POINT('',(-1.73811241238545,1.,1.34869019493419));
#32971=CARTESIAN_POINT('',(-1.81978687191668,0.,1.23627494547115));
#32972=CARTESIAN_POINT('Ctrl Pts',(-1.5055822144029,-1.,0.892032620296855));
#32973=CARTESIAN_POINT('Ctrl Pts',(-1.5055822144029,1.,0.892032620296855));
#32974=CARTESIAN_POINT('Ctrl Pts',(-1.50980486807181,-1.,0.894452006967538));
#32975=CARTESIAN_POINT('Ctrl Pts',(-1.50980486807181,1.,0.894452006967538));
#32976=CARTESIAN_POINT('Ctrl Pts',(-1.51805569591479,-1.,0.89918504749193));
#32977=CARTESIAN_POINT('Ctrl Pts',(-1.51805569591479,1.,0.89918504749193));
#32978=CARTESIAN_POINT('Ctrl Pts',(-1.52984849890434,-1.,0.905967409640499));
#32979=CARTESIAN_POINT('Ctrl Pts',(-1.52984849890434,1.,0.905967409640499));
#32980=CARTESIAN_POINT('Ctrl Pts',(-1.54440491152808,-1.,0.91437591904658));
#32981=CARTESIAN_POINT('Ctrl Pts',(-1.54440491152808,1.,0.91437591904658));
#32982=CARTESIAN_POINT('Ctrl Pts',(-1.56065988582509,-1.,0.923832188966322));
#32983=CARTESIAN_POINT('Ctrl Pts',(-1.56065988582509,1.,0.923832188966322));
#32984=CARTESIAN_POINT('Ctrl Pts',(-1.57499388385561,-1.,0.932246680128849));
#32985=CARTESIAN_POINT('Ctrl Pts',(-1.57499388385561,1.,0.932246680128849));
#32986=CARTESIAN_POINT('Ctrl Pts',(-1.58744937489796,-1.,0.939646377909319));
#32987=CARTESIAN_POINT('Ctrl Pts',(-1.58744937489796,1.,0.939646377909319));
#32988=CARTESIAN_POINT('Ctrl Pts',(-1.59810042045408,-1.,0.946078063325796));
#32989=CARTESIAN_POINT('Ctrl Pts',(-1.59810042045408,1.,0.946078063325796));
#32990=CARTESIAN_POINT('Ctrl Pts',(-1.60706069897794,-1.,0.951613284361248));
#32991=CARTESIAN_POINT('Ctrl Pts',(-1.60706069897794,1.,0.951613284361248));
#32992=CARTESIAN_POINT('Ctrl Pts',(-1.61449324337233,-1.,0.956354422921573));
#32993=CARTESIAN_POINT('Ctrl Pts',(-1.61449324337233,1.,0.956354422921573));
#32994=CARTESIAN_POINT('Ctrl Pts',(-1.62061638139929,-1.,0.960438326099958));
#32995=CARTESIAN_POINT('Ctrl Pts',(-1.62061638139929,1.,0.960438326099958));
#32996=CARTESIAN_POINT('Ctrl Pts',(-1.6257193066974,-1.,0.964046107037821));
#32997=CARTESIAN_POINT('Ctrl Pts',(-1.6257193066974,1.,0.964046107037821));
#32998=CARTESIAN_POINT('Ctrl Pts',(-1.63013849959083,-1.,0.967387853228041));
#32999=CARTESIAN_POINT('Ctrl Pts',(-1.63013849959083,1.,0.967387853228041));
#33000=CARTESIAN_POINT('Ctrl Pts',(-1.63420665729609,-1.,0.970669715996356));
#33001=CARTESIAN_POINT('Ctrl Pts',(-1.63420665729609,1.,0.970669715996356));
#33002=CARTESIAN_POINT('Ctrl Pts',(-1.63820952658157,-1.,0.974066058287501));
#33003=CARTESIAN_POINT('Ctrl Pts',(-1.63820952658157,1.,0.974066058287501));
#33004=CARTESIAN_POINT('Ctrl Pts',(-1.64233990826831,-1.,0.977689794120297));
#33005=CARTESIAN_POINT('Ctrl Pts',(-1.64233990826831,1.,0.977689794120297));
#33006=CARTESIAN_POINT('Ctrl Pts',(-1.64665139190834,-1.,0.981562530940574));
#33007=CARTESIAN_POINT('Ctrl Pts',(-1.64665139190834,1.,0.981562530940574));
#33008=CARTESIAN_POINT('Ctrl Pts',(-1.6511001661277,-1.,0.985642622921626));
#33009=CARTESIAN_POINT('Ctrl Pts',(-1.6511001661277,1.,0.985642622921626));
#33010=CARTESIAN_POINT('Ctrl Pts',(-1.65559044289746,-1.,0.98985562785445));
#33011=CARTESIAN_POINT('Ctrl Pts',(-1.65559044289746,1.,0.98985562785445));
#33012=CARTESIAN_POINT('Ctrl Pts',(-1.66001553809916,-1.,0.994121836661116));
#33013=CARTESIAN_POINT('Ctrl Pts',(-1.66001553809916,1.,0.994121836661116));
#33014=CARTESIAN_POINT('Ctrl Pts',(-1.66430758030304,-1.,0.998389654952317));
#33015=CARTESIAN_POINT('Ctrl Pts',(-1.66430758030304,1.,0.998389654952317));
#33016=CARTESIAN_POINT('Ctrl Pts',(-1.66846059277231,-1.,1.00265091003682));
#33017=CARTESIAN_POINT('Ctrl Pts',(-1.66846059277231,1.,1.00265091003682));
#33018=CARTESIAN_POINT('Ctrl Pts',(-1.67250335383248,-1.,1.00692206696387));
#33019=CARTESIAN_POINT('Ctrl Pts',(-1.67250335383248,1.,1.00692206696387));
#33020=CARTESIAN_POINT('Ctrl Pts',(-1.67648246776457,-1.,1.01123236493507));
#33021=CARTESIAN_POINT('Ctrl Pts',(-1.67648246776457,1.,1.01123236493507));
#33022=CARTESIAN_POINT('Ctrl Pts',(-1.6804428989482,-1.,1.01561026162787));
#33023=CARTESIAN_POINT('Ctrl Pts',(-1.6804428989482,1.,1.01561026162787));
#33024=CARTESIAN_POINT('Ctrl Pts',(-1.68440578021739,-1.,1.02006795074222));
#33025=CARTESIAN_POINT('Ctrl Pts',(-1.68440578021739,1.,1.02006795074222));
#33026=CARTESIAN_POINT('Ctrl Pts',(-1.68836910178475,-1.,1.02460180535272));
#33027=CARTESIAN_POINT('Ctrl Pts',(-1.68836910178475,1.,1.02460180535272));
#33028=CARTESIAN_POINT('Ctrl Pts',(-1.69231840863471,-1.,1.02919977579155));
#33029=CARTESIAN_POINT('Ctrl Pts',(-1.69231840863471,1.,1.02919977579155));
#33030=CARTESIAN_POINT('Ctrl Pts',(-1.69623414782769,-1.,1.03384646003587));
#33031=CARTESIAN_POINT('Ctrl Pts',(-1.69623414782769,1.,1.03384646003587));
#33032=CARTESIAN_POINT('Ctrl Pts',(-1.70010052930951,-1.,1.03852922490782));
#33033=CARTESIAN_POINT('Ctrl Pts',(-1.70010052930951,1.,1.03852922490782));
#33034=CARTESIAN_POINT('Ctrl Pts',(-1.70391338707969,-1.,1.04324363334546));
#33035=CARTESIAN_POINT('Ctrl Pts',(-1.70391338707969,1.,1.04324363334546));
#33036=CARTESIAN_POINT('Ctrl Pts',(-1.70767646263641,-1.,1.0479908540499));
#33037=CARTESIAN_POINT('Ctrl Pts',(-1.70767646263641,1.,1.0479908540499));
#33038=CARTESIAN_POINT('Ctrl Pts',(-1.71139783543986,-1.,1.05277517202854));
#33039=CARTESIAN_POINT('Ctrl Pts',(-1.71139783543986,1.,1.05277517202854));
#33040=CARTESIAN_POINT('Ctrl Pts',(-1.71508654427022,-1.,1.05760163192481));
#33041=CARTESIAN_POINT('Ctrl Pts',(-1.71508654427022,1.,1.05760163192481));
#33042=CARTESIAN_POINT('Ctrl Pts',(-1.71874858456908,-1.,1.0624732468065));
#33043=CARTESIAN_POINT('Ctrl Pts',(-1.71874858456908,1.,1.0624732468065));
#33044=CARTESIAN_POINT('Ctrl Pts',(-1.72238500928456,-1.,1.06738966975463));
#33045=CARTESIAN_POINT('Ctrl Pts',(-1.72238500928456,1.,1.06738966975463));
#33046=CARTESIAN_POINT('Ctrl Pts',(-1.72599406198489,-1.,1.07234866990252));
#33047=CARTESIAN_POINT('Ctrl Pts',(-1.72599406198489,1.,1.07234866990252));
#33048=CARTESIAN_POINT('Ctrl Pts',(-1.72957248977424,-1.,1.0773470373727));
#33049=CARTESIAN_POINT('Ctrl Pts',(-1.72957248977424,1.,1.0773470373727));
#33050=CARTESIAN_POINT('Ctrl Pts',(-1.73311705663407,-1.,1.08238162784749));
#33051=CARTESIAN_POINT('Ctrl Pts',(-1.73311705663407,1.,1.08238162784749));
#33052=CARTESIAN_POINT('Ctrl Pts',(-1.73662628326093,-1.,1.08745056285429));
#33053=CARTESIAN_POINT('Ctrl Pts',(-1.73662628326093,1.,1.08745056285429));
#33054=CARTESIAN_POINT('Ctrl Pts',(-1.74010053962252,-1.,1.09255329056496));
#33055=CARTESIAN_POINT('Ctrl Pts',(-1.74010053962252,1.,1.09255329056496));
#33056=CARTESIAN_POINT('Ctrl Pts',(-1.74354119236212,-1.,1.09768999241229));
#33057=CARTESIAN_POINT('Ctrl Pts',(-1.74354119236212,1.,1.09768999241229));
#33058=CARTESIAN_POINT('Ctrl Pts',(-1.74695004214924,-1.,1.10286118991144));
#33059=CARTESIAN_POINT('Ctrl Pts',(-1.74695004214924,1.,1.10286118991144));
#33060=CARTESIAN_POINT('Ctrl Pts',(-1.75032866075914,-1.,1.10806728183003));
#33061=CARTESIAN_POINT('Ctrl Pts',(-1.75032866075914,1.,1.10806728183003));
#33062=CARTESIAN_POINT('Ctrl Pts',(-1.75367772094617,-1.,1.11330807582542));
#33063=CARTESIAN_POINT('Ctrl Pts',(-1.75367772094617,1.,1.11330807582542));
#33064=CARTESIAN_POINT('Ctrl Pts',(-1.75699720772089,-1.,1.11858293216752));
#33065=CARTESIAN_POINT('Ctrl Pts',(-1.75699720772089,1.,1.11858293216752));
#33066=CARTESIAN_POINT('Ctrl Pts',(-1.76028671825084,-1.,1.12389096855078));
#33067=CARTESIAN_POINT('Ctrl Pts',(-1.76028671825084,1.,1.12389096855078));
#33068=CARTESIAN_POINT('Ctrl Pts',(-1.76354571966171,-1.,1.12923123555076));
#33069=CARTESIAN_POINT('Ctrl Pts',(-1.76354571966171,1.,1.12923123555076));
#33070=CARTESIAN_POINT('Ctrl Pts',(-1.76677384551883,-1.,1.13460291804635));
#33071=CARTESIAN_POINT('Ctrl Pts',(-1.76677384551883,1.,1.13460291804635));
#33072=CARTESIAN_POINT('Ctrl Pts',(-1.76997111386806,-1.,1.14000548337));
#33073=CARTESIAN_POINT('Ctrl Pts',(-1.76997111386806,1.,1.14000548337));
#33074=CARTESIAN_POINT('Ctrl Pts',(-1.77313777896234,-1.,1.14543858226948));
#33075=CARTESIAN_POINT('Ctrl Pts',(-1.77313777896234,1.,1.14543858226948));
#33076=CARTESIAN_POINT('Ctrl Pts',(-1.77627422557034,-1.,1.15090197841531));
#33077=CARTESIAN_POINT('Ctrl Pts',(-1.77627422557034,1.,1.15090197841531));
#33078=CARTESIAN_POINT('Ctrl Pts',(-1.77938085564261,-1.,1.15639547194689));
#33079=CARTESIAN_POINT('Ctrl Pts',(-1.77938085564261,1.,1.15639547194689));
#33080=CARTESIAN_POINT('Ctrl Pts',(-1.78245795880949,-1.,1.16191881298458));
#33081=CARTESIAN_POINT('Ctrl Pts',(-1.78245795880949,1.,1.16191881298458));
#33082=CARTESIAN_POINT('Ctrl Pts',(-1.78550566040349,-1.,1.16747166312239));
#33083=CARTESIAN_POINT('Ctrl Pts',(-1.78550566040349,1.,1.16747166312239));
#33084=CARTESIAN_POINT('Ctrl Pts',(-1.78852398877523,-1.,1.17305363177265));
#33085=CARTESIAN_POINT('Ctrl Pts',(-1.78852398877523,1.,1.17305363177265));
#33086=CARTESIAN_POINT('Ctrl Pts',(-1.79151291552646,-1.,1.17866429440781));
#33087=CARTESIAN_POINT('Ctrl Pts',(-1.79151291552646,1.,1.17866429440781));
#33088=CARTESIAN_POINT('Ctrl Pts',(-1.79447240321572,-1.,1.18430321697471));
#33089=CARTESIAN_POINT('Ctrl Pts',(-1.79447240321572,1.,1.18430321697471));
#33090=CARTESIAN_POINT('Ctrl Pts',(-1.79740245923649,-1.,1.1899699793456));
#33091=CARTESIAN_POINT('Ctrl Pts',(-1.79740245923649,1.,1.1899699793456));
#33092=CARTESIAN_POINT('Ctrl Pts',(-1.80030314370121,-1.,1.19566418930405));
#33093=CARTESIAN_POINT('Ctrl Pts',(-1.80030314370121,1.,1.19566418930405));
#33094=CARTESIAN_POINT('Ctrl Pts',(-1.8031745483882,-1.,1.2013854893912));
#33095=CARTESIAN_POINT('Ctrl Pts',(-1.8031745483882,1.,1.2013854893912));
#33096=CARTESIAN_POINT('Ctrl Pts',(-1.80601678480772,-1.,1.20713356605519));
#33097=CARTESIAN_POINT('Ctrl Pts',(-1.80601678480772,1.,1.20713356605519));
#33098=CARTESIAN_POINT('Ctrl Pts',(-1.80882996916931,-1.,1.2129081570818));
#33099=CARTESIAN_POINT('Ctrl Pts',(-1.80882996916931,1.,1.2129081570818));
#33100=CARTESIAN_POINT('Ctrl Pts',(-1.81161420806172,-1.,1.2187090610323));
#33101=CARTESIAN_POINT('Ctrl Pts',(-1.81161420806172,1.,1.2187090610323));
#33102=CARTESIAN_POINT('Ctrl Pts',(-1.81436959209778,-1.,1.22453613304507));
#33103=CARTESIAN_POINT('Ctrl Pts',(-1.81436959209778,1.,1.22453613304507));
#33104=CARTESIAN_POINT('Ctrl Pts',(-1.81655087183054,-1.,1.22921864890975));
#33105=CARTESIAN_POINT('Ctrl Pts',(-1.81655087183054,1.,1.22921864890975));
#33106=CARTESIAN_POINT('Ctrl Pts',(-1.81817389920914,-1.,1.23274224526804));
#33107=CARTESIAN_POINT('Ctrl Pts',(-1.81817389920914,1.,1.23274224526804));
#33108=CARTESIAN_POINT('Ctrl Pts',(-1.81925017193531,-1.,1.23509651170384));
#33109=CARTESIAN_POINT('Ctrl Pts',(-1.81925017193531,1.,1.23509651170384));
#33110=CARTESIAN_POINT('Ctrl Pts',(-1.81978687191668,-1.,1.23627494547115));
#33111=CARTESIAN_POINT('Ctrl Pts',(-1.81978687191668,1.,1.23627494547115));
#33112=CARTESIAN_POINT('',(-1.5055822144029,1.,0.892032620296855));
#33113=CARTESIAN_POINT('Ctrl Pts',(-1.5055822144029,1.,0.892032620296855));
#33114=CARTESIAN_POINT('Ctrl Pts',(-1.50980486807181,1.,0.894452006967538));
#33115=CARTESIAN_POINT('Ctrl Pts',(-1.51805569591479,1.,0.89918504749193));
#33116=CARTESIAN_POINT('Ctrl Pts',(-1.52984849890434,1.,0.905967409640499));
#33117=CARTESIAN_POINT('Ctrl Pts',(-1.54440491152808,1.,0.91437591904658));
#33118=CARTESIAN_POINT('Ctrl Pts',(-1.56065988582509,1.,0.923832188966322));
#33119=CARTESIAN_POINT('Ctrl Pts',(-1.57499388385561,1.,0.932246680128849));
#33120=CARTESIAN_POINT('Ctrl Pts',(-1.58744937489796,1.,0.939646377909319));
#33121=CARTESIAN_POINT('Ctrl Pts',(-1.59810042045408,1.,0.946078063325796));
#33122=CARTESIAN_POINT('Ctrl Pts',(-1.60706069897794,1.,0.951613284361248));
#33123=CARTESIAN_POINT('Ctrl Pts',(-1.61449324337233,1.,0.956354422921573));
#33124=CARTESIAN_POINT('Ctrl Pts',(-1.62061638139929,1.,0.960438326099958));
#33125=CARTESIAN_POINT('Ctrl Pts',(-1.6257193066974,1.,0.964046107037821));
#33126=CARTESIAN_POINT('Ctrl Pts',(-1.63013849959083,1.,0.967387853228041));
#33127=CARTESIAN_POINT('Ctrl Pts',(-1.63420665729609,1.,0.970669715996356));
#33128=CARTESIAN_POINT('Ctrl Pts',(-1.63820952658157,1.,0.974066058287501));
#33129=CARTESIAN_POINT('Ctrl Pts',(-1.64233990826831,1.,0.977689794120297));
#33130=CARTESIAN_POINT('Ctrl Pts',(-1.64665139190834,1.,0.981562530940574));
#33131=CARTESIAN_POINT('Ctrl Pts',(-1.6511001661277,1.,0.985642622921626));
#33132=CARTESIAN_POINT('Ctrl Pts',(-1.65559044289746,1.,0.98985562785445));
#33133=CARTESIAN_POINT('Ctrl Pts',(-1.66001553809916,1.,0.994121836661116));
#33134=CARTESIAN_POINT('Ctrl Pts',(-1.66430758030304,1.,0.998389654952317));
#33135=CARTESIAN_POINT('Ctrl Pts',(-1.66846059277231,1.,1.00265091003682));
#33136=CARTESIAN_POINT('Ctrl Pts',(-1.67250335383248,1.,1.00692206696387));
#33137=CARTESIAN_POINT('Ctrl Pts',(-1.67648246776457,1.,1.01123236493507));
#33138=CARTESIAN_POINT('Ctrl Pts',(-1.6804428989482,1.,1.01561026162787));
#33139=CARTESIAN_POINT('Ctrl Pts',(-1.68440578021739,1.,1.02006795074222));
#33140=CARTESIAN_POINT('Ctrl Pts',(-1.68836910178475,1.,1.02460180535272));
#33141=CARTESIAN_POINT('Ctrl Pts',(-1.69231840863471,1.,1.02919977579155));
#33142=CARTESIAN_POINT('Ctrl Pts',(-1.69623414782769,1.,1.03384646003587));
#33143=CARTESIAN_POINT('Ctrl Pts',(-1.70010052930951,1.,1.03852922490782));
#33144=CARTESIAN_POINT('Ctrl Pts',(-1.70391338707969,1.,1.04324363334546));
#33145=CARTESIAN_POINT('Ctrl Pts',(-1.70767646263641,1.,1.0479908540499));
#33146=CARTESIAN_POINT('Ctrl Pts',(-1.71139783543986,1.,1.05277517202854));
#33147=CARTESIAN_POINT('Ctrl Pts',(-1.71508654427022,1.,1.05760163192481));
#33148=CARTESIAN_POINT('Ctrl Pts',(-1.71874858456908,1.,1.0624732468065));
#33149=CARTESIAN_POINT('Ctrl Pts',(-1.72238500928456,1.,1.06738966975463));
#33150=CARTESIAN_POINT('Ctrl Pts',(-1.72599406198489,1.,1.07234866990252));
#33151=CARTESIAN_POINT('Ctrl Pts',(-1.72957248977424,1.,1.0773470373727));
#33152=CARTESIAN_POINT('Ctrl Pts',(-1.73311705663407,1.,1.08238162784749));
#33153=CARTESIAN_POINT('Ctrl Pts',(-1.73662628326093,1.,1.08745056285429));
#33154=CARTESIAN_POINT('Ctrl Pts',(-1.74010053962252,1.,1.09255329056496));
#33155=CARTESIAN_POINT('Ctrl Pts',(-1.74354119236212,1.,1.09768999241229));
#33156=CARTESIAN_POINT('Ctrl Pts',(-1.74695004214924,1.,1.10286118991144));
#33157=CARTESIAN_POINT('Ctrl Pts',(-1.75032866075914,1.,1.10806728183003));
#33158=CARTESIAN_POINT('Ctrl Pts',(-1.75367772094617,1.,1.11330807582542));
#33159=CARTESIAN_POINT('Ctrl Pts',(-1.75699720772089,1.,1.11858293216752));
#33160=CARTESIAN_POINT('Ctrl Pts',(-1.76028671825084,1.,1.12389096855078));
#33161=CARTESIAN_POINT('Ctrl Pts',(-1.76354571966171,1.,1.12923123555076));
#33162=CARTESIAN_POINT('Ctrl Pts',(-1.76677384551883,1.,1.13460291804635));
#33163=CARTESIAN_POINT('Ctrl Pts',(-1.76997111386806,1.,1.14000548337));
#33164=CARTESIAN_POINT('Ctrl Pts',(-1.77313777896234,1.,1.14543858226948));
#33165=CARTESIAN_POINT('Ctrl Pts',(-1.77627422557034,1.,1.15090197841531));
#33166=CARTESIAN_POINT('Ctrl Pts',(-1.77938085564261,1.,1.15639547194689));
#33167=CARTESIAN_POINT('Ctrl Pts',(-1.78245795880949,1.,1.16191881298458));
#33168=CARTESIAN_POINT('Ctrl Pts',(-1.78550566040349,1.,1.16747166312239));
#33169=CARTESIAN_POINT('Ctrl Pts',(-1.78852398877523,1.,1.17305363177265));
#33170=CARTESIAN_POINT('Ctrl Pts',(-1.79151291552646,1.,1.17866429440781));
#33171=CARTESIAN_POINT('Ctrl Pts',(-1.79447240321572,1.,1.18430321697471));
#33172=CARTESIAN_POINT('Ctrl Pts',(-1.79740245923649,1.,1.1899699793456));
#33173=CARTESIAN_POINT('Ctrl Pts',(-1.80030314370121,1.,1.19566418930405));
#33174=CARTESIAN_POINT('Ctrl Pts',(-1.8031745483882,1.,1.2013854893912));
#33175=CARTESIAN_POINT('Ctrl Pts',(-1.80601678480772,1.,1.20713356605519));
#33176=CARTESIAN_POINT('Ctrl Pts',(-1.80882996916931,1.,1.2129081570818));
#33177=CARTESIAN_POINT('Ctrl Pts',(-1.81161420806172,1.,1.2187090610323));
#33178=CARTESIAN_POINT('Ctrl Pts',(-1.81436959209778,1.,1.22453613304507));
#33179=CARTESIAN_POINT('Ctrl Pts',(-1.81655087183054,1.,1.22921864890975));
#33180=CARTESIAN_POINT('Ctrl Pts',(-1.81817389920914,1.,1.23274224526804));
#33181=CARTESIAN_POINT('Ctrl Pts',(-1.81925017193531,1.,1.23509651170384));
#33182=CARTESIAN_POINT('Ctrl Pts',(-1.81978687191668,1.,1.23627494547115));
#33183=CARTESIAN_POINT('',(-1.5055822144029,0.,0.892032620296856));
#33184=CARTESIAN_POINT('Origin',(0.,0.,0.));
#33185=CARTESIAN_POINT('',(-1.60662857109684,1.,0.693717979106305));
#33186=CARTESIAN_POINT('Origin',(0.,1.,0.));
#33187=CARTESIAN_POINT('',(-1.60662857109684,0.,0.693717979106306));
#33188=CARTESIAN_POINT('Ctrl Pts',(-2.0698113262342,-1.,0.7455743247944));
#33189=CARTESIAN_POINT('Ctrl Pts',(-2.0698113262342,1.,0.7455743247944));
#33190=CARTESIAN_POINT('Ctrl Pts',(-2.06854248895728,-1.,0.745832791378367));
#33191=CARTESIAN_POINT('Ctrl Pts',(-2.06854248895728,1.,0.745832791378367));
#33192=CARTESIAN_POINT('Ctrl Pts',(-2.06600523016815,-1.,0.7463458715442));
#33193=CARTESIAN_POINT('Ctrl Pts',(-2.06600523016815,1.,0.7463458715442));
#33194=CARTESIAN_POINT('Ctrl Pts',(-2.06220058927826,-1.,0.747103932787919));
#33195=CARTESIAN_POINT('Ctrl Pts',(-2.06220058927826,1.,0.747103932787919));
#33196=CARTESIAN_POINT('Ctrl Pts',(-2.05713023031006,-1.,0.748091554183802));
#33197=CARTESIAN_POINT('Ctrl Pts',(-2.05713023031006,1.,0.748091554183802));
#33198=CARTESIAN_POINT('Ctrl Pts',(-2.05079645592154,-1.,0.749287468665046));
#33199=CARTESIAN_POINT('Ctrl Pts',(-2.05079645592154,1.,0.749287468665046));
#33200=CARTESIAN_POINT('Ctrl Pts',(-2.04446689147979,-1.,0.750444657875576));
#33201=CARTESIAN_POINT('Ctrl Pts',(-2.04446689147979,1.,0.750444657875576));
#33202=CARTESIAN_POINT('Ctrl Pts',(-2.03814160092099,-1.,0.751562963361115));
#33203=CARTESIAN_POINT('Ctrl Pts',(-2.03814160092099,1.,0.751562963361115));
#33204=CARTESIAN_POINT('Ctrl Pts',(-2.03182068456221,-1.,0.752642180487211));
#33205=CARTESIAN_POINT('Ctrl Pts',(-2.03182068456221,1.,0.752642180487211));
#33206=CARTESIAN_POINT('Ctrl Pts',(-2.02550428623313,-1.,0.753682061112768));
#33207=CARTESIAN_POINT('Ctrl Pts',(-2.02550428623313,1.,0.753682061112768));
#33208=CARTESIAN_POINT('Ctrl Pts',(-2.01919259405809,-1.,0.754682330722816));
#33209=CARTESIAN_POINT('Ctrl Pts',(-2.01919259405809,1.,0.754682330722816));
#33210=CARTESIAN_POINT('Ctrl Pts',(-2.01288584328084,-1.,0.755642704957865));
#33211=CARTESIAN_POINT('Ctrl Pts',(-2.01288584328084,1.,0.755642704957865));
#33212=CARTESIAN_POINT('Ctrl Pts',(-2.0065843158773,-1.,0.75656290464667));
#33213=CARTESIAN_POINT('Ctrl Pts',(-2.0065843158773,1.,0.75656290464667));
#33214=CARTESIAN_POINT('Ctrl Pts',(-2.00028834739178,-1.,0.757442676862724));
#33215=CARTESIAN_POINT('Ctrl Pts',(-2.00028834739178,1.,0.757442676862724));
#33216=CARTESIAN_POINT('Ctrl Pts',(-1.99399831098817,-1.,0.758281796766761));
#33217=CARTESIAN_POINT('Ctrl Pts',(-1.99399831098817,1.,0.758281796766761));
#33218=CARTESIAN_POINT('Ctrl Pts',(-1.98771456680874,-1.,0.759080037802488));
#33219=CARTESIAN_POINT('Ctrl Pts',(-1.98771456680874,1.,0.759080037802488));
#33220=CARTESIAN_POINT('Ctrl Pts',(-1.98143741418172,-1.,0.75983714745219));
#33221=CARTESIAN_POINT('Ctrl Pts',(-1.98143741418172,1.,0.75983714745219));
#33222=CARTESIAN_POINT('Ctrl Pts',(-1.97516705321494,-1.,0.760552825409757));
#33223=CARTESIAN_POINT('Ctrl Pts',(-1.97516705321494,1.,0.760552825409757));
#33224=CARTESIAN_POINT('Ctrl Pts',(-1.96890351582499,-1.,0.76122669048382));
#33225=CARTESIAN_POINT('Ctrl Pts',(-1.96890351582499,1.,0.76122669048382));
#33226=CARTESIAN_POINT('Ctrl Pts',(-1.96264672744186,-1.,0.761858300014423));
#33227=CARTESIAN_POINT('Ctrl Pts',(-1.96264672744186,1.,0.761858300014423));
#33228=CARTESIAN_POINT('Ctrl Pts',(-1.95639665309869,-1.,0.762447203806179));
#33229=CARTESIAN_POINT('Ctrl Pts',(-1.95639665309869,1.,0.762447203806179));
#33230=CARTESIAN_POINT('Ctrl Pts',(-1.95015342590024,-1.,0.762992990878769));
#33231=CARTESIAN_POINT('Ctrl Pts',(-1.95015342590024,1.,0.762992990878769));
#33232=CARTESIAN_POINT('Ctrl Pts',(-1.9439174661764,-1.,0.763495333538629));
#33233=CARTESIAN_POINT('Ctrl Pts',(-1.9439174661764,1.,0.763495333538629));
#33234=CARTESIAN_POINT('Ctrl Pts',(-1.93768964875886,-1.,0.763954049121458));
#33235=CARTESIAN_POINT('Ctrl Pts',(-1.93768964875886,1.,0.763954049121458));
#33236=CARTESIAN_POINT('Ctrl Pts',(-1.93147105496382,-1.,0.76436901067394));
#33237=CARTESIAN_POINT('Ctrl Pts',(-1.93147105496382,1.,0.76436901067394));
#33238=CARTESIAN_POINT('Ctrl Pts',(-1.92526263537048,-1.,0.764740025488211));
#33239=CARTESIAN_POINT('Ctrl Pts',(-1.92526263537048,1.,0.764740025488211));
#33240=CARTESIAN_POINT('Ctrl Pts',(-1.91906491634196,-1.,0.765066729667088));
#33241=CARTESIAN_POINT('Ctrl Pts',(-1.91906491634196,1.,0.765066729667088));
#33242=CARTESIAN_POINT('Ctrl Pts',(-1.91287765805169,-1.,0.765348465884722));
#33243=CARTESIAN_POINT('Ctrl Pts',(-1.91287765805169,1.,0.765348465884722));
#33244=CARTESIAN_POINT('Ctrl Pts',(-1.90669961402356,-1.,0.765584196937919));
#33245=CARTESIAN_POINT('Ctrl Pts',(-1.90669961402356,1.,0.765584196937919));
#33246=CARTESIAN_POINT('Ctrl Pts',(-1.90052930393596,-1.,0.765772772593386));
#33247=CARTESIAN_POINT('Ctrl Pts',(-1.90052930393596,1.,0.765772772593386));
#33248=CARTESIAN_POINT('Ctrl Pts',(-1.89436577771388,-1.,0.765913193856978));
#33249=CARTESIAN_POINT('Ctrl Pts',(-1.89436577771388,1.,0.765913193856978));
#33250=CARTESIAN_POINT('Ctrl Pts',(-1.88820926433409,-1.,0.766004837062091));
#33251=CARTESIAN_POINT('Ctrl Pts',(-1.88820926433409,1.,0.766004837062091));
#33252=CARTESIAN_POINT('Ctrl Pts',(-1.88206215302561,-1.,0.766047794851864));
#33253=CARTESIAN_POINT('Ctrl Pts',(-1.88206215302561,1.,0.766047794851864));
#33254=CARTESIAN_POINT('Ctrl Pts',(-1.87592888967883,-1.,0.766042837036744));
#33255=CARTESIAN_POINT('Ctrl Pts',(-1.87592888967883,1.,0.766042837036744));
#33256=CARTESIAN_POINT('Ctrl Pts',(-1.86981398314341,-1.,0.765990708546091));
#33257=CARTESIAN_POINT('Ctrl Pts',(-1.86981398314341,1.,0.765990708546091));
#33258=CARTESIAN_POINT('Ctrl Pts',(-1.86372027063312,-1.,0.765891519092547));
#33259=CARTESIAN_POINT('Ctrl Pts',(-1.86372027063312,1.,0.765891519092547));
#33260=CARTESIAN_POINT('Ctrl Pts',(-1.85764741390394,-1.,0.765744212909318));
#33261=CARTESIAN_POINT('Ctrl Pts',(-1.85764741390394,1.,0.765744212909318));
#33262=CARTESIAN_POINT('Ctrl Pts',(-1.85158945130063,-1.,0.765545710619062));
#33263=CARTESIAN_POINT('Ctrl Pts',(-1.85158945130063,1.,0.765545710619062));
#33264=CARTESIAN_POINT('Ctrl Pts',(-1.84553698875924,-1.,0.765291664862029));
#33265=CARTESIAN_POINT('Ctrl Pts',(-1.84553698875924,1.,0.765291664862029));
#33266=CARTESIAN_POINT('Ctrl Pts',(-1.83948181064835,-1.,0.764978057881737));
#33267=CARTESIAN_POINT('Ctrl Pts',(-1.83948181064835,1.,0.764978057881737));
#33268=CARTESIAN_POINT('Ctrl Pts',(-1.83342077227142,-1.,0.764602549687853));
#33269=CARTESIAN_POINT('Ctrl Pts',(-1.83342077227142,1.,0.764602549687853));
#33270=CARTESIAN_POINT('Ctrl Pts',(-1.82735991200065,-1.,0.764165902605995));
#33271=CARTESIAN_POINT('Ctrl Pts',(-1.82735991200065,1.,0.764165902605995));
#33272=CARTESIAN_POINT('Ctrl Pts',(-1.82131873145266,-1.,0.763673465462726));
#33273=CARTESIAN_POINT('Ctrl Pts',(-1.82131873145266,1.,0.763673465462726));
#33274=CARTESIAN_POINT('Ctrl Pts',(-1.8153211840553,-1.,0.763132003836634));
#33275=CARTESIAN_POINT('Ctrl Pts',(-1.8153211840553,1.,0.763132003836634));
#33276=CARTESIAN_POINT('Ctrl Pts',(-1.80938551463965,-1.,0.762546129463938));
#33277=CARTESIAN_POINT('Ctrl Pts',(-1.80938551463965,1.,0.762546129463938));
#33278=CARTESIAN_POINT('Ctrl Pts',(-1.80351583877342,-1.,0.761915336443547));
#33279=CARTESIAN_POINT('Ctrl Pts',(-1.80351583877342,1.,0.761915336443547));
#33280=CARTESIAN_POINT('Ctrl Pts',(-1.79768986997783,-1.,0.761229695230558));
#33281=CARTESIAN_POINT('Ctrl Pts',(-1.79768986997783,1.,0.761229695230558));
#33282=CARTESIAN_POINT('Ctrl Pts',(-1.7918581561088,-1.,0.760469555880749));
#33283=CARTESIAN_POINT('Ctrl Pts',(-1.7918581561088,1.,0.760469555880749));
#33284=CARTESIAN_POINT('Ctrl Pts',(-1.78596964884604,-1.,0.759614401110189));
#33285=CARTESIAN_POINT('Ctrl Pts',(-1.78596964884604,1.,0.759614401110189));
#33286=CARTESIAN_POINT('Ctrl Pts',(-1.77999411220945,-1.,0.758650626677518));
#33287=CARTESIAN_POINT('Ctrl Pts',(-1.77999411220945,1.,0.758650626677518));
#33288=CARTESIAN_POINT('Ctrl Pts',(-1.77394167108292,-1.,0.757578264077029));
#33289=CARTESIAN_POINT('Ctrl Pts',(-1.77394167108292,1.,0.757578264077029));
#33290=CARTESIAN_POINT('Ctrl Pts',(-1.76789396002998,-1.,0.75642189602781));
#33291=CARTESIAN_POINT('Ctrl Pts',(-1.76789396002998,1.,0.75642189602781));
#33292=CARTESIAN_POINT('Ctrl Pts',(-1.76197817240128,-1.,0.755220979974461));
#33293=CARTESIAN_POINT('Ctrl Pts',(-1.76197817240128,1.,0.755220979974461));
#33294=CARTESIAN_POINT('Ctrl Pts',(-1.75631083600019,-1.,0.754009254027829));
#33295=CARTESIAN_POINT('Ctrl Pts',(-1.75631083600019,1.,0.754009254027829));
#33296=CARTESIAN_POINT('Ctrl Pts',(-1.75095139468794,-1.,0.752797683531314));
#33297=CARTESIAN_POINT('Ctrl Pts',(-1.75095139468794,1.,0.752797683531314));
#33298=CARTESIAN_POINT('Ctrl Pts',(-1.74585086852502,-1.,0.751555614164482));
#33299=CARTESIAN_POINT('Ctrl Pts',(-1.74585086852502,1.,0.751555614164482));
#33300=CARTESIAN_POINT('Ctrl Pts',(-1.74080458267114,-1.,0.750193435981249));
#33301=CARTESIAN_POINT('Ctrl Pts',(-1.74080458267114,1.,0.750193435981249));
#33302=CARTESIAN_POINT('Ctrl Pts',(-1.7355035168033,-1.,0.74858246295687));
#33303=CARTESIAN_POINT('Ctrl Pts',(-1.7355035168033,1.,0.74858246295687));
#33304=CARTESIAN_POINT('Ctrl Pts',(-1.72958533647714,-1.,0.746574710097752));
#33305=CARTESIAN_POINT('Ctrl Pts',(-1.72958533647714,1.,0.746574710097752));
#33306=CARTESIAN_POINT('Ctrl Pts',(-1.72268229916769,-1.,0.744021445433093));
#33307=CARTESIAN_POINT('Ctrl Pts',(-1.72268229916769,1.,0.744021445433093));
#33308=CARTESIAN_POINT('Ctrl Pts',(-1.71447789751001,-1.,0.74079516202821));
#33309=CARTESIAN_POINT('Ctrl Pts',(-1.71447789751001,1.,0.74079516202821));
#33310=CARTESIAN_POINT('Ctrl Pts',(-1.70473309004249,-1.,0.736799665716932));
#33311=CARTESIAN_POINT('Ctrl Pts',(-1.70473309004249,1.,0.736799665716932));
#33312=CARTESIAN_POINT('Ctrl Pts',(-1.69326921972915,-1.,0.731963238685357));
#33313=CARTESIAN_POINT('Ctrl Pts',(-1.69326921972915,1.,0.731963238685357));
#33314=CARTESIAN_POINT('Ctrl Pts',(-1.67996158451922,-1.,0.726235967982445));
#33315=CARTESIAN_POINT('Ctrl Pts',(-1.67996158451922,1.,0.726235967982445));
#33316=CARTESIAN_POINT('Ctrl Pts',(-1.66472880551777,-1.,0.71958543378795));
#33317=CARTESIAN_POINT('Ctrl Pts',(-1.66472880551777,1.,0.71958543378795));
#33318=CARTESIAN_POINT('Ctrl Pts',(-1.64752408828442,-1.,0.711993139340447));
#33319=CARTESIAN_POINT('Ctrl Pts',(-1.64752408828442,1.,0.711993139340447));
#33320=CARTESIAN_POINT('Ctrl Pts',(-1.6321654166204,-1.,0.705159151977294));
#33321=CARTESIAN_POINT('Ctrl Pts',(-1.6321654166204,1.,0.705159151977294));
#33322=CARTESIAN_POINT('Ctrl Pts',(-1.61974673471117,-1.,0.699605146398837));
#33323=CARTESIAN_POINT('Ctrl Pts',(-1.61974673471117,1.,0.699605146398837));
#33324=CARTESIAN_POINT('Ctrl Pts',(-1.61106790957619,-1.,0.69571209787897));
#33325=CARTESIAN_POINT('Ctrl Pts',(-1.61106790957619,1.,0.69571209787897));
#33326=CARTESIAN_POINT('Ctrl Pts',(-1.60662857109684,-1.,0.693717979106305));
#33327=CARTESIAN_POINT('Ctrl Pts',(-1.60662857109684,1.,0.693717979106305));
#33328=CARTESIAN_POINT('',(-2.0698113262342,1.,0.7455743247944));
#33329=CARTESIAN_POINT('Ctrl Pts',(-2.0698113262342,1.,0.7455743247944));
#33330=CARTESIAN_POINT('Ctrl Pts',(-2.06854248895728,1.,0.745832791378367));
#33331=CARTESIAN_POINT('Ctrl Pts',(-2.06600523016815,1.,0.7463458715442));
#33332=CARTESIAN_POINT('Ctrl Pts',(-2.06220058927826,1.,0.747103932787919));
#33333=CARTESIAN_POINT('Ctrl Pts',(-2.05713023031006,1.,0.748091554183802));
#33334=CARTESIAN_POINT('Ctrl Pts',(-2.05079645592154,1.,0.749287468665046));
#33335=CARTESIAN_POINT('Ctrl Pts',(-2.04446689147979,1.,0.750444657875576));
#33336=CARTESIAN_POINT('Ctrl Pts',(-2.03814160092099,1.,0.751562963361115));
#33337=CARTESIAN_POINT('Ctrl Pts',(-2.03182068456221,1.,0.752642180487211));
#33338=CARTESIAN_POINT('Ctrl Pts',(-2.02550428623313,1.,0.753682061112768));
#33339=CARTESIAN_POINT('Ctrl Pts',(-2.01919259405809,1.,0.754682330722816));
#33340=CARTESIAN_POINT('Ctrl Pts',(-2.01288584328084,1.,0.755642704957865));
#33341=CARTESIAN_POINT('Ctrl Pts',(-2.0065843158773,1.,0.75656290464667));
#33342=CARTESIAN_POINT('Ctrl Pts',(-2.00028834739178,1.,0.757442676862724));
#33343=CARTESIAN_POINT('Ctrl Pts',(-1.99399831098817,1.,0.758281796766761));
#33344=CARTESIAN_POINT('Ctrl Pts',(-1.98771456680874,1.,0.759080037802488));
#33345=CARTESIAN_POINT('Ctrl Pts',(-1.98143741418172,1.,0.75983714745219));
#33346=CARTESIAN_POINT('Ctrl Pts',(-1.97516705321494,1.,0.760552825409757));
#33347=CARTESIAN_POINT('Ctrl Pts',(-1.96890351582499,1.,0.76122669048382));
#33348=CARTESIAN_POINT('Ctrl Pts',(-1.96264672744186,1.,0.761858300014423));
#33349=CARTESIAN_POINT('Ctrl Pts',(-1.95639665309869,1.,0.762447203806179));
#33350=CARTESIAN_POINT('Ctrl Pts',(-1.95015342590024,1.,0.762992990878769));
#33351=CARTESIAN_POINT('Ctrl Pts',(-1.9439174661764,1.,0.763495333538629));
#33352=CARTESIAN_POINT('Ctrl Pts',(-1.93768964875886,1.,0.763954049121458));
#33353=CARTESIAN_POINT('Ctrl Pts',(-1.93147105496382,1.,0.76436901067394));
#33354=CARTESIAN_POINT('Ctrl Pts',(-1.92526263537048,1.,0.764740025488211));
#33355=CARTESIAN_POINT('Ctrl Pts',(-1.91906491634196,1.,0.765066729667088));
#33356=CARTESIAN_POINT('Ctrl Pts',(-1.91287765805169,1.,0.765348465884722));
#33357=CARTESIAN_POINT('Ctrl Pts',(-1.90669961402356,1.,0.765584196937919));
#33358=CARTESIAN_POINT('Ctrl Pts',(-1.90052930393596,1.,0.765772772593386));
#33359=CARTESIAN_POINT('Ctrl Pts',(-1.89436577771388,1.,0.765913193856978));
#33360=CARTESIAN_POINT('Ctrl Pts',(-1.88820926433409,1.,0.766004837062091));
#33361=CARTESIAN_POINT('Ctrl Pts',(-1.88206215302561,1.,0.766047794851864));
#33362=CARTESIAN_POINT('Ctrl Pts',(-1.87592888967883,1.,0.766042837036744));
#33363=CARTESIAN_POINT('Ctrl Pts',(-1.86981398314341,1.,0.765990708546091));
#33364=CARTESIAN_POINT('Ctrl Pts',(-1.86372027063312,1.,0.765891519092547));
#33365=CARTESIAN_POINT('Ctrl Pts',(-1.85764741390394,1.,0.765744212909318));
#33366=CARTESIAN_POINT('Ctrl Pts',(-1.85158945130063,1.,0.765545710619062));
#33367=CARTESIAN_POINT('Ctrl Pts',(-1.84553698875924,1.,0.765291664862029));
#33368=CARTESIAN_POINT('Ctrl Pts',(-1.83948181064835,1.,0.764978057881737));
#33369=CARTESIAN_POINT('Ctrl Pts',(-1.83342077227142,1.,0.764602549687853));
#33370=CARTESIAN_POINT('Ctrl Pts',(-1.82735991200065,1.,0.764165902605995));
#33371=CARTESIAN_POINT('Ctrl Pts',(-1.82131873145266,1.,0.763673465462726));
#33372=CARTESIAN_POINT('Ctrl Pts',(-1.8153211840553,1.,0.763132003836634));
#33373=CARTESIAN_POINT('Ctrl Pts',(-1.80938551463965,1.,0.762546129463938));
#33374=CARTESIAN_POINT('Ctrl Pts',(-1.80351583877342,1.,0.761915336443547));
#33375=CARTESIAN_POINT('Ctrl Pts',(-1.79768986997783,1.,0.761229695230558));
#33376=CARTESIAN_POINT('Ctrl Pts',(-1.7918581561088,1.,0.760469555880749));
#33377=CARTESIAN_POINT('Ctrl Pts',(-1.78596964884604,1.,0.759614401110189));
#33378=CARTESIAN_POINT('Ctrl Pts',(-1.77999411220945,1.,0.758650626677518));
#33379=CARTESIAN_POINT('Ctrl Pts',(-1.77394167108292,1.,0.757578264077029));
#33380=CARTESIAN_POINT('Ctrl Pts',(-1.76789396002998,1.,0.75642189602781));
#33381=CARTESIAN_POINT('Ctrl Pts',(-1.76197817240128,1.,0.755220979974461));
#33382=CARTESIAN_POINT('Ctrl Pts',(-1.75631083600019,1.,0.754009254027829));
#33383=CARTESIAN_POINT('Ctrl Pts',(-1.75095139468794,1.,0.752797683531314));
#33384=CARTESIAN_POINT('Ctrl Pts',(-1.74585086852502,1.,0.751555614164482));
#33385=CARTESIAN_POINT('Ctrl Pts',(-1.74080458267114,1.,0.750193435981249));
#33386=CARTESIAN_POINT('Ctrl Pts',(-1.7355035168033,1.,0.74858246295687));
#33387=CARTESIAN_POINT('Ctrl Pts',(-1.72958533647714,1.,0.746574710097752));
#33388=CARTESIAN_POINT('Ctrl Pts',(-1.72268229916769,1.,0.744021445433093));
#33389=CARTESIAN_POINT('Ctrl Pts',(-1.71447789751001,1.,0.74079516202821));
#33390=CARTESIAN_POINT('Ctrl Pts',(-1.70473309004249,1.,0.736799665716932));
#33391=CARTESIAN_POINT('Ctrl Pts',(-1.69326921972915,1.,0.731963238685357));
#33392=CARTESIAN_POINT('Ctrl Pts',(-1.67996158451922,1.,0.726235967982445));
#33393=CARTESIAN_POINT('Ctrl Pts',(-1.66472880551777,1.,0.71958543378795));
#33394=CARTESIAN_POINT('Ctrl Pts',(-1.64752408828442,1.,0.711993139340447));
#33395=CARTESIAN_POINT('Ctrl Pts',(-1.6321654166204,1.,0.705159151977294));
#33396=CARTESIAN_POINT('Ctrl Pts',(-1.61974673471117,1.,0.699605146398837));
#33397=CARTESIAN_POINT('Ctrl Pts',(-1.61106790957619,1.,0.69571209787897));
#33398=CARTESIAN_POINT('Ctrl Pts',(-1.60662857109684,1.,0.693717979106305));
#33399=CARTESIAN_POINT('',(-2.0698113262342,0.,0.7455743247944));
#33400=CARTESIAN_POINT('Origin',(-2.11275013067528,0.,0.61342227326009));
#33401=CARTESIAN_POINT('',(-2.11275013067528,1.,0.61342227326009));
#33402=CARTESIAN_POINT('',(-2.0698113262342,1.,0.7455743247944));
#33403=CARTESIAN_POINT('',(-2.11275013067528,0.,0.61342227326009));
#33404=CARTESIAN_POINT('Ctrl Pts',(-1.7075470150345,-1.,0.383122945602004));
#33405=CARTESIAN_POINT('Ctrl Pts',(-1.7075470150345,1.,0.383122945602004));
#33406=CARTESIAN_POINT('Ctrl Pts',(-1.71231062891958,-1.,0.384119047315542));
#33407=CARTESIAN_POINT('Ctrl Pts',(-1.71231062891958,1.,0.384119047315542));
#33408=CARTESIAN_POINT('Ctrl Pts',(-1.72162022246158,-1.,0.38607079032701));
#33409=CARTESIAN_POINT('Ctrl Pts',(-1.72162022246158,1.,0.38607079032701));
#33410=CARTESIAN_POINT('Ctrl Pts',(-1.7349317097561,-1.,0.388877023509191));
#33411=CARTESIAN_POINT('Ctrl Pts',(-1.7349317097561,1.,0.388877023509191));
#33412=CARTESIAN_POINT('Ctrl Pts',(-1.75137405313962,-1.,0.392375812294307));
#33413=CARTESIAN_POINT('Ctrl Pts',(-1.75137405313962,1.,0.392375812294307));
#33414=CARTESIAN_POINT('Ctrl Pts',(-1.7697556004756,-1.,0.39634619612042));
#33415=CARTESIAN_POINT('Ctrl Pts',(-1.7697556004756,1.,0.39634619612042));
#33416=CARTESIAN_POINT('Ctrl Pts',(-1.78598826347533,-1.,0.39991940378308));
#33417=CARTESIAN_POINT('Ctrl Pts',(-1.78598826347533,1.,0.39991940378308));
#33418=CARTESIAN_POINT('Ctrl Pts',(-1.80012077176221,-1.,0.403107976170441));
#33419=CARTESIAN_POINT('Ctrl Pts',(-1.80012077176221,1.,0.403107976170441));
#33420=CARTESIAN_POINT('Ctrl Pts',(-1.81223801813988,-1.,0.405933518411838));
#33421=CARTESIAN_POINT('Ctrl Pts',(-1.81223801813988,1.,0.405933518411838));
#33422=CARTESIAN_POINT('Ctrl Pts',(-1.8224702267854,-1.,0.408428948108533));
#33423=CARTESIAN_POINT('Ctrl Pts',(-1.8224702267854,1.,0.408428948108533));
#33424=CARTESIAN_POINT('Ctrl Pts',(-1.83100408895216,-1.,0.410641256301675));
#33425=CARTESIAN_POINT('Ctrl Pts',(-1.83100408895216,1.,0.410641256301675));
#33426=CARTESIAN_POINT('Ctrl Pts',(-1.83808953475839,-1.,0.412633125322161));
#33427=CARTESIAN_POINT('Ctrl Pts',(-1.83808953475839,1.,0.412633125322161));
#33428=CARTESIAN_POINT('Ctrl Pts',(-1.8440575707371,-1.,0.41448743825434));
#33429=CARTESIAN_POINT('Ctrl Pts',(-1.8440575707371,1.,0.41448743825434));
#33430=CARTESIAN_POINT('Ctrl Pts',(-1.84929312929882,-1.,0.416300022038864));
#33431=CARTESIAN_POINT('Ctrl Pts',(-1.84929312929882,1.,0.416300022038864));
#33432=CARTESIAN_POINT('Ctrl Pts',(-1.85417632856234,-1.,0.418164129143534));
#33433=CARTESIAN_POINT('Ctrl Pts',(-1.85417632856234,1.,0.418164129143534));
#33434=CARTESIAN_POINT('Ctrl Pts',(-1.85903281096686,-1.,0.420157287975619));
#33435=CARTESIAN_POINT('Ctrl Pts',(-1.85903281096686,1.,0.420157287975619));
#33436=CARTESIAN_POINT('Ctrl Pts',(-1.86408083334028,-1.,0.422327307418275));
#33437=CARTESIAN_POINT('Ctrl Pts',(-1.86408083334028,1.,0.422327307418275));
#33438=CARTESIAN_POINT('Ctrl Pts',(-1.86937803944323,-1.,0.424678177291359));
#33439=CARTESIAN_POINT('Ctrl Pts',(-1.86937803944323,1.,0.424678177291359));
#33440=CARTESIAN_POINT('Ctrl Pts',(-1.87486989291484,-1.,0.427183828519102));
#33441=CARTESIAN_POINT('Ctrl Pts',(-1.87486989291484,1.,0.427183828519102));
#33442=CARTESIAN_POINT('Ctrl Pts',(-1.88044229001832,-1.,0.429803062482344));
#33443=CARTESIAN_POINT('Ctrl Pts',(-1.88044229001832,1.,0.429803062482344));
#33444=CARTESIAN_POINT('Ctrl Pts',(-1.88596913666793,-1.,0.432493038548748));
#33445=CARTESIAN_POINT('Ctrl Pts',(-1.88596913666793,1.,0.432493038548748));
#33446=CARTESIAN_POINT('Ctrl Pts',(-1.89136993975504,-1.,0.435225660963383));
#33447=CARTESIAN_POINT('Ctrl Pts',(-1.89136993975504,1.,0.435225660963383));
#33448=CARTESIAN_POINT('Ctrl Pts',(-1.89663648956466,-1.,0.437995003948244));
#33449=CARTESIAN_POINT('Ctrl Pts',(-1.89663648956466,1.,0.437995003948244));
#33450=CARTESIAN_POINT('Ctrl Pts',(-1.90180124389086,-1.,0.440807833704038));
#33451=CARTESIAN_POINT('Ctrl Pts',(-1.90180124389086,1.,0.440807833704038));
#33452=CARTESIAN_POINT('Ctrl Pts',(-1.90691756144898,-1.,0.44367755684915));
#33453=CARTESIAN_POINT('Ctrl Pts',(-1.90691756144898,1.,0.44367755684915));
#33454=CARTESIAN_POINT('Ctrl Pts',(-1.9120369998112,-1.,0.446617343485711));
#33455=CARTESIAN_POINT('Ctrl Pts',(-1.9120369998112,1.,0.446617343485711));
#33456=CARTESIAN_POINT('Ctrl Pts',(-1.91718342555755,-1.,0.449632260106662));
#33457=CARTESIAN_POINT('Ctrl Pts',(-1.91718342555755,1.,0.449632260106662));
#33458=CARTESIAN_POINT('Ctrl Pts',(-1.92235380648502,-1.,0.452719478359432));
#33459=CARTESIAN_POINT('Ctrl Pts',(-1.92235380648502,1.,0.452719478359432));
#33460=CARTESIAN_POINT('Ctrl Pts',(-1.92753067150476,-1.,0.455872005174371));
#33461=CARTESIAN_POINT('Ctrl Pts',(-1.92753067150476,1.,0.455872005174371));
#33462=CARTESIAN_POINT('Ctrl Pts',(-1.93269066517934,-1.,0.459081234547926));
#33463=CARTESIAN_POINT('Ctrl Pts',(-1.93269066517934,1.,0.459081234547926));
#33464=CARTESIAN_POINT('Ctrl Pts',(-1.93781486640821,-1.,0.462340031009056));
#33465=CARTESIAN_POINT('Ctrl Pts',(-1.93781486640821,1.,0.462340031009056));
#33466=CARTESIAN_POINT('Ctrl Pts',(-1.9428979419619,-1.,0.46564546202603));
#33467=CARTESIAN_POINT('Ctrl Pts',(-1.9428979419619,1.,0.46564546202603));
#33468=CARTESIAN_POINT('Ctrl Pts',(-1.94794381136514,-1.,0.468997482913135));
#33469=CARTESIAN_POINT('Ctrl Pts',(-1.94794381136514,1.,0.468997482913135));
#33470=CARTESIAN_POINT('Ctrl Pts',(-1.95296148278133,-1.,0.472397672264072));
#33471=CARTESIAN_POINT('Ctrl Pts',(-1.95296148278133,1.,0.472397672264072));
#33472=CARTESIAN_POINT('Ctrl Pts',(-1.95796111148177,-1.,0.475848034683176));
#33473=CARTESIAN_POINT('Ctrl Pts',(-1.95796111148177,1.,0.475848034683176));
#33474=CARTESIAN_POINT('Ctrl Pts',(-1.96294933055943,-1.,0.479349583074855));
#33475=CARTESIAN_POINT('Ctrl Pts',(-1.96294933055943,1.,0.479349583074855));
#33476=CARTESIAN_POINT('Ctrl Pts',(-1.96792703422362,-1.,0.48290166212069));
#33477=CARTESIAN_POINT('Ctrl Pts',(-1.96792703422362,1.,0.48290166212069));
#33478=CARTESIAN_POINT('Ctrl Pts',(-1.97289186263272,-1.,0.486502692907659));
#33479=CARTESIAN_POINT('Ctrl Pts',(-1.97289186263272,1.,0.486502692907659));
#33480=CARTESIAN_POINT('Ctrl Pts',(-1.97783973019229,-1.,0.490150627860952));
#33481=CARTESIAN_POINT('Ctrl Pts',(-1.97783973019229,1.,0.490150627860952));
#33482=CARTESIAN_POINT('Ctrl Pts',(-1.98276658761821,-1.,0.493843476541494));
#33483=CARTESIAN_POINT('Ctrl Pts',(-1.98276658761821,1.,0.493843476541494));
#33484=CARTESIAN_POINT('Ctrl Pts',(-1.98767044752932,-1.,0.497579909545574));
#33485=CARTESIAN_POINT('Ctrl Pts',(-1.98767044752932,1.,0.497579909545574));
#33486=CARTESIAN_POINT('Ctrl Pts',(-1.99255149126155,-1.,0.501359287727146));
#33487=CARTESIAN_POINT('Ctrl Pts',(-1.99255149126155,1.,0.501359287727146));
#33488=CARTESIAN_POINT('Ctrl Pts',(-1.99741107463572,-1.,0.505181361323026));
#33489=CARTESIAN_POINT('Ctrl Pts',(-1.99741107463572,1.,0.505181361323026));
#33490=CARTESIAN_POINT('Ctrl Pts',(-2.00225107134734,-1.,0.509046069886157));
#33491=CARTESIAN_POINT('Ctrl Pts',(-2.00225107134734,1.,0.509046069886157));
#33492=CARTESIAN_POINT('Ctrl Pts',(-2.00707309946949,-1.,0.512953306961792));
#33493=CARTESIAN_POINT('Ctrl Pts',(-2.00707309946949,1.,0.512953306961792));
#33494=CARTESIAN_POINT('Ctrl Pts',(-2.01187773939242,-1.,0.516902681728687));
#33495=CARTESIAN_POINT('Ctrl Pts',(-2.01187773939242,1.,0.516902681728687));
#33496=CARTESIAN_POINT('Ctrl Pts',(-2.01666477917286,-1.,0.52089359039937));
#33497=CARTESIAN_POINT('Ctrl Pts',(-2.01666477917286,1.,0.52089359039937));
#33498=CARTESIAN_POINT('Ctrl Pts',(-2.02143356304698,-1.,0.524925318333476));
#33499=CARTESIAN_POINT('Ctrl Pts',(-2.02143356304698,1.,0.524925318333476));
#33500=CARTESIAN_POINT('Ctrl Pts',(-2.0261832908329,-1.,0.528997127241914));
#33501=CARTESIAN_POINT('Ctrl Pts',(-2.0261832908329,1.,0.528997127241914));
#33502=CARTESIAN_POINT('Ctrl Pts',(-2.03091336214426,-1.,0.533108355132976));
#33503=CARTESIAN_POINT('Ctrl Pts',(-2.03091336214426,1.,0.533108355132976));
#33504=CARTESIAN_POINT('Ctrl Pts',(-2.03562362954037,-1.,0.537258489833262));
#33505=CARTESIAN_POINT('Ctrl Pts',(-2.03562362954037,1.,0.537258489833262));
#33506=CARTESIAN_POINT('Ctrl Pts',(-2.04031422690527,-1.,0.541447120615659));
#33507=CARTESIAN_POINT('Ctrl Pts',(-2.04031422690527,1.,0.541447120615659));
#33508=CARTESIAN_POINT('Ctrl Pts',(-2.04498544714588,-1.,0.54567390381743));
#33509=CARTESIAN_POINT('Ctrl Pts',(-2.04498544714588,1.,0.54567390381743));
#33510=CARTESIAN_POINT('Ctrl Pts',(-2.04963761077958,-1.,0.549938525150295));
#33511=CARTESIAN_POINT('Ctrl Pts',(-2.04963761077958,1.,0.549938525150295));
#33512=CARTESIAN_POINT('Ctrl Pts',(-2.05427091604413,-1.,0.554240657463906));
#33513=CARTESIAN_POINT('Ctrl Pts',(-2.05427091604413,1.,0.554240657463906));
#33514=CARTESIAN_POINT('Ctrl Pts',(-2.05888537756462,-1.,0.558579940185151));
#33515=CARTESIAN_POINT('Ctrl Pts',(-2.05888537756462,1.,0.558579940185151));
#33516=CARTESIAN_POINT('Ctrl Pts',(-2.06348090160589,-1.,0.562955993082261));
#33517=CARTESIAN_POINT('Ctrl Pts',(-2.06348090160589,1.,0.562955993082261));
#33518=CARTESIAN_POINT('Ctrl Pts',(-2.06805732997334,-1.,0.567368421181087));
#33519=CARTESIAN_POINT('Ctrl Pts',(-2.06805732997334,1.,0.567368421181087));
#33520=CARTESIAN_POINT('Ctrl Pts',(-2.07261449292824,-1.,0.571816823242603));
#33521=CARTESIAN_POINT('Ctrl Pts',(-2.07261449292824,1.,0.571816823242603));
#33522=CARTESIAN_POINT('Ctrl Pts',(-2.07715226767559,-1.,0.576300797416844));
#33523=CARTESIAN_POINT('Ctrl Pts',(-2.07715226767559,1.,0.576300797416844));
#33524=CARTESIAN_POINT('Ctrl Pts',(-2.08167059018418,-1.,0.580819952108063));
#33525=CARTESIAN_POINT('Ctrl Pts',(-2.08167059018418,1.,0.580819952108063));
#33526=CARTESIAN_POINT('Ctrl Pts',(-2.08616943727951,-1.,0.585373918991617));
#33527=CARTESIAN_POINT('Ctrl Pts',(-2.08616943727951,1.,0.585373918991617));
#33528=CARTESIAN_POINT('Ctrl Pts',(-2.09064881812129,-1.,0.589962365403406));
#33529=CARTESIAN_POINT('Ctrl Pts',(-2.09064881812129,1.,0.589962365403406));
#33530=CARTESIAN_POINT('Ctrl Pts',(-2.0951087622027,-1.,0.594585006052162));
#33531=CARTESIAN_POINT('Ctrl Pts',(-2.0951087622027,1.,0.594585006052162));
#33532=CARTESIAN_POINT('Ctrl Pts',(-2.0995493086477,-1.,0.599241616420533));
#33533=CARTESIAN_POINT('Ctrl Pts',(-2.0995493086477,1.,0.599241616420533));
#33534=CARTESIAN_POINT('Ctrl Pts',(-2.10397049886949,-1.,0.60393203073603));
#33535=CARTESIAN_POINT('Ctrl Pts',(-2.10397049886949,1.,0.60393203073603));
#33536=CARTESIAN_POINT('Ctrl Pts',(-2.1074919961518,-1.,0.607711315454876));
#33537=CARTESIAN_POINT('Ctrl Pts',(-2.1074919961518,1.,0.607711315454876));
#33538=CARTESIAN_POINT('Ctrl Pts',(-2.11012443807238,-1.,0.610560911689899));
#33539=CARTESIAN_POINT('Ctrl Pts',(-2.11012443807238,1.,0.610560911689899));
#33540=CARTESIAN_POINT('Ctrl Pts',(-2.11187554259986,-1.,0.6124673655618));
#33541=CARTESIAN_POINT('Ctrl Pts',(-2.11187554259986,1.,0.6124673655618));
#33542=CARTESIAN_POINT('Ctrl Pts',(-2.11275013067528,-1.,0.61342227326009));
#33543=CARTESIAN_POINT('Ctrl Pts',(-2.11275013067528,1.,0.61342227326009));
#33544=CARTESIAN_POINT('',(-1.7075470150345,1.,0.383122945602004));
#33545=CARTESIAN_POINT('Ctrl Pts',(-1.7075470150345,1.,0.383122945602004));
#33546=CARTESIAN_POINT('Ctrl Pts',(-1.71231062891958,1.,0.384119047315542));
#33547=CARTESIAN_POINT('Ctrl Pts',(-1.72162022246158,1.,0.38607079032701));
#33548=CARTESIAN_POINT('Ctrl Pts',(-1.7349317097561,1.,0.388877023509191));
#33549=CARTESIAN_POINT('Ctrl Pts',(-1.75137405313962,1.,0.392375812294307));
#33550=CARTESIAN_POINT('Ctrl Pts',(-1.7697556004756,1.,0.39634619612042));
#33551=CARTESIAN_POINT('Ctrl Pts',(-1.78598826347533,1.,0.39991940378308));
#33552=CARTESIAN_POINT('Ctrl Pts',(-1.80012077176221,1.,0.403107976170441));
#33553=CARTESIAN_POINT('Ctrl Pts',(-1.81223801813988,1.,0.405933518411838));
#33554=CARTESIAN_POINT('Ctrl Pts',(-1.8224702267854,1.,0.408428948108533));
#33555=CARTESIAN_POINT('Ctrl Pts',(-1.83100408895216,1.,0.410641256301675));
#33556=CARTESIAN_POINT('Ctrl Pts',(-1.83808953475839,1.,0.412633125322161));
#33557=CARTESIAN_POINT('Ctrl Pts',(-1.8440575707371,1.,0.41448743825434));
#33558=CARTESIAN_POINT('Ctrl Pts',(-1.84929312929882,1.,0.416300022038864));
#33559=CARTESIAN_POINT('Ctrl Pts',(-1.85417632856234,1.,0.418164129143534));
#33560=CARTESIAN_POINT('Ctrl Pts',(-1.85903281096686,1.,0.420157287975619));
#33561=CARTESIAN_POINT('Ctrl Pts',(-1.86408083334028,1.,0.422327307418275));
#33562=CARTESIAN_POINT('Ctrl Pts',(-1.86937803944323,1.,0.424678177291359));
#33563=CARTESIAN_POINT('Ctrl Pts',(-1.87486989291484,1.,0.427183828519102));
#33564=CARTESIAN_POINT('Ctrl Pts',(-1.88044229001832,1.,0.429803062482344));
#33565=CARTESIAN_POINT('Ctrl Pts',(-1.88596913666793,1.,0.432493038548748));
#33566=CARTESIAN_POINT('Ctrl Pts',(-1.89136993975504,1.,0.435225660963383));
#33567=CARTESIAN_POINT('Ctrl Pts',(-1.89663648956466,1.,0.437995003948244));
#33568=CARTESIAN_POINT('Ctrl Pts',(-1.90180124389086,1.,0.440807833704038));
#33569=CARTESIAN_POINT('Ctrl Pts',(-1.90691756144898,1.,0.44367755684915));
#33570=CARTESIAN_POINT('Ctrl Pts',(-1.9120369998112,1.,0.446617343485711));
#33571=CARTESIAN_POINT('Ctrl Pts',(-1.91718342555755,1.,0.449632260106662));
#33572=CARTESIAN_POINT('Ctrl Pts',(-1.92235380648502,1.,0.452719478359432));
#33573=CARTESIAN_POINT('Ctrl Pts',(-1.92753067150476,1.,0.455872005174371));
#33574=CARTESIAN_POINT('Ctrl Pts',(-1.93269066517934,1.,0.459081234547926));
#33575=CARTESIAN_POINT('Ctrl Pts',(-1.93781486640821,1.,0.462340031009056));
#33576=CARTESIAN_POINT('Ctrl Pts',(-1.9428979419619,1.,0.46564546202603));
#33577=CARTESIAN_POINT('Ctrl Pts',(-1.94794381136514,1.,0.468997482913135));
#33578=CARTESIAN_POINT('Ctrl Pts',(-1.95296148278133,1.,0.472397672264072));
#33579=CARTESIAN_POINT('Ctrl Pts',(-1.95796111148177,1.,0.475848034683176));
#33580=CARTESIAN_POINT('Ctrl Pts',(-1.96294933055943,1.,0.479349583074855));
#33581=CARTESIAN_POINT('Ctrl Pts',(-1.96792703422362,1.,0.48290166212069));
#33582=CARTESIAN_POINT('Ctrl Pts',(-1.97289186263272,1.,0.486502692907659));
#33583=CARTESIAN_POINT('Ctrl Pts',(-1.97783973019229,1.,0.490150627860952));
#33584=CARTESIAN_POINT('Ctrl Pts',(-1.98276658761821,1.,0.493843476541494));
#33585=CARTESIAN_POINT('Ctrl Pts',(-1.98767044752932,1.,0.497579909545574));
#33586=CARTESIAN_POINT('Ctrl Pts',(-1.99255149126155,1.,0.501359287727146));
#33587=CARTESIAN_POINT('Ctrl Pts',(-1.99741107463572,1.,0.505181361323026));
#33588=CARTESIAN_POINT('Ctrl Pts',(-2.00225107134734,1.,0.509046069886157));
#33589=CARTESIAN_POINT('Ctrl Pts',(-2.00707309946949,1.,0.512953306961792));
#33590=CARTESIAN_POINT('Ctrl Pts',(-2.01187773939242,1.,0.516902681728687));
#33591=CARTESIAN_POINT('Ctrl Pts',(-2.01666477917286,1.,0.52089359039937));
#33592=CARTESIAN_POINT('Ctrl Pts',(-2.02143356304698,1.,0.524925318333476));
#33593=CARTESIAN_POINT('Ctrl Pts',(-2.0261832908329,1.,0.528997127241914));
#33594=CARTESIAN_POINT('Ctrl Pts',(-2.03091336214426,1.,0.533108355132976));
#33595=CARTESIAN_POINT('Ctrl Pts',(-2.03562362954037,1.,0.537258489833262));
#33596=CARTESIAN_POINT('Ctrl Pts',(-2.04031422690527,1.,0.541447120615659));
#33597=CARTESIAN_POINT('Ctrl Pts',(-2.04498544714588,1.,0.54567390381743));
#33598=CARTESIAN_POINT('Ctrl Pts',(-2.04963761077958,1.,0.549938525150295));
#33599=CARTESIAN_POINT('Ctrl Pts',(-2.05427091604413,1.,0.554240657463906));
#33600=CARTESIAN_POINT('Ctrl Pts',(-2.05888537756462,1.,0.558579940185151));
#33601=CARTESIAN_POINT('Ctrl Pts',(-2.06348090160589,1.,0.562955993082261));
#33602=CARTESIAN_POINT('Ctrl Pts',(-2.06805732997334,1.,0.567368421181087));
#33603=CARTESIAN_POINT('Ctrl Pts',(-2.07261449292824,1.,0.571816823242603));
#33604=CARTESIAN_POINT('Ctrl Pts',(-2.07715226767559,1.,0.576300797416844));
#33605=CARTESIAN_POINT('Ctrl Pts',(-2.08167059018418,1.,0.580819952108063));
#33606=CARTESIAN_POINT('Ctrl Pts',(-2.08616943727951,1.,0.585373918991617));
#33607=CARTESIAN_POINT('Ctrl Pts',(-2.09064881812129,1.,0.589962365403406));
#33608=CARTESIAN_POINT('Ctrl Pts',(-2.0951087622027,1.,0.594585006052162));
#33609=CARTESIAN_POINT('Ctrl Pts',(-2.0995493086477,1.,0.599241616420533));
#33610=CARTESIAN_POINT('Ctrl Pts',(-2.10397049886949,1.,0.60393203073603));
#33611=CARTESIAN_POINT('Ctrl Pts',(-2.1074919961518,1.,0.607711315454876));
#33612=CARTESIAN_POINT('Ctrl Pts',(-2.11012443807238,1.,0.610560911689899));
#33613=CARTESIAN_POINT('Ctrl Pts',(-2.11187554259986,1.,0.6124673655618));
#33614=CARTESIAN_POINT('Ctrl Pts',(-2.11275013067528,1.,0.61342227326009));
#33615=CARTESIAN_POINT('',(-1.7075470150345,0.,0.383122945602003));
#33616=CARTESIAN_POINT('Origin',(0.,0.,0.));
#33617=CARTESIAN_POINT('',(-1.74236521665491,1.,0.163289472382896));
#33618=CARTESIAN_POINT('Origin',(0.,1.,0.));
#33619=CARTESIAN_POINT('',(-1.74236521665491,0.,0.163289472382896));
#33620=CARTESIAN_POINT('Ctrl Pts',(-2.19890268624765,-1.,0.069476445021958));
#33621=CARTESIAN_POINT('Ctrl Pts',(-2.19890268624765,1.,0.069476445021958));
#33622=CARTESIAN_POINT('Ctrl Pts',(-2.19777582085423,-1.,0.0701143536325489));
#33623=CARTESIAN_POINT('Ctrl Pts',(-2.19777582085423,1.,0.0701143536325489));
#33624=CARTESIAN_POINT('Ctrl Pts',(-2.19552129484002,-1.,0.0713863779526153));
#33625=CARTESIAN_POINT('Ctrl Pts',(-2.19552129484002,1.,0.0713863779526153));
#33626=CARTESIAN_POINT('Ctrl Pts',(-2.19213712013662,-1.,0.0732830357306724));
#33627=CARTESIAN_POINT('Ctrl Pts',(-2.19213712013662,1.,0.0732830357306724));
#33628=CARTESIAN_POINT('Ctrl Pts',(-2.1876201139953,-1.,0.0757891465836146));
#33629=CARTESIAN_POINT('Ctrl Pts',(-2.1876201139953,1.,0.0757891465836146));
#33630=CARTESIAN_POINT('Ctrl Pts',(-2.18196589448887,-1.,0.0788837727685241));
#33631=CARTESIAN_POINT('Ctrl Pts',(-2.18196589448887,1.,0.0788837727685241));
#33632=CARTESIAN_POINT('Ctrl Pts',(-2.176303712113,-1.,0.0819402680872764));
#33633=CARTESIAN_POINT('Ctrl Pts',(-2.176303712113,1.,0.0819402680872764));
#33634=CARTESIAN_POINT('Ctrl Pts',(-2.17063357870952,-1.,0.0849584620835371));
#33635=CARTESIAN_POINT('Ctrl Pts',(-2.17063357870952,1.,0.0849584620835371));
#33636=CARTESIAN_POINT('Ctrl Pts',(-2.16495552645014,-1.,0.0879381291386921));
#33637=CARTESIAN_POINT('Ctrl Pts',(-2.16495552645014,1.,0.0879381291386921));
#33638=CARTESIAN_POINT('Ctrl Pts',(-2.15926961544516,-1.,0.0908789888107264));
#33639=CARTESIAN_POINT('Ctrl Pts',(-2.15926961544516,1.,0.0908789888107264));
#33640=CARTESIAN_POINT('Ctrl Pts',(-2.1535759397817,-1.,0.0937807218867642));
#33641=CARTESIAN_POINT('Ctrl Pts',(-2.1535759397817,1.,0.0937807218867642));
#33642=CARTESIAN_POINT('Ctrl Pts',(-2.14787463531795,-1.,0.0966429852305457));
#33643=CARTESIAN_POINT('Ctrl Pts',(-2.14787463531795,1.,0.0966429852305457));
#33644=CARTESIAN_POINT('Ctrl Pts',(-2.14216588396025,-1.,0.0994654261990914));
#33645=CARTESIAN_POINT('Ctrl Pts',(-2.14216588396025,1.,0.0994654261990914));
#33646=CARTESIAN_POINT('Ctrl Pts',(-2.13644992667165,-1.,0.1022477005561));
#33647=CARTESIAN_POINT('Ctrl Pts',(-2.13644992667165,1.,0.1022477005561));
#33648=CARTESIAN_POINT('Ctrl Pts',(-2.13072704887293,-1.,0.104989479152739));
#33649=CARTESIAN_POINT('Ctrl Pts',(-2.13072704887293,1.,0.104989479152739));
#33650=CARTESIAN_POINT('Ctrl Pts',(-2.12499752307,-1.,0.10769043523109));
#33651=CARTESIAN_POINT('Ctrl Pts',(-2.12499752307,1.,0.10769043523109));
#33652=CARTESIAN_POINT('Ctrl Pts',(-2.11926155590865,-1.,0.110350236135025));
#33653=CARTESIAN_POINT('Ctrl Pts',(-2.11926155590865,1.,0.110350236135025));
#33654=CARTESIAN_POINT('Ctrl Pts',(-2.11351924490306,-1.,0.112968534419737));
#33655=CARTESIAN_POINT('Ctrl Pts',(-2.11351924490306,1.,0.112968534419737));
#33656=CARTESIAN_POINT('Ctrl Pts',(-2.10777050261309,-1.,0.115544957687926));
#33657=CARTESIAN_POINT('Ctrl Pts',(-2.10777050261309,1.,0.115544957687926));
#33658=CARTESIAN_POINT('Ctrl Pts',(-2.102015121329,-1.,0.118079107988355));
#33659=CARTESIAN_POINT('Ctrl Pts',(-2.102015121329,1.,0.118079107988355));
#33660=CARTESIAN_POINT('Ctrl Pts',(-2.0962529286773,-1.,0.120570567965122));
#33661=CARTESIAN_POINT('Ctrl Pts',(-2.0962529286773,1.,0.120570567965122));
#33662=CARTESIAN_POINT('Ctrl Pts',(-2.09048392424825,-1.,0.123018905621083));
#33663=CARTESIAN_POINT('Ctrl Pts',(-2.09048392424825,1.,0.123018905621083));
#33664=CARTESIAN_POINT('Ctrl Pts',(-2.08470840653643,-1.,0.125423679412061));
#33665=CARTESIAN_POINT('Ctrl Pts',(-2.08470840653643,1.,0.125423679412061));
#33666=CARTESIAN_POINT('Ctrl Pts',(-2.07892715110987,-1.,0.12778444527612));
#33667=CARTESIAN_POINT('Ctrl Pts',(-2.07892715110987,1.,0.12778444527612));
#33668=CARTESIAN_POINT('Ctrl Pts',(-2.07314114713063,-1.,0.130100748328403));
#33669=CARTESIAN_POINT('Ctrl Pts',(-2.07314114713063,1.,0.130100748328403));
#33670=CARTESIAN_POINT('Ctrl Pts',(-2.06735123910326,-1.,0.13237211154771));
#33671=CARTESIAN_POINT('Ctrl Pts',(-2.06735123910326,1.,0.13237211154771));
#33672=CARTESIAN_POINT('Ctrl Pts',(-2.06155781517842,-1.,0.134598026192106));
#33673=CARTESIAN_POINT('Ctrl Pts',(-2.06155781517842,1.,0.134598026192106));
#33674=CARTESIAN_POINT('Ctrl Pts',(-2.05576044414264,-1.,0.136777941218043));
#33675=CARTESIAN_POINT('Ctrl Pts',(-2.05576044414264,1.,0.136777941218043));
#33676=CARTESIAN_POINT('Ctrl Pts',(-2.04995762001328,-1.,0.138911255368966));
#33677=CARTESIAN_POINT('Ctrl Pts',(-2.04995762001328,1.,0.138911255368966));
#33678=CARTESIAN_POINT('Ctrl Pts',(-2.04414757947916,-1.,0.140997332152546));
#33679=CARTESIAN_POINT('Ctrl Pts',(-2.04414757947916,1.,0.140997332152546));
#33680=CARTESIAN_POINT('Ctrl Pts',(-2.03832911025912,-1.,0.143035515058209));
#33681=CARTESIAN_POINT('Ctrl Pts',(-2.03832911025912,1.,0.143035515058209));
#33682=CARTESIAN_POINT('Ctrl Pts',(-2.03250223739942,-1.,0.145025140186057));
#33683=CARTESIAN_POINT('Ctrl Pts',(-2.03250223739942,1.,0.145025140186057));
#33684=CARTESIAN_POINT('Ctrl Pts',(-2.02666926182017,-1.,0.146965557332583));
#33685=CARTESIAN_POINT('Ctrl Pts',(-2.02666926182017,1.,0.146965557332583));
#33686=CARTESIAN_POINT('Ctrl Pts',(-2.02083464969894,-1.,0.148856124775337));
#33687=CARTESIAN_POINT('Ctrl Pts',(-2.02083464969894,1.,0.148856124775337));
#33688=CARTESIAN_POINT('Ctrl Pts',(-2.01500291940238,-1.,0.150696157673078));
#33689=CARTESIAN_POINT('Ctrl Pts',(-2.01500291940238,1.,0.150696157673078));
#33690=CARTESIAN_POINT('Ctrl Pts',(-2.00917680318424,-1.,0.15248488362145));
#33691=CARTESIAN_POINT('Ctrl Pts',(-2.00917680318424,1.,0.15248488362145));
#33692=CARTESIAN_POINT('Ctrl Pts',(-2.00335565310543,-1.,0.154221403049722));
#33693=CARTESIAN_POINT('Ctrl Pts',(-2.00335565310543,1.,0.154221403049722));
#33694=CARTESIAN_POINT('Ctrl Pts',(-1.99753284771497,-1.,0.155904629548783));
#33695=CARTESIAN_POINT('Ctrl Pts',(-1.99753284771497,1.,0.155904629548783));
#33696=CARTESIAN_POINT('Ctrl Pts',(-1.99169810931908,-1.,0.157533331459227));
#33697=CARTESIAN_POINT('Ctrl Pts',(-1.99169810931908,1.,0.157533331459227));
#33698=CARTESIAN_POINT('Ctrl Pts',(-1.98584238283292,-1.,0.159106226437299));
#33699=CARTESIAN_POINT('Ctrl Pts',(-1.98584238283292,1.,0.159106226437299));
#33700=CARTESIAN_POINT('Ctrl Pts',(-1.97996195437559,-1.,0.160622060784611));
#33701=CARTESIAN_POINT('Ctrl Pts',(-1.97996195437559,1.,0.160622060784611));
#33702=CARTESIAN_POINT('Ctrl Pts',(-1.97406280235188,-1.,0.162079693556288));
#33703=CARTESIAN_POINT('Ctrl Pts',(-1.97406280235188,1.,0.162079693556288));
#33704=CARTESIAN_POINT('Ctrl Pts',(-1.96816512677967,-1.,0.163478185457734));
#33705=CARTESIAN_POINT('Ctrl Pts',(-1.96816512677967,1.,0.163478185457734));
#33706=CARTESIAN_POINT('Ctrl Pts',(-1.96229379940136,-1.,0.164816568920269));
#33707=CARTESIAN_POINT('Ctrl Pts',(-1.96229379940136,1.,0.164816568920269));
#33708=CARTESIAN_POINT('Ctrl Pts',(-1.9564675971873,-1.,0.166093592002812));
#33709=CARTESIAN_POINT('Ctrl Pts',(-1.9564675971873,1.,0.166093592002812));
#33710=CARTESIAN_POINT('Ctrl Pts',(-1.95069027794294,-1.,0.167307501784475));
#33711=CARTESIAN_POINT('Ctrl Pts',(-1.95069027794294,1.,0.167307501784475));
#33712=CARTESIAN_POINT('Ctrl Pts',(-1.94493757756931,-1.,0.168455741607556));
#33713=CARTESIAN_POINT('Ctrl Pts',(-1.94493757756931,1.,0.168455741607556));
#33714=CARTESIAN_POINT('Ctrl Pts',(-1.93915639211581,-1.,0.169534904817491));
#33715=CARTESIAN_POINT('Ctrl Pts',(-1.93915639211581,1.,0.169534904817491));
#33716=CARTESIAN_POINT('Ctrl Pts',(-1.93329183155539,-1.,0.170541253116201));
#33717=CARTESIAN_POINT('Ctrl Pts',(-1.93329183155539,1.,0.170541253116201));
#33718=CARTESIAN_POINT('Ctrl Pts',(-1.92731093582036,-1.,0.171471191532988));
#33719=CARTESIAN_POINT('Ctrl Pts',(-1.92731093582036,1.,0.171471191532988));
#33720=CARTESIAN_POINT('Ctrl Pts',(-1.9212233439798,-1.,0.172321621259514));
#33721=CARTESIAN_POINT('Ctrl Pts',(-1.9212233439798,1.,0.172321621259514));
#33722=CARTESIAN_POINT('Ctrl Pts',(-1.91511429159527,-1.,0.173090695383496));
#33723=CARTESIAN_POINT('Ctrl Pts',(-1.91511429159527,1.,0.173090695383496));
#33724=CARTESIAN_POINT('Ctrl Pts',(-1.90911693975267,-1.,0.173776635257817));
#33725=CARTESIAN_POINT('Ctrl Pts',(-1.90911693975267,1.,0.173776635257817));
#33726=CARTESIAN_POINT('Ctrl Pts',(-1.90335253862834,-1.,0.174375518661085));
#33727=CARTESIAN_POINT('Ctrl Pts',(-1.90335253862834,1.,0.174375518661085));
#33728=CARTESIAN_POINT('Ctrl Pts',(-1.89788101117132,-1.,0.174879405091263));
#33729=CARTESIAN_POINT('Ctrl Pts',(-1.89788101117132,1.,0.174879405091263));
#33730=CARTESIAN_POINT('Ctrl Pts',(-1.892646301985,-1.,0.175274276190844));
#33731=CARTESIAN_POINT('Ctrl Pts',(-1.892646301985,1.,0.175274276190844));
#33732=CARTESIAN_POINT('Ctrl Pts',(-1.88742606273259,-1.,0.175538155840648));
#33733=CARTESIAN_POINT('Ctrl Pts',(-1.88742606273259,1.,0.175538155840648));
#33734=CARTESIAN_POINT('Ctrl Pts',(-1.88188663145367,-1.,0.175644148889698));
#33735=CARTESIAN_POINT('Ctrl Pts',(-1.88188663145367,1.,0.175644148889698));
#33736=CARTESIAN_POINT('Ctrl Pts',(-1.87563767773588,-1.,0.175563480746485));
#33737=CARTESIAN_POINT('Ctrl Pts',(-1.87563767773588,1.,0.175563480746485));
#33738=CARTESIAN_POINT('Ctrl Pts',(-1.86828349694799,-1.,0.175268337590758));
#33739=CARTESIAN_POINT('Ctrl Pts',(-1.86828349694799,1.,0.175268337590758));
#33740=CARTESIAN_POINT('Ctrl Pts',(-1.85948367088837,-1.,0.17473525927603));
#33741=CARTESIAN_POINT('Ctrl Pts',(-1.85948367088837,1.,0.17473525927603));
#33742=CARTESIAN_POINT('Ctrl Pts',(-1.8489811319852,-1.,0.173946627587731));
#33743=CARTESIAN_POINT('Ctrl Pts',(-1.8489811319852,1.,0.173946627587731));
#33744=CARTESIAN_POINT('Ctrl Pts',(-1.83658380527692,-1.,0.1728894428919));
#33745=CARTESIAN_POINT('Ctrl Pts',(-1.83658380527692,1.,0.1728894428919));
#33746=CARTESIAN_POINT('Ctrl Pts',(-1.82215766811545,-1.,0.171554770204119));
#33747=CARTESIAN_POINT('Ctrl Pts',(-1.82215766811545,1.,0.171554770204119));
#33748=CARTESIAN_POINT('Ctrl Pts',(-1.80561530629706,-1.,0.169936923904608));
#33749=CARTESIAN_POINT('Ctrl Pts',(-1.80561530629706,1.,0.169936923904608));
#33750=CARTESIAN_POINT('Ctrl Pts',(-1.7869064998507,-1.,0.168032772805197));
#33751=CARTESIAN_POINT('Ctrl Pts',(-1.7869064998507,1.,0.168032772805197));
#33752=CARTESIAN_POINT('Ctrl Pts',(-1.77018771684844,-1.,0.1662793551464));
#33753=CARTESIAN_POINT('Ctrl Pts',(-1.77018771684844,1.,0.1662793551464));
#33754=CARTESIAN_POINT('Ctrl Pts',(-1.75666056638427,-1.,0.164834765707158));
#33755=CARTESIAN_POINT('Ctrl Pts',(-1.75666056638427,1.,0.164834765707158));
#33756=CARTESIAN_POINT('Ctrl Pts',(-1.7472034950333,-1.,0.163814161002002));
#33757=CARTESIAN_POINT('Ctrl Pts',(-1.7472034950333,1.,0.163814161002002));
#33758=CARTESIAN_POINT('Ctrl Pts',(-1.74236521665491,-1.,0.163289472382896));
#33759=CARTESIAN_POINT('Ctrl Pts',(-1.74236521665491,1.,0.163289472382896));
#33760=CARTESIAN_POINT('',(-2.19890268624765,1.,0.069476445021958));
#33761=CARTESIAN_POINT('Ctrl Pts',(-2.19890268624765,1.,0.069476445021958));
#33762=CARTESIAN_POINT('Ctrl Pts',(-2.19777582085423,1.,0.0701143536325489));
#33763=CARTESIAN_POINT('Ctrl Pts',(-2.19552129484002,1.,0.0713863779526153));
#33764=CARTESIAN_POINT('Ctrl Pts',(-2.19213712013662,1.,0.0732830357306724));
#33765=CARTESIAN_POINT('Ctrl Pts',(-2.1876201139953,1.,0.0757891465836146));
#33766=CARTESIAN_POINT('Ctrl Pts',(-2.18196589448887,1.,0.0788837727685241));
#33767=CARTESIAN_POINT('Ctrl Pts',(-2.176303712113,1.,0.0819402680872764));
#33768=CARTESIAN_POINT('Ctrl Pts',(-2.17063357870952,1.,0.0849584620835371));
#33769=CARTESIAN_POINT('Ctrl Pts',(-2.16495552645014,1.,0.0879381291386921));
#33770=CARTESIAN_POINT('Ctrl Pts',(-2.15926961544516,1.,0.0908789888107264));
#33771=CARTESIAN_POINT('Ctrl Pts',(-2.1535759397817,1.,0.0937807218867642));
#33772=CARTESIAN_POINT('Ctrl Pts',(-2.14787463531795,1.,0.0966429852305457));
#33773=CARTESIAN_POINT('Ctrl Pts',(-2.14216588396025,1.,0.0994654261990914));
#33774=CARTESIAN_POINT('Ctrl Pts',(-2.13644992667165,1.,0.1022477005561));
#33775=CARTESIAN_POINT('Ctrl Pts',(-2.13072704887293,1.,0.104989479152739));
#33776=CARTESIAN_POINT('Ctrl Pts',(-2.12499752307,1.,0.10769043523109));
#33777=CARTESIAN_POINT('Ctrl Pts',(-2.11926155590865,1.,0.110350236135025));
#33778=CARTESIAN_POINT('Ctrl Pts',(-2.11351924490306,1.,0.112968534419737));
#33779=CARTESIAN_POINT('Ctrl Pts',(-2.10777050261309,1.,0.115544957687926));
#33780=CARTESIAN_POINT('Ctrl Pts',(-2.102015121329,1.,0.118079107988355));
#33781=CARTESIAN_POINT('Ctrl Pts',(-2.0962529286773,1.,0.120570567965122));
#33782=CARTESIAN_POINT('Ctrl Pts',(-2.09048392424825,1.,0.123018905621083));
#33783=CARTESIAN_POINT('Ctrl Pts',(-2.08470840653643,1.,0.125423679412061));
#33784=CARTESIAN_POINT('Ctrl Pts',(-2.07892715110987,1.,0.12778444527612));
#33785=CARTESIAN_POINT('Ctrl Pts',(-2.07314114713063,1.,0.130100748328403));
#33786=CARTESIAN_POINT('Ctrl Pts',(-2.06735123910326,1.,0.13237211154771));
#33787=CARTESIAN_POINT('Ctrl Pts',(-2.06155781517842,1.,0.134598026192106));
#33788=CARTESIAN_POINT('Ctrl Pts',(-2.05576044414264,1.,0.136777941218043));
#33789=CARTESIAN_POINT('Ctrl Pts',(-2.04995762001328,1.,0.138911255368966));
#33790=CARTESIAN_POINT('Ctrl Pts',(-2.04414757947916,1.,0.140997332152546));
#33791=CARTESIAN_POINT('Ctrl Pts',(-2.03832911025912,1.,0.143035515058209));
#33792=CARTESIAN_POINT('Ctrl Pts',(-2.03250223739942,1.,0.145025140186057));
#33793=CARTESIAN_POINT('Ctrl Pts',(-2.02666926182017,1.,0.146965557332583));
#33794=CARTESIAN_POINT('Ctrl Pts',(-2.02083464969894,1.,0.148856124775337));
#33795=CARTESIAN_POINT('Ctrl Pts',(-2.01500291940238,1.,0.150696157673078));
#33796=CARTESIAN_POINT('Ctrl Pts',(-2.00917680318424,1.,0.15248488362145));
#33797=CARTESIAN_POINT('Ctrl Pts',(-2.00335565310543,1.,0.154221403049722));
#33798=CARTESIAN_POINT('Ctrl Pts',(-1.99753284771497,1.,0.155904629548783));
#33799=CARTESIAN_POINT('Ctrl Pts',(-1.99169810931908,1.,0.157533331459227));
#33800=CARTESIAN_POINT('Ctrl Pts',(-1.98584238283292,1.,0.159106226437299));
#33801=CARTESIAN_POINT('Ctrl Pts',(-1.97996195437559,1.,0.160622060784611));
#33802=CARTESIAN_POINT('Ctrl Pts',(-1.97406280235188,1.,0.162079693556288));
#33803=CARTESIAN_POINT('Ctrl Pts',(-1.96816512677967,1.,0.163478185457734));
#33804=CARTESIAN_POINT('Ctrl Pts',(-1.96229379940136,1.,0.164816568920269));
#33805=CARTESIAN_POINT('Ctrl Pts',(-1.9564675971873,1.,0.166093592002812));
#33806=CARTESIAN_POINT('Ctrl Pts',(-1.95069027794294,1.,0.167307501784475));
#33807=CARTESIAN_POINT('Ctrl Pts',(-1.94493757756931,1.,0.168455741607556));
#33808=CARTESIAN_POINT('Ctrl Pts',(-1.93915639211581,1.,0.169534904817491));
#33809=CARTESIAN_POINT('Ctrl Pts',(-1.93329183155539,1.,0.170541253116201));
#33810=CARTESIAN_POINT('Ctrl Pts',(-1.92731093582036,1.,0.171471191532988));
#33811=CARTESIAN_POINT('Ctrl Pts',(-1.9212233439798,1.,0.172321621259514));
#33812=CARTESIAN_POINT('Ctrl Pts',(-1.91511429159527,1.,0.173090695383496));
#33813=CARTESIAN_POINT('Ctrl Pts',(-1.90911693975267,1.,0.173776635257817));
#33814=CARTESIAN_POINT('Ctrl Pts',(-1.90335253862834,1.,0.174375518661085));
#33815=CARTESIAN_POINT('Ctrl Pts',(-1.89788101117132,1.,0.174879405091263));
#33816=CARTESIAN_POINT('Ctrl Pts',(-1.892646301985,1.,0.175274276190844));
#33817=CARTESIAN_POINT('Ctrl Pts',(-1.88742606273259,1.,0.175538155840648));
#33818=CARTESIAN_POINT('Ctrl Pts',(-1.88188663145367,1.,0.175644148889698));
#33819=CARTESIAN_POINT('Ctrl Pts',(-1.87563767773588,1.,0.175563480746485));
#33820=CARTESIAN_POINT('Ctrl Pts',(-1.86828349694799,1.,0.175268337590758));
#33821=CARTESIAN_POINT('Ctrl Pts',(-1.85948367088837,1.,0.17473525927603));
#33822=CARTESIAN_POINT('Ctrl Pts',(-1.8489811319852,1.,0.173946627587731));
#33823=CARTESIAN_POINT('Ctrl Pts',(-1.83658380527692,1.,0.1728894428919));
#33824=CARTESIAN_POINT('Ctrl Pts',(-1.82215766811545,1.,0.171554770204119));
#33825=CARTESIAN_POINT('Ctrl Pts',(-1.80561530629706,1.,0.169936923904608));
#33826=CARTESIAN_POINT('Ctrl Pts',(-1.7869064998507,1.,0.168032772805197));
#33827=CARTESIAN_POINT('Ctrl Pts',(-1.77018771684844,1.,0.1662793551464));
#33828=CARTESIAN_POINT('Ctrl Pts',(-1.75666056638427,1.,0.164834765707158));
#33829=CARTESIAN_POINT('Ctrl Pts',(-1.7472034950333,1.,0.163814161002002));
#33830=CARTESIAN_POINT('Ctrl Pts',(-1.74236521665491,1.,0.163289472382896));
#33831=CARTESIAN_POINT('',(-2.19890268624765,0.,0.069476445021958));
#33832=CARTESIAN_POINT('Origin',(-2.19890268624765,0.,-0.0694764450219585));
#33833=CARTESIAN_POINT('',(-2.19890268624765,1.,-0.0694764450219585));
#33834=CARTESIAN_POINT('',(-2.19890268624765,1.,0.069476445021958));
#33835=CARTESIAN_POINT('',(-2.19890268624765,0.,-0.0694764450219585));
#33836=CARTESIAN_POINT('Ctrl Pts',(-1.74236521665491,-1.,-0.163289472382896));
#33837=CARTESIAN_POINT('Ctrl Pts',(-1.74236521665491,1.,-0.163289472382896));
#33838=CARTESIAN_POINT('Ctrl Pts',(-1.74720349503904,-1.,-0.163814161002474));
#33839=CARTESIAN_POINT('Ctrl Pts',(-1.74720349503904,1.,-0.163814161002474));
#33840=CARTESIAN_POINT('Ctrl Pts',(-1.75666056640041,-1.,-0.164834765708484));
#33841=CARTESIAN_POINT('Ctrl Pts',(-1.75666056640041,1.,-0.164834765708484));
#33842=CARTESIAN_POINT('Ctrl Pts',(-1.77018771687692,-1.,-0.166279355148738));
#33843=CARTESIAN_POINT('Ctrl Pts',(-1.77018771687692,1.,-0.166279355148738));
#33844=CARTESIAN_POINT('Ctrl Pts',(-1.78690649988931,-1.,-0.16803277280837));
#33845=CARTESIAN_POINT('Ctrl Pts',(-1.78690649988931,1.,-0.16803277280837));
#33846=CARTESIAN_POINT('Ctrl Pts',(-1.80561530633924,-1.,-0.169936923908078));
#33847=CARTESIAN_POINT('Ctrl Pts',(-1.80561530633924,1.,-0.169936923908078));
#33848=CARTESIAN_POINT('Ctrl Pts',(-1.82215766815414,-1.,-0.171554770207306));
#33849=CARTESIAN_POINT('Ctrl Pts',(-1.82215766815414,1.,-0.171554770207306));
#33850=CARTESIAN_POINT('Ctrl Pts',(-1.83658380530747,-1.,-0.17288944289442));
#33851=CARTESIAN_POINT('Ctrl Pts',(-1.83658380530747,1.,-0.17288944289442));
#33852=CARTESIAN_POINT('Ctrl Pts',(-1.84898113200543,-1.,-0.173946627589401));
#33853=CARTESIAN_POINT('Ctrl Pts',(-1.84898113200543,1.,-0.173946627589401));
#33854=CARTESIAN_POINT('Ctrl Pts',(-1.85948367089838,-1.,-0.174735259276856));
#33855=CARTESIAN_POINT('Ctrl Pts',(-1.85948367089838,1.,-0.174735259276856));
#33856=CARTESIAN_POINT('Ctrl Pts',(-1.86828349694972,-1.,-0.175268337590901));
#33857=CARTESIAN_POINT('Ctrl Pts',(-1.86828349694972,1.,-0.175268337590901));
#33858=CARTESIAN_POINT('Ctrl Pts',(-1.87563767773249,-1.,-0.175563480746205));
#33859=CARTESIAN_POINT('Ctrl Pts',(-1.87563767773249,1.,-0.175563480746205));
#33860=CARTESIAN_POINT('Ctrl Pts',(-1.88188663144846,-1.,-0.175644148889271));
#33861=CARTESIAN_POINT('Ctrl Pts',(-1.88188663144846,1.,-0.175644148889271));
#33862=CARTESIAN_POINT('Ctrl Pts',(-1.88742606272818,-1.,-0.175538155840286));
#33863=CARTESIAN_POINT('Ctrl Pts',(-1.88742606272818,1.,-0.175538155840286));
#33864=CARTESIAN_POINT('Ctrl Pts',(-1.89264630198279,-1.,-0.175274276190664));
#33865=CARTESIAN_POINT('Ctrl Pts',(-1.89264630198279,1.,-0.175274276190664));
#33866=CARTESIAN_POINT('Ctrl Pts',(-1.89788101117148,-1.,-0.174879405091277));
#33867=CARTESIAN_POINT('Ctrl Pts',(-1.89788101117148,1.,-0.174879405091277));
#33868=CARTESIAN_POINT('Ctrl Pts',(-1.90335253863003,-1.,-0.174375518661222));
#33869=CARTESIAN_POINT('Ctrl Pts',(-1.90335253863003,1.,-0.174375518661222));
#33870=CARTESIAN_POINT('Ctrl Pts',(-1.90911693975475,-1.,-0.173776635257984));
#33871=CARTESIAN_POINT('Ctrl Pts',(-1.90911693975475,1.,-0.173776635257984));
#33872=CARTESIAN_POINT('Ctrl Pts',(-1.91511429159681,-1.,-0.173090695383619));
#33873=CARTESIAN_POINT('Ctrl Pts',(-1.91511429159681,1.,-0.173090695383619));
#33874=CARTESIAN_POINT('Ctrl Pts',(-1.92122334398034,-1.,-0.172321621259557));
#33875=CARTESIAN_POINT('Ctrl Pts',(-1.92122334398034,1.,-0.172321621259557));
#33876=CARTESIAN_POINT('Ctrl Pts',(-1.92731093582,-1.,-0.17147119153296));
#33877=CARTESIAN_POINT('Ctrl Pts',(-1.92731093582,1.,-0.17147119153296));
#33878=CARTESIAN_POINT('Ctrl Pts',(-1.93329183155455,-1.,-0.170541253116136));
#33879=CARTESIAN_POINT('Ctrl Pts',(-1.93329183155455,1.,-0.170541253116136));
#33880=CARTESIAN_POINT('Ctrl Pts',(-1.93915639211497,-1.,-0.169534904817425));
#33881=CARTESIAN_POINT('Ctrl Pts',(-1.93915639211497,1.,-0.169534904817425));
#33882=CARTESIAN_POINT('Ctrl Pts',(-1.94493757756879,-1.,-0.168455741607516));
#33883=CARTESIAN_POINT('Ctrl Pts',(-1.94493757756879,1.,-0.168455741607516));
#33884=CARTESIAN_POINT('Ctrl Pts',(-1.95069027794286,-1.,-0.167307501784469));
#33885=CARTESIAN_POINT('Ctrl Pts',(-1.95069027794286,1.,-0.167307501784469));
#33886=CARTESIAN_POINT('Ctrl Pts',(-1.95646759718755,-1.,-0.166093592002833));
#33887=CARTESIAN_POINT('Ctrl Pts',(-1.95646759718755,1.,-0.166093592002833));
#33888=CARTESIAN_POINT('Ctrl Pts',(-1.96229379940174,-1.,-0.1648165689203));
#33889=CARTESIAN_POINT('Ctrl Pts',(-1.96229379940174,1.,-0.1648165689203));
#33890=CARTESIAN_POINT('Ctrl Pts',(-1.96816512678,-1.,-0.16347818545776));
#33891=CARTESIAN_POINT('Ctrl Pts',(-1.96816512678,1.,-0.16347818545776));
#33892=CARTESIAN_POINT('Ctrl Pts',(-1.97406280235204,-1.,-0.162079693556302));
#33893=CARTESIAN_POINT('Ctrl Pts',(-1.97406280235204,1.,-0.162079693556302));
#33894=CARTESIAN_POINT('Ctrl Pts',(-1.97996195437557,-1.,-0.16062206078461));
#33895=CARTESIAN_POINT('Ctrl Pts',(-1.97996195437557,1.,-0.16062206078461));
#33896=CARTESIAN_POINT('Ctrl Pts',(-1.98584238283279,-1.,-0.159106226437289));
#33897=CARTESIAN_POINT('Ctrl Pts',(-1.98584238283279,1.,-0.159106226437289));
#33898=CARTESIAN_POINT('Ctrl Pts',(-1.99169810931893,-1.,-0.157533331459215));
#33899=CARTESIAN_POINT('Ctrl Pts',(-1.99169810931893,1.,-0.157533331459215));
#33900=CARTESIAN_POINT('Ctrl Pts',(-1.99753284771487,-1.,-0.155904629548775));
#33901=CARTESIAN_POINT('Ctrl Pts',(-1.99753284771487,1.,-0.155904629548775));
#33902=CARTESIAN_POINT('Ctrl Pts',(-2.00335565310539,-1.,-0.154221403049719));
#33903=CARTESIAN_POINT('Ctrl Pts',(-2.00335565310539,1.,-0.154221403049719));
#33904=CARTESIAN_POINT('Ctrl Pts',(-2.00917680318426,-1.,-0.152484883621452));
#33905=CARTESIAN_POINT('Ctrl Pts',(-2.00917680318426,1.,-0.152484883621452));
#33906=CARTESIAN_POINT('Ctrl Pts',(-2.01500291940243,-1.,-0.150696157673084));
#33907=CARTESIAN_POINT('Ctrl Pts',(-2.01500291940243,1.,-0.150696157673084));
#33908=CARTESIAN_POINT('Ctrl Pts',(-2.02083464969897,-1.,-0.148856124775343));
#33909=CARTESIAN_POINT('Ctrl Pts',(-2.02083464969897,1.,-0.148856124775343));
#33910=CARTESIAN_POINT('Ctrl Pts',(-2.02666926182017,-1.,-0.146965557332586));
#33911=CARTESIAN_POINT('Ctrl Pts',(-2.02666926182017,1.,-0.146965557332586));
#33912=CARTESIAN_POINT('Ctrl Pts',(-2.03250223739941,-1.,-0.145025140186058));
#33913=CARTESIAN_POINT('Ctrl Pts',(-2.03250223739941,1.,-0.145025140186058));
#33914=CARTESIAN_POINT('Ctrl Pts',(-2.03832911025913,-1.,-0.143035515058208));
#33915=CARTESIAN_POINT('Ctrl Pts',(-2.03832911025913,1.,-0.143035515058208));
#33916=CARTESIAN_POINT('Ctrl Pts',(-2.04414757947919,-1.,-0.140997332152545));
#33917=CARTESIAN_POINT('Ctrl Pts',(-2.04414757947919,1.,-0.140997332152545));
#33918=CARTESIAN_POINT('Ctrl Pts',(-2.04995762001333,-1.,-0.138911255368966));
#33919=CARTESIAN_POINT('Ctrl Pts',(-2.04995762001333,1.,-0.138911255368966));
#33920=CARTESIAN_POINT('Ctrl Pts',(-2.0557604441427,-1.,-0.136777941218044));
#33921=CARTESIAN_POINT('Ctrl Pts',(-2.0557604441427,1.,-0.136777941218044));
#33922=CARTESIAN_POINT('Ctrl Pts',(-2.06155781517844,-1.,-0.134598026192107));
#33923=CARTESIAN_POINT('Ctrl Pts',(-2.06155781517844,1.,-0.134598026192107));
#33924=CARTESIAN_POINT('Ctrl Pts',(-2.06735123910319,-1.,-0.13237211154771));
#33925=CARTESIAN_POINT('Ctrl Pts',(-2.06735123910319,1.,-0.13237211154771));
#33926=CARTESIAN_POINT('Ctrl Pts',(-2.07314114713047,-1.,-0.130100748328401));
#33927=CARTESIAN_POINT('Ctrl Pts',(-2.07314114713047,1.,-0.130100748328401));
#33928=CARTESIAN_POINT('Ctrl Pts',(-2.07892715110967,-1.,-0.127784445276116));
#33929=CARTESIAN_POINT('Ctrl Pts',(-2.07892715110967,1.,-0.127784445276116));
#33930=CARTESIAN_POINT('Ctrl Pts',(-2.08470840653628,-1.,-0.125423679412058));
#33931=CARTESIAN_POINT('Ctrl Pts',(-2.08470840653628,1.,-0.125423679412058));
#33932=CARTESIAN_POINT('Ctrl Pts',(-2.09048392424826,-1.,-0.123018905621083));
#33933=CARTESIAN_POINT('Ctrl Pts',(-2.09048392424826,1.,-0.123018905621083));
#33934=CARTESIAN_POINT('Ctrl Pts',(-2.09625292867756,-1.,-0.120570567965129));
#33935=CARTESIAN_POINT('Ctrl Pts',(-2.09625292867756,1.,-0.120570567965129));
#33936=CARTESIAN_POINT('Ctrl Pts',(-2.10201512132945,-1.,-0.118079107988368));
#33937=CARTESIAN_POINT('Ctrl Pts',(-2.10201512132945,1.,-0.118079107988368));
#33938=CARTESIAN_POINT('Ctrl Pts',(-2.10777050261359,-1.,-0.11554495768794));
#33939=CARTESIAN_POINT('Ctrl Pts',(-2.10777050261359,1.,-0.11554495768794));
#33940=CARTESIAN_POINT('Ctrl Pts',(-2.11351924490335,-1.,-0.112968534419746));
#33941=CARTESIAN_POINT('Ctrl Pts',(-2.11351924490335,1.,-0.112968534419746));
#33942=CARTESIAN_POINT('Ctrl Pts',(-2.11926155590849,-1.,-0.11035023613502));
#33943=CARTESIAN_POINT('Ctrl Pts',(-2.11926155590849,1.,-0.11035023613502));
#33944=CARTESIAN_POINT('Ctrl Pts',(-2.12499752306927,-1.,-0.107690435231068));
#33945=CARTESIAN_POINT('Ctrl Pts',(-2.12499752306927,1.,-0.107690435231068));
#33946=CARTESIAN_POINT('Ctrl Pts',(-2.1307270488718,-1.,-0.104989479152703));
#33947=CARTESIAN_POINT('Ctrl Pts',(-2.1307270488718,1.,-0.104989479152703));
#33948=CARTESIAN_POINT('Ctrl Pts',(-2.13644992667052,-1.,-0.102247700556064));
#33949=CARTESIAN_POINT('Ctrl Pts',(-2.13644992667052,1.,-0.102247700556064));
#33950=CARTESIAN_POINT('Ctrl Pts',(-2.14216588395974,-1.,-0.0994654261990744));
#33951=CARTESIAN_POINT('Ctrl Pts',(-2.14216588395974,1.,-0.0994654261990744));
#33952=CARTESIAN_POINT('Ctrl Pts',(-2.14787463531864,-1.,-0.096642985230569));
#33953=CARTESIAN_POINT('Ctrl Pts',(-2.14787463531864,1.,-0.096642985230569));
#33954=CARTESIAN_POINT('Ctrl Pts',(-2.15357593978377,-1.,-0.0937807218868346));
#33955=CARTESIAN_POINT('Ctrl Pts',(-2.15357593978377,1.,-0.0937807218868346));
#33956=CARTESIAN_POINT('Ctrl Pts',(-2.15926961544808,-1.,-0.0908789888108267));
#33957=CARTESIAN_POINT('Ctrl Pts',(-2.15926961544808,1.,-0.0908789888108267));
#33958=CARTESIAN_POINT('Ctrl Pts',(-2.16495552645275,-1.,-0.0879381291387824));
#33959=CARTESIAN_POINT('Ctrl Pts',(-2.16495552645275,1.,-0.0879381291387824));
#33960=CARTESIAN_POINT('Ctrl Pts',(-2.17063357871031,-1.,-0.0849584620835644));
#33961=CARTESIAN_POINT('Ctrl Pts',(-2.17063357871031,1.,-0.0849584620835644));
#33962=CARTESIAN_POINT('Ctrl Pts',(-2.1763037121106,-1.,-0.0819402680871941));
#33963=CARTESIAN_POINT('Ctrl Pts',(-2.1763037121106,1.,-0.0819402680871941));
#33964=CARTESIAN_POINT('Ctrl Pts',(-2.18196589448304,-1.,-0.0788837727683229));
#33965=CARTESIAN_POINT('Ctrl Pts',(-2.18196589448304,1.,-0.0788837727683229));
#33966=CARTESIAN_POINT('Ctrl Pts',(-2.1876201139874,-1.,-0.0757891465833413));
#33967=CARTESIAN_POINT('Ctrl Pts',(-2.1876201139874,1.,-0.0757891465833413));
#33968=CARTESIAN_POINT('Ctrl Pts',(-2.19213712012956,-1.,-0.0732830357304277));
#33969=CARTESIAN_POINT('Ctrl Pts',(-2.19213712012956,1.,-0.0732830357304277));
#33970=CARTESIAN_POINT('Ctrl Pts',(-2.19552129483562,-1.,-0.0713863779524629));
#33971=CARTESIAN_POINT('Ctrl Pts',(-2.19552129483562,1.,-0.0713863779524629));
#33972=CARTESIAN_POINT('Ctrl Pts',(-2.19777582085261,-1.,-0.0701143536324927));
#33973=CARTESIAN_POINT('Ctrl Pts',(-2.19777582085261,1.,-0.0701143536324927));
#33974=CARTESIAN_POINT('Ctrl Pts',(-2.19890268624765,-1.,-0.0694764450219585));
#33975=CARTESIAN_POINT('Ctrl Pts',(-2.19890268624765,1.,-0.0694764450219585));
#33976=CARTESIAN_POINT('',(-1.74236521665491,1.,-0.163289472382896));
#33977=CARTESIAN_POINT('Ctrl Pts',(-1.74236521665491,1.,-0.163289472382896));
#33978=CARTESIAN_POINT('Ctrl Pts',(-1.74720349503904,1.,-0.163814161002474));
#33979=CARTESIAN_POINT('Ctrl Pts',(-1.75666056640041,1.,-0.164834765708484));
#33980=CARTESIAN_POINT('Ctrl Pts',(-1.77018771687692,1.,-0.166279355148738));
#33981=CARTESIAN_POINT('Ctrl Pts',(-1.78690649988931,1.,-0.16803277280837));
#33982=CARTESIAN_POINT('Ctrl Pts',(-1.80561530633924,1.,-0.169936923908078));
#33983=CARTESIAN_POINT('Ctrl Pts',(-1.82215766815414,1.,-0.171554770207306));
#33984=CARTESIAN_POINT('Ctrl Pts',(-1.83658380530747,1.,-0.17288944289442));
#33985=CARTESIAN_POINT('Ctrl Pts',(-1.84898113200543,1.,-0.173946627589401));
#33986=CARTESIAN_POINT('Ctrl Pts',(-1.85948367089838,1.,-0.174735259276856));
#33987=CARTESIAN_POINT('Ctrl Pts',(-1.86828349694972,1.,-0.175268337590901));
#33988=CARTESIAN_POINT('Ctrl Pts',(-1.87563767773249,1.,-0.175563480746205));
#33989=CARTESIAN_POINT('Ctrl Pts',(-1.88188663144846,1.,-0.175644148889271));
#33990=CARTESIAN_POINT('Ctrl Pts',(-1.88742606272818,1.,-0.175538155840286));
#33991=CARTESIAN_POINT('Ctrl Pts',(-1.89264630198279,1.,-0.175274276190664));
#33992=CARTESIAN_POINT('Ctrl Pts',(-1.89788101117148,1.,-0.174879405091277));
#33993=CARTESIAN_POINT('Ctrl Pts',(-1.90335253863003,1.,-0.174375518661222));
#33994=CARTESIAN_POINT('Ctrl Pts',(-1.90911693975475,1.,-0.173776635257984));
#33995=CARTESIAN_POINT('Ctrl Pts',(-1.91511429159681,1.,-0.173090695383619));
#33996=CARTESIAN_POINT('Ctrl Pts',(-1.92122334398034,1.,-0.172321621259557));
#33997=CARTESIAN_POINT('Ctrl Pts',(-1.92731093582,1.,-0.17147119153296));
#33998=CARTESIAN_POINT('Ctrl Pts',(-1.93329183155455,1.,-0.170541253116136));
#33999=CARTESIAN_POINT('Ctrl Pts',(-1.93915639211497,1.,-0.169534904817425));
#34000=CARTESIAN_POINT('Ctrl Pts',(-1.94493757756879,1.,-0.168455741607516));
#34001=CARTESIAN_POINT('Ctrl Pts',(-1.95069027794286,1.,-0.167307501784469));
#34002=CARTESIAN_POINT('Ctrl Pts',(-1.95646759718755,1.,-0.166093592002833));
#34003=CARTESIAN_POINT('Ctrl Pts',(-1.96229379940174,1.,-0.1648165689203));
#34004=CARTESIAN_POINT('Ctrl Pts',(-1.96816512678,1.,-0.16347818545776));
#34005=CARTESIAN_POINT('Ctrl Pts',(-1.97406280235204,1.,-0.162079693556302));
#34006=CARTESIAN_POINT('Ctrl Pts',(-1.97996195437557,1.,-0.16062206078461));
#34007=CARTESIAN_POINT('Ctrl Pts',(-1.98584238283279,1.,-0.159106226437289));
#34008=CARTESIAN_POINT('Ctrl Pts',(-1.99169810931893,1.,-0.157533331459215));
#34009=CARTESIAN_POINT('Ctrl Pts',(-1.99753284771487,1.,-0.155904629548775));
#34010=CARTESIAN_POINT('Ctrl Pts',(-2.00335565310539,1.,-0.154221403049719));
#34011=CARTESIAN_POINT('Ctrl Pts',(-2.00917680318426,1.,-0.152484883621452));
#34012=CARTESIAN_POINT('Ctrl Pts',(-2.01500291940243,1.,-0.150696157673084));
#34013=CARTESIAN_POINT('Ctrl Pts',(-2.02083464969897,1.,-0.148856124775343));
#34014=CARTESIAN_POINT('Ctrl Pts',(-2.02666926182017,1.,-0.146965557332586));
#34015=CARTESIAN_POINT('Ctrl Pts',(-2.03250223739941,1.,-0.145025140186058));
#34016=CARTESIAN_POINT('Ctrl Pts',(-2.03832911025913,1.,-0.143035515058208));
#34017=CARTESIAN_POINT('Ctrl Pts',(-2.04414757947919,1.,-0.140997332152545));
#34018=CARTESIAN_POINT('Ctrl Pts',(-2.04995762001333,1.,-0.138911255368966));
#34019=CARTESIAN_POINT('Ctrl Pts',(-2.0557604441427,1.,-0.136777941218044));
#34020=CARTESIAN_POINT('Ctrl Pts',(-2.06155781517844,1.,-0.134598026192107));
#34021=CARTESIAN_POINT('Ctrl Pts',(-2.06735123910319,1.,-0.13237211154771));
#34022=CARTESIAN_POINT('Ctrl Pts',(-2.07314114713047,1.,-0.130100748328401));
#34023=CARTESIAN_POINT('Ctrl Pts',(-2.07892715110967,1.,-0.127784445276116));
#34024=CARTESIAN_POINT('Ctrl Pts',(-2.08470840653628,1.,-0.125423679412058));
#34025=CARTESIAN_POINT('Ctrl Pts',(-2.09048392424826,1.,-0.123018905621083));
#34026=CARTESIAN_POINT('Ctrl Pts',(-2.09625292867756,1.,-0.120570567965129));
#34027=CARTESIAN_POINT('Ctrl Pts',(-2.10201512132945,1.,-0.118079107988368));
#34028=CARTESIAN_POINT('Ctrl Pts',(-2.10777050261359,1.,-0.11554495768794));
#34029=CARTESIAN_POINT('Ctrl Pts',(-2.11351924490335,1.,-0.112968534419746));
#34030=CARTESIAN_POINT('Ctrl Pts',(-2.11926155590849,1.,-0.11035023613502));
#34031=CARTESIAN_POINT('Ctrl Pts',(-2.12499752306927,1.,-0.107690435231068));
#34032=CARTESIAN_POINT('Ctrl Pts',(-2.1307270488718,1.,-0.104989479152703));
#34033=CARTESIAN_POINT('Ctrl Pts',(-2.13644992667052,1.,-0.102247700556064));
#34034=CARTESIAN_POINT('Ctrl Pts',(-2.14216588395974,1.,-0.0994654261990744));
#34035=CARTESIAN_POINT('Ctrl Pts',(-2.14787463531864,1.,-0.096642985230569));
#34036=CARTESIAN_POINT('Ctrl Pts',(-2.15357593978377,1.,-0.0937807218868346));
#34037=CARTESIAN_POINT('Ctrl Pts',(-2.15926961544808,1.,-0.0908789888108267));
#34038=CARTESIAN_POINT('Ctrl Pts',(-2.16495552645275,1.,-0.0879381291387824));
#34039=CARTESIAN_POINT('Ctrl Pts',(-2.17063357871031,1.,-0.0849584620835644));
#34040=CARTESIAN_POINT('Ctrl Pts',(-2.1763037121106,1.,-0.0819402680871941));
#34041=CARTESIAN_POINT('Ctrl Pts',(-2.18196589448304,1.,-0.0788837727683229));
#34042=CARTESIAN_POINT('Ctrl Pts',(-2.1876201139874,1.,-0.0757891465833413));
#34043=CARTESIAN_POINT('Ctrl Pts',(-2.19213712012956,1.,-0.0732830357304277));
#34044=CARTESIAN_POINT('Ctrl Pts',(-2.19552129483562,1.,-0.0713863779524629));
#34045=CARTESIAN_POINT('Ctrl Pts',(-2.19777582085261,1.,-0.0701143536324927));
#34046=CARTESIAN_POINT('Ctrl Pts',(-2.19890268624765,1.,-0.0694764450219585));
#34047=CARTESIAN_POINT('',(-1.74236521665491,0.,-0.163289472382896));
#34048=CARTESIAN_POINT('Origin',(0.,0.,0.));
#34049=CARTESIAN_POINT('',(-1.7075470150345,1.,-0.383122945602004));
#34050=CARTESIAN_POINT('Origin',(0.,1.,0.));
#34051=CARTESIAN_POINT('',(-1.7075470150345,0.,-0.383122945602004));
#34052=CARTESIAN_POINT('Ctrl Pts',(-2.11275013067528,-1.,-0.61342227326009));
#34053=CARTESIAN_POINT('Ctrl Pts',(-2.11275013067528,1.,-0.61342227326009));
#34054=CARTESIAN_POINT('Ctrl Pts',(-2.11187554260142,-1.,-0.61246736556225));
#34055=CARTESIAN_POINT('Ctrl Pts',(-2.11187554260142,1.,-0.61246736556225));
#34056=CARTESIAN_POINT('Ctrl Pts',(-2.11012443807661,-1.,-0.610560911691113));
#34057=CARTESIAN_POINT('Ctrl Pts',(-2.11012443807661,1.,-0.610560911691113));
#34058=CARTESIAN_POINT('Ctrl Pts',(-2.10749199615859,-1.,-0.607711315456826));
#34059=CARTESIAN_POINT('Ctrl Pts',(-2.10749199615859,1.,-0.607711315456826));
#34060=CARTESIAN_POINT('Ctrl Pts',(-2.10397049887709,-1.,-0.603932030738212));
#34061=CARTESIAN_POINT('Ctrl Pts',(-2.10397049887709,1.,-0.603932030738212));
#34062=CARTESIAN_POINT('Ctrl Pts',(-2.09954930865331,-1.,-0.599241616422144));
#34063=CARTESIAN_POINT('Ctrl Pts',(-2.09954930865331,1.,-0.599241616422144));
#34064=CARTESIAN_POINT('Ctrl Pts',(-2.09510876220501,-1.,-0.594585006052823));
#34065=CARTESIAN_POINT('Ctrl Pts',(-2.09510876220501,1.,-0.594585006052823));
#34066=CARTESIAN_POINT('Ctrl Pts',(-2.09064881812053,-1.,-0.589962365403189));
#34067=CARTESIAN_POINT('Ctrl Pts',(-2.09064881812053,1.,-0.589962365403189));
#34068=CARTESIAN_POINT('Ctrl Pts',(-2.086169437277,-1.,-0.585373918990895));
#34069=CARTESIAN_POINT('Ctrl Pts',(-2.086169437277,1.,-0.585373918990895));
#34070=CARTESIAN_POINT('Ctrl Pts',(-2.08167059018138,-1.,-0.580819952107257));
#34071=CARTESIAN_POINT('Ctrl Pts',(-2.08167059018138,1.,-0.580819952107257));
#34072=CARTESIAN_POINT('Ctrl Pts',(-2.07715226767361,-1.,-0.576300797416274));
#34073=CARTESIAN_POINT('Ctrl Pts',(-2.07715226767361,1.,-0.576300797416274));
#34074=CARTESIAN_POINT('Ctrl Pts',(-2.07261449292757,-1.,-0.571816823242411));
#34075=CARTESIAN_POINT('Ctrl Pts',(-2.07261449292757,1.,-0.571816823242411));
#34076=CARTESIAN_POINT('Ctrl Pts',(-2.06805732997383,-1.,-0.567368421181229));
#34077=CARTESIAN_POINT('Ctrl Pts',(-2.06805732997383,1.,-0.567368421181229));
#34078=CARTESIAN_POINT('Ctrl Pts',(-2.06348090160697,-1.,-0.562955993082574));
#34079=CARTESIAN_POINT('Ctrl Pts',(-2.06348090160697,1.,-0.562955993082574));
#34080=CARTESIAN_POINT('Ctrl Pts',(-2.05888537756571,-1.,-0.558579940185467));
#34081=CARTESIAN_POINT('Ctrl Pts',(-2.05888537756571,1.,-0.558579940185467));
#34082=CARTESIAN_POINT('Ctrl Pts',(-2.05427091604482,-1.,-0.554240657464109));
#34083=CARTESIAN_POINT('Ctrl Pts',(-2.05427091604482,1.,-0.554240657464109));
#34084=CARTESIAN_POINT('Ctrl Pts',(-2.04963761077974,-1.,-0.549938525150342));
#34085=CARTESIAN_POINT('Ctrl Pts',(-2.04963761077974,1.,-0.549938525150342));
#34086=CARTESIAN_POINT('Ctrl Pts',(-2.0449854471456,-1.,-0.545673903817348));
#34087=CARTESIAN_POINT('Ctrl Pts',(-2.0449854471456,1.,-0.545673903817348));
#34088=CARTESIAN_POINT('Ctrl Pts',(-2.0403142269048,-1.,-0.54144712061552));
#34089=CARTESIAN_POINT('Ctrl Pts',(-2.0403142269048,1.,-0.54144712061552));
#34090=CARTESIAN_POINT('Ctrl Pts',(-2.03562362953993,-1.,-0.537258489833134));
#34091=CARTESIAN_POINT('Ctrl Pts',(-2.03562362953993,1.,-0.537258489833134));
#34092=CARTESIAN_POINT('Ctrl Pts',(-2.03091336214401,-1.,-0.533108355132905));
#34093=CARTESIAN_POINT('Ctrl Pts',(-2.03091336214401,1.,-0.533108355132905));
#34094=CARTESIAN_POINT('Ctrl Pts',(-2.02618329083289,-1.,-0.52899712724191));
#34095=CARTESIAN_POINT('Ctrl Pts',(-2.02618329083289,1.,-0.52899712724191));
#34096=CARTESIAN_POINT('Ctrl Pts',(-2.02143356304712,-1.,-0.524925318333518));
#34097=CARTESIAN_POINT('Ctrl Pts',(-2.02143356304712,1.,-0.524925318333518));
#34098=CARTESIAN_POINT('Ctrl Pts',(-2.01666477917305,-1.,-0.520893590399428));
#34099=CARTESIAN_POINT('Ctrl Pts',(-2.01666477917305,1.,-0.520893590399428));
#34100=CARTESIAN_POINT('Ctrl Pts',(-2.01187773939257,-1.,-0.516902681728733));
#34101=CARTESIAN_POINT('Ctrl Pts',(-2.01187773939257,1.,-0.516902681728733));
#34102=CARTESIAN_POINT('Ctrl Pts',(-2.00707309946955,-1.,-0.512953306961813));
#34103=CARTESIAN_POINT('Ctrl Pts',(-2.00707309946955,1.,-0.512953306961813));
#34104=CARTESIAN_POINT('Ctrl Pts',(-2.00225107134733,-1.,-0.509046069886152));
#34105=CARTESIAN_POINT('Ctrl Pts',(-2.00225107134733,1.,-0.509046069886152));
#34106=CARTESIAN_POINT('Ctrl Pts',(-1.99741107463567,-1.,-0.505181361323011));
#34107=CARTESIAN_POINT('Ctrl Pts',(-1.99741107463567,1.,-0.505181361323011));
#34108=CARTESIAN_POINT('Ctrl Pts',(-1.9925514912615,-1.,-0.501359287727129));
#34109=CARTESIAN_POINT('Ctrl Pts',(-1.9925514912615,1.,-0.501359287727129));
#34110=CARTESIAN_POINT('Ctrl Pts',(-1.98767044752929,-1.,-0.497579909545564));
#34111=CARTESIAN_POINT('Ctrl Pts',(-1.98767044752929,1.,-0.497579909545564));
#34112=CARTESIAN_POINT('Ctrl Pts',(-1.9827665876182,-1.,-0.493843476541492));
#34113=CARTESIAN_POINT('Ctrl Pts',(-1.9827665876182,1.,-0.493843476541492));
#34114=CARTESIAN_POINT('Ctrl Pts',(-1.97783973019229,-1.,-0.490150627860955));
#34115=CARTESIAN_POINT('Ctrl Pts',(-1.97783973019229,1.,-0.490150627860955));
#34116=CARTESIAN_POINT('Ctrl Pts',(-1.97289186263272,-1.,-0.486502692907661));
#34117=CARTESIAN_POINT('Ctrl Pts',(-1.97289186263272,1.,-0.486502692907661));
#34118=CARTESIAN_POINT('Ctrl Pts',(-1.96792703422358,-1.,-0.482901662120686));
#34119=CARTESIAN_POINT('Ctrl Pts',(-1.96792703422358,1.,-0.482901662120686));
#34120=CARTESIAN_POINT('Ctrl Pts',(-1.96294933055938,-1.,-0.479349583074846));
#34121=CARTESIAN_POINT('Ctrl Pts',(-1.96294933055938,1.,-0.479349583074846));
#34122=CARTESIAN_POINT('Ctrl Pts',(-1.95796111148175,-1.,-0.475848034683171));
#34123=CARTESIAN_POINT('Ctrl Pts',(-1.95796111148175,1.,-0.475848034683171));
#34124=CARTESIAN_POINT('Ctrl Pts',(-1.95296148278136,-1.,-0.472397672264079));
#34125=CARTESIAN_POINT('Ctrl Pts',(-1.95296148278136,1.,-0.472397672264079));
#34126=CARTESIAN_POINT('Ctrl Pts',(-1.94794381136524,-1.,-0.468997482913158));
#34127=CARTESIAN_POINT('Ctrl Pts',(-1.94794381136524,1.,-0.468997482913158));
#34128=CARTESIAN_POINT('Ctrl Pts',(-1.94289794196205,-1.,-0.465645462026064));
#34129=CARTESIAN_POINT('Ctrl Pts',(-1.94289794196205,1.,-0.465645462026064));
#34130=CARTESIAN_POINT('Ctrl Pts',(-1.93781486640834,-1.,-0.462340031009087));
#34131=CARTESIAN_POINT('Ctrl Pts',(-1.93781486640834,1.,-0.462340031009087));
#34132=CARTESIAN_POINT('Ctrl Pts',(-1.93269066517936,-1.,-0.459081234547931));
#34133=CARTESIAN_POINT('Ctrl Pts',(-1.93269066517936,1.,-0.459081234547931));
#34134=CARTESIAN_POINT('Ctrl Pts',(-1.92753067150461,-1.,-0.455872005174335));
#34135=CARTESIAN_POINT('Ctrl Pts',(-1.92753067150461,1.,-0.455872005174335));
#34136=CARTESIAN_POINT('Ctrl Pts',(-1.9223538064847,-1.,-0.452719478359356));
#34137=CARTESIAN_POINT('Ctrl Pts',(-1.9223538064847,1.,-0.452719478359356));
#34138=CARTESIAN_POINT('Ctrl Pts',(-1.91718342555717,-1.,-0.449632260106572));
#34139=CARTESIAN_POINT('Ctrl Pts',(-1.91718342555717,1.,-0.449632260106572));
#34140=CARTESIAN_POINT('Ctrl Pts',(-1.91203699981095,-1.,-0.446617343485651));
#34141=CARTESIAN_POINT('Ctrl Pts',(-1.91203699981095,1.,-0.446617343485651));
#34142=CARTESIAN_POINT('Ctrl Pts',(-1.90691756144906,-1.,-0.44367755684917));
#34143=CARTESIAN_POINT('Ctrl Pts',(-1.90691756144906,1.,-0.44367755684917));
#34144=CARTESIAN_POINT('Ctrl Pts',(-1.90180124389137,-1.,-0.44080783370416));
#34145=CARTESIAN_POINT('Ctrl Pts',(-1.90180124389137,1.,-0.44080783370416));
#34146=CARTESIAN_POINT('Ctrl Pts',(-1.89663648956549,-1.,-0.437995003948443));
#34147=CARTESIAN_POINT('Ctrl Pts',(-1.89663648956549,1.,-0.437995003948443));
#34148=CARTESIAN_POINT('Ctrl Pts',(-1.89136993975585,-1.,-0.43522566096358));
#34149=CARTESIAN_POINT('Ctrl Pts',(-1.89136993975585,1.,-0.43522566096358));
#34150=CARTESIAN_POINT('Ctrl Pts',(-1.88596913666828,-1.,-0.432493038548833));
#34151=CARTESIAN_POINT('Ctrl Pts',(-1.88596913666828,1.,-0.432493038548833));
#34152=CARTESIAN_POINT('Ctrl Pts',(-1.88044229001778,-1.,-0.429803062482217));
#34153=CARTESIAN_POINT('Ctrl Pts',(-1.88044229001778,1.,-0.429803062482217));
#34154=CARTESIAN_POINT('Ctrl Pts',(-1.87486989291333,-1.,-0.427183828518743));
#34155=CARTESIAN_POINT('Ctrl Pts',(-1.87486989291333,1.,-0.427183828518743));
#34156=CARTESIAN_POINT('Ctrl Pts',(-1.8693780394412,-1.,-0.424678177290876));
#34157=CARTESIAN_POINT('Ctrl Pts',(-1.8693780394412,1.,-0.424678177290876));
#34158=CARTESIAN_POINT('Ctrl Pts',(-1.86408083333863,-1.,-0.422327307417884));
#34159=CARTESIAN_POINT('Ctrl Pts',(-1.86408083333863,1.,-0.422327307417884));
#34160=CARTESIAN_POINT('Ctrl Pts',(-1.8590328109667,-1.,-0.420157287975583));
#34161=CARTESIAN_POINT('Ctrl Pts',(-1.8590328109667,1.,-0.420157287975583));
#34162=CARTESIAN_POINT('Ctrl Pts',(-1.8541763285645,-1.,-0.418164129144045));
#34163=CARTESIAN_POINT('Ctrl Pts',(-1.8541763285645,1.,-0.418164129144045));
#34164=CARTESIAN_POINT('Ctrl Pts',(-1.84929312930314,-1.,-0.416300022039885));
#34165=CARTESIAN_POINT('Ctrl Pts',(-1.84929312930314,1.,-0.416300022039885));
#34166=CARTESIAN_POINT('Ctrl Pts',(-1.84405757074218,-1.,-0.414487438255542));
#34167=CARTESIAN_POINT('Ctrl Pts',(-1.84405757074218,1.,-0.414487438255542));
#34168=CARTESIAN_POINT('Ctrl Pts',(-1.8380895347617,-1.,-0.412633125322945));
#34169=CARTESIAN_POINT('Ctrl Pts',(-1.8380895347617,1.,-0.412633125322945));
#34170=CARTESIAN_POINT('Ctrl Pts',(-1.83100408895047,-1.,-0.410641256301276));
#34171=CARTESIAN_POINT('Ctrl Pts',(-1.83100408895047,1.,-0.410641256301276));
#34172=CARTESIAN_POINT('Ctrl Pts',(-1.82247022677562,-1.,-0.408428948106227));
#34173=CARTESIAN_POINT('Ctrl Pts',(-1.82247022677562,1.,-0.408428948106227));
#34174=CARTESIAN_POINT('Ctrl Pts',(-1.81223801812013,-1.,-0.405933518407175));
#34175=CARTESIAN_POINT('Ctrl Pts',(-1.81223801812013,1.,-0.405933518407175));
#34176=CARTESIAN_POINT('Ctrl Pts',(-1.80012077173238,-1.,-0.403107976163396));
#34177=CARTESIAN_POINT('Ctrl Pts',(-1.80012077173238,1.,-0.403107976163396));
#34178=CARTESIAN_POINT('Ctrl Pts',(-1.78598826343754,-1.,-0.399919403774155));
#34179=CARTESIAN_POINT('Ctrl Pts',(-1.78598826343754,1.,-0.399919403774155));
#34180=CARTESIAN_POINT('Ctrl Pts',(-1.76975560043442,-1.,-0.396346196110688));
#34181=CARTESIAN_POINT('Ctrl Pts',(-1.76975560043442,1.,-0.396346196110688));
#34182=CARTESIAN_POINT('Ctrl Pts',(-1.75137405310193,-1.,-0.392375812285395));
#34183=CARTESIAN_POINT('Ctrl Pts',(-1.75137405310193,1.,-0.392375812285395));
#34184=CARTESIAN_POINT('Ctrl Pts',(-1.73493170972829,-1.,-0.388877023502615));
#34185=CARTESIAN_POINT('Ctrl Pts',(-1.73493170972829,1.,-0.388877023502615));
#34186=CARTESIAN_POINT('Ctrl Pts',(-1.72162022244582,-1.,-0.386070790323281));
#34187=CARTESIAN_POINT('Ctrl Pts',(-1.72162022244582,1.,-0.386070790323281));
#34188=CARTESIAN_POINT('Ctrl Pts',(-1.71231062891398,-1.,-0.384119047314215));
#34189=CARTESIAN_POINT('Ctrl Pts',(-1.71231062891398,1.,-0.384119047314215));
#34190=CARTESIAN_POINT('Ctrl Pts',(-1.7075470150345,-1.,-0.383122945602004));
#34191=CARTESIAN_POINT('Ctrl Pts',(-1.7075470150345,1.,-0.383122945602004));
#34192=CARTESIAN_POINT('',(-2.11275013067528,1.,-0.61342227326009));
#34193=CARTESIAN_POINT('Ctrl Pts',(-2.11275013067528,1.,-0.61342227326009));
#34194=CARTESIAN_POINT('Ctrl Pts',(-2.11187554260142,1.,-0.61246736556225));
#34195=CARTESIAN_POINT('Ctrl Pts',(-2.11012443807661,1.,-0.610560911691113));
#34196=CARTESIAN_POINT('Ctrl Pts',(-2.10749199615859,1.,-0.607711315456826));
#34197=CARTESIAN_POINT('Ctrl Pts',(-2.10397049887709,1.,-0.603932030738212));
#34198=CARTESIAN_POINT('Ctrl Pts',(-2.09954930865331,1.,-0.599241616422144));
#34199=CARTESIAN_POINT('Ctrl Pts',(-2.09510876220501,1.,-0.594585006052823));
#34200=CARTESIAN_POINT('Ctrl Pts',(-2.09064881812053,1.,-0.589962365403189));
#34201=CARTESIAN_POINT('Ctrl Pts',(-2.086169437277,1.,-0.585373918990895));
#34202=CARTESIAN_POINT('Ctrl Pts',(-2.08167059018138,1.,-0.580819952107257));
#34203=CARTESIAN_POINT('Ctrl Pts',(-2.07715226767361,1.,-0.576300797416274));
#34204=CARTESIAN_POINT('Ctrl Pts',(-2.07261449292757,1.,-0.571816823242411));
#34205=CARTESIAN_POINT('Ctrl Pts',(-2.06805732997383,1.,-0.567368421181229));
#34206=CARTESIAN_POINT('Ctrl Pts',(-2.06348090160697,1.,-0.562955993082574));
#34207=CARTESIAN_POINT('Ctrl Pts',(-2.05888537756571,1.,-0.558579940185467));
#34208=CARTESIAN_POINT('Ctrl Pts',(-2.05427091604482,1.,-0.554240657464109));
#34209=CARTESIAN_POINT('Ctrl Pts',(-2.04963761077974,1.,-0.549938525150342));
#34210=CARTESIAN_POINT('Ctrl Pts',(-2.0449854471456,1.,-0.545673903817348));
#34211=CARTESIAN_POINT('Ctrl Pts',(-2.0403142269048,1.,-0.54144712061552));
#34212=CARTESIAN_POINT('Ctrl Pts',(-2.03562362953993,1.,-0.537258489833134));
#34213=CARTESIAN_POINT('Ctrl Pts',(-2.03091336214401,1.,-0.533108355132905));
#34214=CARTESIAN_POINT('Ctrl Pts',(-2.02618329083289,1.,-0.52899712724191));
#34215=CARTESIAN_POINT('Ctrl Pts',(-2.02143356304712,1.,-0.524925318333518));
#34216=CARTESIAN_POINT('Ctrl Pts',(-2.01666477917305,1.,-0.520893590399428));
#34217=CARTESIAN_POINT('Ctrl Pts',(-2.01187773939257,1.,-0.516902681728733));
#34218=CARTESIAN_POINT('Ctrl Pts',(-2.00707309946955,1.,-0.512953306961813));
#34219=CARTESIAN_POINT('Ctrl Pts',(-2.00225107134733,1.,-0.509046069886152));
#34220=CARTESIAN_POINT('Ctrl Pts',(-1.99741107463567,1.,-0.505181361323011));
#34221=CARTESIAN_POINT('Ctrl Pts',(-1.9925514912615,1.,-0.501359287727129));
#34222=CARTESIAN_POINT('Ctrl Pts',(-1.98767044752929,1.,-0.497579909545564));
#34223=CARTESIAN_POINT('Ctrl Pts',(-1.9827665876182,1.,-0.493843476541492));
#34224=CARTESIAN_POINT('Ctrl Pts',(-1.97783973019229,1.,-0.490150627860955));
#34225=CARTESIAN_POINT('Ctrl Pts',(-1.97289186263272,1.,-0.486502692907661));
#34226=CARTESIAN_POINT('Ctrl Pts',(-1.96792703422358,1.,-0.482901662120686));
#34227=CARTESIAN_POINT('Ctrl Pts',(-1.96294933055938,1.,-0.479349583074846));
#34228=CARTESIAN_POINT('Ctrl Pts',(-1.95796111148175,1.,-0.475848034683171));
#34229=CARTESIAN_POINT('Ctrl Pts',(-1.95296148278136,1.,-0.472397672264079));
#34230=CARTESIAN_POINT('Ctrl Pts',(-1.94794381136524,1.,-0.468997482913158));
#34231=CARTESIAN_POINT('Ctrl Pts',(-1.94289794196205,1.,-0.465645462026064));
#34232=CARTESIAN_POINT('Ctrl Pts',(-1.93781486640834,1.,-0.462340031009087));
#34233=CARTESIAN_POINT('Ctrl Pts',(-1.93269066517936,1.,-0.459081234547931));
#34234=CARTESIAN_POINT('Ctrl Pts',(-1.92753067150461,1.,-0.455872005174335));
#34235=CARTESIAN_POINT('Ctrl Pts',(-1.9223538064847,1.,-0.452719478359356));
#34236=CARTESIAN_POINT('Ctrl Pts',(-1.91718342555717,1.,-0.449632260106572));
#34237=CARTESIAN_POINT('Ctrl Pts',(-1.91203699981095,1.,-0.446617343485651));
#34238=CARTESIAN_POINT('Ctrl Pts',(-1.90691756144906,1.,-0.44367755684917));
#34239=CARTESIAN_POINT('Ctrl Pts',(-1.90180124389137,1.,-0.44080783370416));
#34240=CARTESIAN_POINT('Ctrl Pts',(-1.89663648956549,1.,-0.437995003948443));
#34241=CARTESIAN_POINT('Ctrl Pts',(-1.89136993975585,1.,-0.43522566096358));
#34242=CARTESIAN_POINT('Ctrl Pts',(-1.88596913666828,1.,-0.432493038548833));
#34243=CARTESIAN_POINT('Ctrl Pts',(-1.88044229001778,1.,-0.429803062482217));
#34244=CARTESIAN_POINT('Ctrl Pts',(-1.87486989291333,1.,-0.427183828518743));
#34245=CARTESIAN_POINT('Ctrl Pts',(-1.8693780394412,1.,-0.424678177290876));
#34246=CARTESIAN_POINT('Ctrl Pts',(-1.86408083333863,1.,-0.422327307417884));
#34247=CARTESIAN_POINT('Ctrl Pts',(-1.8590328109667,1.,-0.420157287975583));
#34248=CARTESIAN_POINT('Ctrl Pts',(-1.8541763285645,1.,-0.418164129144045));
#34249=CARTESIAN_POINT('Ctrl Pts',(-1.84929312930314,1.,-0.416300022039885));
#34250=CARTESIAN_POINT('Ctrl Pts',(-1.84405757074218,1.,-0.414487438255542));
#34251=CARTESIAN_POINT('Ctrl Pts',(-1.8380895347617,1.,-0.412633125322945));
#34252=CARTESIAN_POINT('Ctrl Pts',(-1.83100408895047,1.,-0.410641256301276));
#34253=CARTESIAN_POINT('Ctrl Pts',(-1.82247022677562,1.,-0.408428948106227));
#34254=CARTESIAN_POINT('Ctrl Pts',(-1.81223801812013,1.,-0.405933518407175));
#34255=CARTESIAN_POINT('Ctrl Pts',(-1.80012077173238,1.,-0.403107976163396));
#34256=CARTESIAN_POINT('Ctrl Pts',(-1.78598826343754,1.,-0.399919403774155));
#34257=CARTESIAN_POINT('Ctrl Pts',(-1.76975560043442,1.,-0.396346196110688));
#34258=CARTESIAN_POINT('Ctrl Pts',(-1.75137405310193,1.,-0.392375812285395));
#34259=CARTESIAN_POINT('Ctrl Pts',(-1.73493170972829,1.,-0.388877023502615));
#34260=CARTESIAN_POINT('Ctrl Pts',(-1.72162022244582,1.,-0.386070790323281));
#34261=CARTESIAN_POINT('Ctrl Pts',(-1.71231062891398,1.,-0.384119047314215));
#34262=CARTESIAN_POINT('Ctrl Pts',(-1.7075470150345,1.,-0.383122945602004));
#34263=CARTESIAN_POINT('',(-2.11275013067528,0.,-0.61342227326009));
#34264=CARTESIAN_POINT('Origin',(-2.0698113262342,0.,-0.745574324794401));
#34265=CARTESIAN_POINT('',(-2.0698113262342,1.,-0.745574324794401));
#34266=CARTESIAN_POINT('',(-2.11275013067528,1.,-0.61342227326009));
#34267=CARTESIAN_POINT('',(-2.0698113262342,0.,-0.745574324794401));
#34268=CARTESIAN_POINT('Ctrl Pts',(-1.60662857109684,-1.,-0.693717979106306));
#34269=CARTESIAN_POINT('Ctrl Pts',(-1.60662857109684,1.,-0.693717979106306));
#34270=CARTESIAN_POINT('Ctrl Pts',(-1.61106790958151,-1.,-0.695712097881194));
#34271=CARTESIAN_POINT('Ctrl Pts',(-1.61106790958151,1.,-0.695712097881194));
#34272=CARTESIAN_POINT('Ctrl Pts',(-1.61974673472612,-1.,-0.699605146405088));
#34273=CARTESIAN_POINT('Ctrl Pts',(-1.61974673472612,1.,-0.699605146405088));
#34274=CARTESIAN_POINT('Ctrl Pts',(-1.63216541664676,-1.,-0.705159151988319));
#34275=CARTESIAN_POINT('Ctrl Pts',(-1.63216541664676,1.,-0.705159151988319));
#34276=CARTESIAN_POINT('Ctrl Pts',(-1.64752408832016,-1.,-0.711993139355394));
#34277=CARTESIAN_POINT('Ctrl Pts',(-1.64752408832016,1.,-0.711993139355394));
#34278=CARTESIAN_POINT('Ctrl Pts',(-1.6647288055568,-1.,-0.719585433804282));
#34279=CARTESIAN_POINT('Ctrl Pts',(-1.6647288055568,1.,-0.719585433804282));
#34280=CARTESIAN_POINT('Ctrl Pts',(-1.67996158455503,-1.,-0.726235967997433));
#34281=CARTESIAN_POINT('Ctrl Pts',(-1.67996158455503,1.,-0.726235967997433));
#34282=CARTESIAN_POINT('Ctrl Pts',(-1.69326921975743,-1.,-0.731963238697195));
#34283=CARTESIAN_POINT('Ctrl Pts',(-1.69326921975743,1.,-0.731963238697195));
#34284=CARTESIAN_POINT('Ctrl Pts',(-1.70473309006121,-1.,-0.736799665724771));
#34285=CARTESIAN_POINT('Ctrl Pts',(-1.70473309006121,1.,-0.736799665724771));
#34286=CARTESIAN_POINT('Ctrl Pts',(-1.71447789751927,-1.,-0.740795162032087));
#34287=CARTESIAN_POINT('Ctrl Pts',(-1.71447789751927,1.,-0.740795162032087));
#34288=CARTESIAN_POINT('Ctrl Pts',(-1.7226822991693,-1.,-0.744021445433764));
#34289=CARTESIAN_POINT('Ctrl Pts',(-1.7226822991693,1.,-0.744021445433764));
#34290=CARTESIAN_POINT('Ctrl Pts',(-1.72958533647399,-1.,-0.746574710096436));
#34291=CARTESIAN_POINT('Ctrl Pts',(-1.72958533647399,1.,-0.746574710096436));
#34292=CARTESIAN_POINT('Ctrl Pts',(-1.73550351679848,-1.,-0.748582462954854));
#34293=CARTESIAN_POINT('Ctrl Pts',(-1.73550351679848,1.,-0.748582462954854));
#34294=CARTESIAN_POINT('Ctrl Pts',(-1.74080458266705,-1.,-0.75019343597954));
#34295=CARTESIAN_POINT('Ctrl Pts',(-1.74080458266705,1.,-0.75019343597954));
#34296=CARTESIAN_POINT('Ctrl Pts',(-1.74585086852298,-1.,-0.751555614163629));
#34297=CARTESIAN_POINT('Ctrl Pts',(-1.74585086852298,1.,-0.751555614163629));
#34298=CARTESIAN_POINT('Ctrl Pts',(-1.75095139468809,-1.,-0.752797683531377));
#34299=CARTESIAN_POINT('Ctrl Pts',(-1.75095139468809,1.,-0.752797683531377));
#34300=CARTESIAN_POINT('Ctrl Pts',(-1.75631083600175,-1.,-0.75400925402848));
#34301=CARTESIAN_POINT('Ctrl Pts',(-1.75631083600175,1.,-0.75400925402848));
#34302=CARTESIAN_POINT('Ctrl Pts',(-1.7619781724032,-1.,-0.755220979975262));
#34303=CARTESIAN_POINT('Ctrl Pts',(-1.7619781724032,1.,-0.755220979975262));
#34304=CARTESIAN_POINT('Ctrl Pts',(-1.76789396003141,-1.,-0.756421896028403));
#34305=CARTESIAN_POINT('Ctrl Pts',(-1.76789396003141,1.,-0.756421896028403));
#34306=CARTESIAN_POINT('Ctrl Pts',(-1.77394167108342,-1.,-0.757578264077238));
#34307=CARTESIAN_POINT('Ctrl Pts',(-1.77394167108342,1.,-0.757578264077238));
#34308=CARTESIAN_POINT('Ctrl Pts',(-1.77999411220912,-1.,-0.75865062667738));
#34309=CARTESIAN_POINT('Ctrl Pts',(-1.77999411220912,1.,-0.75865062667738));
#34310=CARTESIAN_POINT('Ctrl Pts',(-1.78596964884526,-1.,-0.759614401109868));
#34311=CARTESIAN_POINT('Ctrl Pts',(-1.78596964884526,1.,-0.759614401109868));
#34312=CARTESIAN_POINT('Ctrl Pts',(-1.79185815610802,-1.,-0.760469555880425));
#34313=CARTESIAN_POINT('Ctrl Pts',(-1.79185815610802,1.,-0.760469555880425));
#34314=CARTESIAN_POINT('Ctrl Pts',(-1.79768986997735,-1.,-0.761229695230359));
#34315=CARTESIAN_POINT('Ctrl Pts',(-1.79768986997735,1.,-0.761229695230359));
#34316=CARTESIAN_POINT('Ctrl Pts',(-1.80351583877334,-1.,-0.761915336443515));
#34317=CARTESIAN_POINT('Ctrl Pts',(-1.80351583877334,1.,-0.761915336443515));
#34318=CARTESIAN_POINT('Ctrl Pts',(-1.80938551463989,-1.,-0.762546129464036));
#34319=CARTESIAN_POINT('Ctrl Pts',(-1.80938551463989,1.,-0.762546129464036));
#34320=CARTESIAN_POINT('Ctrl Pts',(-1.81532118405566,-1.,-0.763132003836783));
#34321=CARTESIAN_POINT('Ctrl Pts',(-1.81532118405566,1.,-0.763132003836783));
#34322=CARTESIAN_POINT('Ctrl Pts',(-1.82131873145297,-1.,-0.763673465462854));
#34323=CARTESIAN_POINT('Ctrl Pts',(-1.82131873145297,1.,-0.763673465462854));
#34324=CARTESIAN_POINT('Ctrl Pts',(-1.8273599120008,-1.,-0.764165902606055));
#34325=CARTESIAN_POINT('Ctrl Pts',(-1.8273599120008,1.,-0.764165902606055));
#34326=CARTESIAN_POINT('Ctrl Pts',(-1.8334207722714,-1.,-0.764602549687845));
#34327=CARTESIAN_POINT('Ctrl Pts',(-1.8334207722714,1.,-0.764602549687845));
#34328=CARTESIAN_POINT('Ctrl Pts',(-1.83948181064823,-1.,-0.764978057881687));
#34329=CARTESIAN_POINT('Ctrl Pts',(-1.83948181064823,1.,-0.764978057881687));
#34330=CARTESIAN_POINT('Ctrl Pts',(-1.8455369887591,-1.,-0.765291664861971));
#34331=CARTESIAN_POINT('Ctrl Pts',(-1.8455369887591,1.,-0.765291664861971));
#34332=CARTESIAN_POINT('Ctrl Pts',(-1.85158945130054,-1.,-0.765545710619023));
#34333=CARTESIAN_POINT('Ctrl Pts',(-1.85158945130054,1.,-0.765545710619023));
#34334=CARTESIAN_POINT('Ctrl Pts',(-1.85764741390391,-1.,-0.765744212909305));
#34335=CARTESIAN_POINT('Ctrl Pts',(-1.85764741390391,1.,-0.765744212909305));
#34336=CARTESIAN_POINT('Ctrl Pts',(-1.86372027063314,-1.,-0.765891519092557));
#34337=CARTESIAN_POINT('Ctrl Pts',(-1.86372027063314,1.,-0.765891519092557));
#34338=CARTESIAN_POINT('Ctrl Pts',(-1.86981398314345,-1.,-0.765990708546111));
#34339=CARTESIAN_POINT('Ctrl Pts',(-1.86981398314345,1.,-0.765990708546111));
#34340=CARTESIAN_POINT('Ctrl Pts',(-1.87592888967886,-1.,-0.766042837036759));
#34341=CARTESIAN_POINT('Ctrl Pts',(-1.87592888967886,1.,-0.766042837036759));
#34342=CARTESIAN_POINT('Ctrl Pts',(-1.88206215302561,-1.,-0.766047794851868));
#34343=CARTESIAN_POINT('Ctrl Pts',(-1.88206215302561,1.,-0.766047794851868));
#34344=CARTESIAN_POINT('Ctrl Pts',(-1.88820926433409,-1.,-0.76600483706209));
#34345=CARTESIAN_POINT('Ctrl Pts',(-1.88820926433409,1.,-0.76600483706209));
#34346=CARTESIAN_POINT('Ctrl Pts',(-1.89436577771389,-1.,-0.765913193856979));
#34347=CARTESIAN_POINT('Ctrl Pts',(-1.89436577771389,1.,-0.765913193856979));
#34348=CARTESIAN_POINT('Ctrl Pts',(-1.90052930393599,-1.,-0.765772772593395));
#34349=CARTESIAN_POINT('Ctrl Pts',(-1.90052930393599,1.,-0.765772772593395));
#34350=CARTESIAN_POINT('Ctrl Pts',(-1.90669961402362,-1.,-0.765584196937936));
#34351=CARTESIAN_POINT('Ctrl Pts',(-1.90669961402362,1.,-0.765584196937936));
#34352=CARTESIAN_POINT('Ctrl Pts',(-1.91287765805174,-1.,-0.765348465884739));
#34353=CARTESIAN_POINT('Ctrl Pts',(-1.91287765805174,1.,-0.765348465884739));
#34354=CARTESIAN_POINT('Ctrl Pts',(-1.91906491634197,-1.,-0.765066729667095));
#34355=CARTESIAN_POINT('Ctrl Pts',(-1.91906491634197,1.,-0.765066729667095));
#34356=CARTESIAN_POINT('Ctrl Pts',(-1.92526263537041,-1.,-0.764740025488189));
#34357=CARTESIAN_POINT('Ctrl Pts',(-1.92526263537041,1.,-0.764740025488189));
#34358=CARTESIAN_POINT('Ctrl Pts',(-1.93147105496367,-1.,-0.764369010673889));
#34359=CARTESIAN_POINT('Ctrl Pts',(-1.93147105496367,1.,-0.764369010673889));
#34360=CARTESIAN_POINT('Ctrl Pts',(-1.93768964875867,-1.,-0.763954049121393));
#34361=CARTESIAN_POINT('Ctrl Pts',(-1.93768964875867,1.,-0.763954049121393));
#34362=CARTESIAN_POINT('Ctrl Pts',(-1.94391746617626,-1.,-0.76349533353858));
#34363=CARTESIAN_POINT('Ctrl Pts',(-1.94391746617626,1.,-0.76349533353858));
#34364=CARTESIAN_POINT('Ctrl Pts',(-1.95015342590025,-1.,-0.762992990878774));
#34365=CARTESIAN_POINT('Ctrl Pts',(-1.95015342590025,1.,-0.762992990878774));
#34366=CARTESIAN_POINT('Ctrl Pts',(-1.95639665309893,-1.,-0.762447203806263));
#34367=CARTESIAN_POINT('Ctrl Pts',(-1.95639665309893,1.,-0.762447203806263));
#34368=CARTESIAN_POINT('Ctrl Pts',(-1.96264672744229,-1.,-0.761858300014575));
#34369=CARTESIAN_POINT('Ctrl Pts',(-1.96264672744229,1.,-0.761858300014575));
#34370=CARTESIAN_POINT('Ctrl Pts',(-1.96890351582545,-1.,-0.761226690483986));
#34371=CARTESIAN_POINT('Ctrl Pts',(-1.96890351582545,1.,-0.761226690483986));
#34372=CARTESIAN_POINT('Ctrl Pts',(-1.97516705321521,-1.,-0.760552825409855));
#34373=CARTESIAN_POINT('Ctrl Pts',(-1.97516705321521,1.,-0.760552825409855));
#34374=CARTESIAN_POINT('Ctrl Pts',(-1.98143741418156,-1.,-0.759837147452135));
#34375=CARTESIAN_POINT('Ctrl Pts',(-1.98143741418156,1.,-0.759837147452135));
#34376=CARTESIAN_POINT('Ctrl Pts',(-1.98771456680806,-1.,-0.759080037802242));
#34377=CARTESIAN_POINT('Ctrl Pts',(-1.98771456680806,1.,-0.759080037802242));
#34378=CARTESIAN_POINT('Ctrl Pts',(-1.9939983109871,-1.,-0.758281796766377));
#34379=CARTESIAN_POINT('Ctrl Pts',(-1.9939983109871,1.,-0.758281796766377));
#34380=CARTESIAN_POINT('Ctrl Pts',(-2.00028834739072,-1.,-0.757442676862341));
#34381=CARTESIAN_POINT('Ctrl Pts',(-2.00028834739072,1.,-0.757442676862341));
#34382=CARTESIAN_POINT('Ctrl Pts',(-2.00658431587682,-1.,-0.756562904646496));
#34383=CARTESIAN_POINT('Ctrl Pts',(-2.00658431587682,1.,-0.756562904646496));
#34384=CARTESIAN_POINT('Ctrl Pts',(-2.01288584328149,-1.,-0.7556427049581));
#34385=CARTESIAN_POINT('Ctrl Pts',(-2.01288584328149,1.,-0.7556427049581));
#34386=CARTESIAN_POINT('Ctrl Pts',(-2.01919259406003,-1.,-0.75468233072352));
#34387=CARTESIAN_POINT('Ctrl Pts',(-2.01919259406003,1.,-0.75468233072352));
#34388=CARTESIAN_POINT('Ctrl Pts',(-2.02550428623587,-1.,-0.753682061113765));
#34389=CARTESIAN_POINT('Ctrl Pts',(-2.02550428623587,1.,-0.753682061113765));
#34390=CARTESIAN_POINT('Ctrl Pts',(-2.03182068456467,-1.,-0.752642180488104));
#34391=CARTESIAN_POINT('Ctrl Pts',(-2.03182068456467,1.,-0.752642180488104));
#34392=CARTESIAN_POINT('Ctrl Pts',(-2.03814160092173,-1.,-0.751562963361383));
#34393=CARTESIAN_POINT('Ctrl Pts',(-2.03814160092173,1.,-0.751562963361383));
#34394=CARTESIAN_POINT('Ctrl Pts',(-2.04446689147754,-1.,-0.750444657874758));
#34395=CARTESIAN_POINT('Ctrl Pts',(-2.04446689147754,1.,-0.750444657874758));
#34396=CARTESIAN_POINT('Ctrl Pts',(-2.05079645591606,-1.,-0.749287468663053));
#34397=CARTESIAN_POINT('Ctrl Pts',(-2.05079645591606,1.,-0.749287468663053));
#34398=CARTESIAN_POINT('Ctrl Pts',(-2.05713023030263,-1.,-0.748091554181101));
#34399=CARTESIAN_POINT('Ctrl Pts',(-2.05713023030263,1.,-0.748091554181101));
#34400=CARTESIAN_POINT('Ctrl Pts',(-2.06220058927162,-1.,-0.747103932785504));
#34401=CARTESIAN_POINT('Ctrl Pts',(-2.06220058927162,1.,-0.747103932785504));
#34402=CARTESIAN_POINT('Ctrl Pts',(-2.06600523016401,-1.,-0.746345871542695));
#34403=CARTESIAN_POINT('Ctrl Pts',(-2.06600523016401,1.,-0.746345871542695));
#34404=CARTESIAN_POINT('Ctrl Pts',(-2.06854248895575,-1.,-0.74583279137781));
#34405=CARTESIAN_POINT('Ctrl Pts',(-2.06854248895575,1.,-0.74583279137781));
#34406=CARTESIAN_POINT('Ctrl Pts',(-2.0698113262342,-1.,-0.745574324794401));
#34407=CARTESIAN_POINT('Ctrl Pts',(-2.0698113262342,1.,-0.745574324794401));
#34408=CARTESIAN_POINT('',(-1.60662857109684,1.,-0.693717979106306));
#34409=CARTESIAN_POINT('Ctrl Pts',(-1.60662857109684,1.,-0.693717979106306));
#34410=CARTESIAN_POINT('Ctrl Pts',(-1.61106790958151,1.,-0.695712097881194));
#34411=CARTESIAN_POINT('Ctrl Pts',(-1.61974673472612,1.,-0.699605146405088));
#34412=CARTESIAN_POINT('Ctrl Pts',(-1.63216541664676,1.,-0.705159151988319));
#34413=CARTESIAN_POINT('Ctrl Pts',(-1.64752408832016,1.,-0.711993139355394));
#34414=CARTESIAN_POINT('Ctrl Pts',(-1.6647288055568,1.,-0.719585433804282));
#34415=CARTESIAN_POINT('Ctrl Pts',(-1.67996158455503,1.,-0.726235967997433));
#34416=CARTESIAN_POINT('Ctrl Pts',(-1.69326921975743,1.,-0.731963238697195));
#34417=CARTESIAN_POINT('Ctrl Pts',(-1.70473309006121,1.,-0.736799665724771));
#34418=CARTESIAN_POINT('Ctrl Pts',(-1.71447789751927,1.,-0.740795162032087));
#34419=CARTESIAN_POINT('Ctrl Pts',(-1.7226822991693,1.,-0.744021445433764));
#34420=CARTESIAN_POINT('Ctrl Pts',(-1.72958533647399,1.,-0.746574710096436));
#34421=CARTESIAN_POINT('Ctrl Pts',(-1.73550351679848,1.,-0.748582462954854));
#34422=CARTESIAN_POINT('Ctrl Pts',(-1.74080458266705,1.,-0.75019343597954));
#34423=CARTESIAN_POINT('Ctrl Pts',(-1.74585086852298,1.,-0.751555614163629));
#34424=CARTESIAN_POINT('Ctrl Pts',(-1.75095139468809,1.,-0.752797683531377));
#34425=CARTESIAN_POINT('Ctrl Pts',(-1.75631083600175,1.,-0.75400925402848));
#34426=CARTESIAN_POINT('Ctrl Pts',(-1.7619781724032,1.,-0.755220979975262));
#34427=CARTESIAN_POINT('Ctrl Pts',(-1.76789396003141,1.,-0.756421896028403));
#34428=CARTESIAN_POINT('Ctrl Pts',(-1.77394167108342,1.,-0.757578264077238));
#34429=CARTESIAN_POINT('Ctrl Pts',(-1.77999411220912,1.,-0.75865062667738));
#34430=CARTESIAN_POINT('Ctrl Pts',(-1.78596964884526,1.,-0.759614401109868));
#34431=CARTESIAN_POINT('Ctrl Pts',(-1.79185815610802,1.,-0.760469555880425));
#34432=CARTESIAN_POINT('Ctrl Pts',(-1.79768986997735,1.,-0.761229695230359));
#34433=CARTESIAN_POINT('Ctrl Pts',(-1.80351583877334,1.,-0.761915336443515));
#34434=CARTESIAN_POINT('Ctrl Pts',(-1.80938551463989,1.,-0.762546129464036));
#34435=CARTESIAN_POINT('Ctrl Pts',(-1.81532118405566,1.,-0.763132003836783));
#34436=CARTESIAN_POINT('Ctrl Pts',(-1.82131873145297,1.,-0.763673465462854));
#34437=CARTESIAN_POINT('Ctrl Pts',(-1.8273599120008,1.,-0.764165902606055));
#34438=CARTESIAN_POINT('Ctrl Pts',(-1.8334207722714,1.,-0.764602549687845));
#34439=CARTESIAN_POINT('Ctrl Pts',(-1.83948181064823,1.,-0.764978057881687));
#34440=CARTESIAN_POINT('Ctrl Pts',(-1.8455369887591,1.,-0.765291664861971));
#34441=CARTESIAN_POINT('Ctrl Pts',(-1.85158945130054,1.,-0.765545710619023));
#34442=CARTESIAN_POINT('Ctrl Pts',(-1.85764741390391,1.,-0.765744212909305));
#34443=CARTESIAN_POINT('Ctrl Pts',(-1.86372027063314,1.,-0.765891519092557));
#34444=CARTESIAN_POINT('Ctrl Pts',(-1.86981398314345,1.,-0.765990708546111));
#34445=CARTESIAN_POINT('Ctrl Pts',(-1.87592888967886,1.,-0.766042837036759));
#34446=CARTESIAN_POINT('Ctrl Pts',(-1.88206215302561,1.,-0.766047794851868));
#34447=CARTESIAN_POINT('Ctrl Pts',(-1.88820926433409,1.,-0.76600483706209));
#34448=CARTESIAN_POINT('Ctrl Pts',(-1.89436577771389,1.,-0.765913193856979));
#34449=CARTESIAN_POINT('Ctrl Pts',(-1.90052930393599,1.,-0.765772772593395));
#34450=CARTESIAN_POINT('Ctrl Pts',(-1.90669961402362,1.,-0.765584196937936));
#34451=CARTESIAN_POINT('Ctrl Pts',(-1.91287765805174,1.,-0.765348465884739));
#34452=CARTESIAN_POINT('Ctrl Pts',(-1.91906491634197,1.,-0.765066729667095));
#34453=CARTESIAN_POINT('Ctrl Pts',(-1.92526263537041,1.,-0.764740025488189));
#34454=CARTESIAN_POINT('Ctrl Pts',(-1.93147105496367,1.,-0.764369010673889));
#34455=CARTESIAN_POINT('Ctrl Pts',(-1.93768964875867,1.,-0.763954049121393));
#34456=CARTESIAN_POINT('Ctrl Pts',(-1.94391746617626,1.,-0.76349533353858));
#34457=CARTESIAN_POINT('Ctrl Pts',(-1.95015342590025,1.,-0.762992990878774));
#34458=CARTESIAN_POINT('Ctrl Pts',(-1.95639665309893,1.,-0.762447203806263));
#34459=CARTESIAN_POINT('Ctrl Pts',(-1.96264672744229,1.,-0.761858300014575));
#34460=CARTESIAN_POINT('Ctrl Pts',(-1.96890351582545,1.,-0.761226690483986));
#34461=CARTESIAN_POINT('Ctrl Pts',(-1.97516705321521,1.,-0.760552825409855));
#34462=CARTESIAN_POINT('Ctrl Pts',(-1.98143741418156,1.,-0.759837147452135));
#34463=CARTESIAN_POINT('Ctrl Pts',(-1.98771456680806,1.,-0.759080037802242));
#34464=CARTESIAN_POINT('Ctrl Pts',(-1.9939983109871,1.,-0.758281796766377));
#34465=CARTESIAN_POINT('Ctrl Pts',(-2.00028834739072,1.,-0.757442676862341));
#34466=CARTESIAN_POINT('Ctrl Pts',(-2.00658431587682,1.,-0.756562904646496));
#34467=CARTESIAN_POINT('Ctrl Pts',(-2.01288584328149,1.,-0.7556427049581));
#34468=CARTESIAN_POINT('Ctrl Pts',(-2.01919259406003,1.,-0.75468233072352));
#34469=CARTESIAN_POINT('Ctrl Pts',(-2.02550428623587,1.,-0.753682061113765));
#34470=CARTESIAN_POINT('Ctrl Pts',(-2.03182068456467,1.,-0.752642180488104));
#34471=CARTESIAN_POINT('Ctrl Pts',(-2.03814160092173,1.,-0.751562963361383));
#34472=CARTESIAN_POINT('Ctrl Pts',(-2.04446689147754,1.,-0.750444657874758));
#34473=CARTESIAN_POINT('Ctrl Pts',(-2.05079645591606,1.,-0.749287468663053));
#34474=CARTESIAN_POINT('Ctrl Pts',(-2.05713023030263,1.,-0.748091554181101));
#34475=CARTESIAN_POINT('Ctrl Pts',(-2.06220058927162,1.,-0.747103932785504));
#34476=CARTESIAN_POINT('Ctrl Pts',(-2.06600523016401,1.,-0.746345871542695));
#34477=CARTESIAN_POINT('Ctrl Pts',(-2.06854248895575,1.,-0.74583279137781));
#34478=CARTESIAN_POINT('Ctrl Pts',(-2.0698113262342,1.,-0.745574324794401));
#34479=CARTESIAN_POINT('',(-1.60662857109684,0.,-0.693717979106306));
#34480=CARTESIAN_POINT('Origin',(0.,0.,0.));
#34481=CARTESIAN_POINT('',(-1.5055822144029,1.,-0.892032620296855));
#34482=CARTESIAN_POINT('Origin',(0.,1.,0.));
#34483=CARTESIAN_POINT('',(-1.5055822144029,0.,-0.892032620296855));
#34484=CARTESIAN_POINT('Ctrl Pts',(-1.81978687191668,-1.,-1.23627494547115));
#34485=CARTESIAN_POINT('Ctrl Pts',(-1.81978687191668,1.,-1.23627494547115));
#34486=CARTESIAN_POINT('Ctrl Pts',(-1.81925017193666,-1.,-1.23509651170476));
#34487=CARTESIAN_POINT('Ctrl Pts',(-1.81925017193666,1.,-1.23509651170476));
#34488=CARTESIAN_POINT('Ctrl Pts',(-1.81817389921279,-1.,-1.2327422452705));
#34489=CARTESIAN_POINT('Ctrl Pts',(-1.81817389921279,1.,-1.2327422452705));
#34490=CARTESIAN_POINT('Ctrl Pts',(-1.8165508718364,-1.,-1.2292186489137));
#34491=CARTESIAN_POINT('Ctrl Pts',(-1.8165508718364,1.,-1.2292186489137));
#34492=CARTESIAN_POINT('Ctrl Pts',(-1.81436959210434,-1.,-1.2245361330495));
#34493=CARTESIAN_POINT('Ctrl Pts',(-1.81436959210434,1.,-1.2245361330495));
#34494=CARTESIAN_POINT('Ctrl Pts',(-1.81161420806656,-1.,-1.21870906103557));
#34495=CARTESIAN_POINT('Ctrl Pts',(-1.81161420806656,1.,-1.21870906103557));
#34496=CARTESIAN_POINT('Ctrl Pts',(-1.80882996917129,-1.,-1.21290815708314));
#34497=CARTESIAN_POINT('Ctrl Pts',(-1.80882996917129,1.,-1.21290815708314));
#34498=CARTESIAN_POINT('Ctrl Pts',(-1.80601678480707,-1.,-1.20713356605475));
#34499=CARTESIAN_POINT('Ctrl Pts',(-1.80601678480707,1.,-1.20713356605475));
#34500=CARTESIAN_POINT('Ctrl Pts',(-1.80317454838603,-1.,-1.20138548938974));
#34501=CARTESIAN_POINT('Ctrl Pts',(-1.80317454838603,1.,-1.20138548938974));
#34502=CARTESIAN_POINT('Ctrl Pts',(-1.80030314369879,-1.,-1.19566418930242));
#34503=CARTESIAN_POINT('Ctrl Pts',(-1.80030314369879,1.,-1.19566418930242));
#34504=CARTESIAN_POINT('Ctrl Pts',(-1.79740245923478,-1.,-1.18996997934445));
#34505=CARTESIAN_POINT('Ctrl Pts',(-1.79740245923478,1.,-1.18996997934445));
#34506=CARTESIAN_POINT('Ctrl Pts',(-1.79447240321515,-1.,-1.18430321697432));
#34507=CARTESIAN_POINT('Ctrl Pts',(-1.79447240321515,1.,-1.18430321697432));
#34508=CARTESIAN_POINT('Ctrl Pts',(-1.79151291552689,-1.,-1.17866429440809));
#34509=CARTESIAN_POINT('Ctrl Pts',(-1.79151291552689,1.,-1.17866429440809));
#34510=CARTESIAN_POINT('Ctrl Pts',(-1.78852398877616,-1.,-1.17305363177328));
#34511=CARTESIAN_POINT('Ctrl Pts',(-1.78852398877616,1.,-1.17305363177328));
#34512=CARTESIAN_POINT('Ctrl Pts',(-1.78550566040443,-1.,-1.16747166312303));
#34513=CARTESIAN_POINT('Ctrl Pts',(-1.78550566040443,1.,-1.16747166312303));
#34514=CARTESIAN_POINT('Ctrl Pts',(-1.78245795881009,-1.,-1.16191881298499));
#34515=CARTESIAN_POINT('Ctrl Pts',(-1.78245795881009,1.,-1.16191881298499));
#34516=CARTESIAN_POINT('Ctrl Pts',(-1.77938085564275,-1.,-1.15639547194698));
#34517=CARTESIAN_POINT('Ctrl Pts',(-1.77938085564275,1.,-1.15639547194698));
#34518=CARTESIAN_POINT('Ctrl Pts',(-1.7762742255701,-1.,-1.15090197841515));
#34519=CARTESIAN_POINT('Ctrl Pts',(-1.7762742255701,1.,-1.15090197841515));
#34520=CARTESIAN_POINT('Ctrl Pts',(-1.77313777896194,-1.,-1.1454385822692));
#34521=CARTESIAN_POINT('Ctrl Pts',(-1.77313777896194,1.,-1.1454385822692));
#34522=CARTESIAN_POINT('Ctrl Pts',(-1.76997111386769,-1.,-1.14000548336975));
#34523=CARTESIAN_POINT('Ctrl Pts',(-1.76997111386769,1.,-1.14000548336975));
#34524=CARTESIAN_POINT('Ctrl Pts',(-1.76677384551862,-1.,-1.1346029180462));
#34525=CARTESIAN_POINT('Ctrl Pts',(-1.76677384551862,1.,-1.1346029180462));
#34526=CARTESIAN_POINT('Ctrl Pts',(-1.7635457196617,-1.,-1.12923123555075));
#34527=CARTESIAN_POINT('Ctrl Pts',(-1.7635457196617,1.,-1.12923123555075));
#34528=CARTESIAN_POINT('Ctrl Pts',(-1.76028671825096,-1.,-1.12389096855086));
#34529=CARTESIAN_POINT('Ctrl Pts',(-1.76028671825096,1.,-1.12389096855086));
#34530=CARTESIAN_POINT('Ctrl Pts',(-1.75699720772105,-1.,-1.11858293216763));
#34531=CARTESIAN_POINT('Ctrl Pts',(-1.75699720772105,1.,-1.11858293216763));
#34532=CARTESIAN_POINT('Ctrl Pts',(-1.7536777209463,-1.,-1.11330807582551));
#34533=CARTESIAN_POINT('Ctrl Pts',(-1.7536777209463,1.,-1.11330807582551));
#34534=CARTESIAN_POINT('Ctrl Pts',(-1.7503286607592,-1.,-1.10806728183007));
#34535=CARTESIAN_POINT('Ctrl Pts',(-1.7503286607592,1.,-1.10806728183007));
#34536=CARTESIAN_POINT('Ctrl Pts',(-1.74695004214923,-1.,-1.10286118991143));
#34537=CARTESIAN_POINT('Ctrl Pts',(-1.74695004214923,1.,-1.10286118991143));
#34538=CARTESIAN_POINT('Ctrl Pts',(-1.74354119236208,-1.,-1.09768999241225));
#34539=CARTESIAN_POINT('Ctrl Pts',(-1.74354119236208,1.,-1.09768999241225));
#34540=CARTESIAN_POINT('Ctrl Pts',(-1.74010053962247,-1.,-1.09255329056493));
#34541=CARTESIAN_POINT('Ctrl Pts',(-1.74010053962247,1.,-1.09255329056493));
#34542=CARTESIAN_POINT('Ctrl Pts',(-1.73662628326091,-1.,-1.08745056285427));
#34543=CARTESIAN_POINT('Ctrl Pts',(-1.73662628326091,1.,-1.08745056285427));
#34544=CARTESIAN_POINT('Ctrl Pts',(-1.73311705663407,-1.,-1.08238162784749));
#34545=CARTESIAN_POINT('Ctrl Pts',(-1.73311705663407,1.,-1.08238162784749));
#34546=CARTESIAN_POINT('Ctrl Pts',(-1.72957248977424,-1.,-1.0773470373727));
#34547=CARTESIAN_POINT('Ctrl Pts',(-1.72957248977424,1.,-1.0773470373727));
#34548=CARTESIAN_POINT('Ctrl Pts',(-1.72599406198488,-1.,-1.07234866990252));
#34549=CARTESIAN_POINT('Ctrl Pts',(-1.72599406198488,1.,-1.07234866990252));
#34550=CARTESIAN_POINT('Ctrl Pts',(-1.72238500928453,-1.,-1.06738966975462));
#34551=CARTESIAN_POINT('Ctrl Pts',(-1.72238500928453,1.,-1.06738966975462));
#34552=CARTESIAN_POINT('Ctrl Pts',(-1.71874858456904,-1.,-1.06247324680647));
#34553=CARTESIAN_POINT('Ctrl Pts',(-1.71874858456904,1.,-1.06247324680647));
#34554=CARTESIAN_POINT('Ctrl Pts',(-1.7150865442702,-1.,-1.05760163192479));
#34555=CARTESIAN_POINT('Ctrl Pts',(-1.7150865442702,1.,-1.05760163192479));
#34556=CARTESIAN_POINT('Ctrl Pts',(-1.71139783543989,-1.,-1.05277517202855));
#34557=CARTESIAN_POINT('Ctrl Pts',(-1.71139783543989,1.,-1.05277517202855));
#34558=CARTESIAN_POINT('Ctrl Pts',(-1.70767646263649,-1.,-1.04799085404995));
#34559=CARTESIAN_POINT('Ctrl Pts',(-1.70767646263649,1.,-1.04799085404995));
#34560=CARTESIAN_POINT('Ctrl Pts',(-1.70391338707982,-1.,-1.04324363334554));
#34561=CARTESIAN_POINT('Ctrl Pts',(-1.70391338707982,1.,-1.04324363334554));
#34562=CARTESIAN_POINT('Ctrl Pts',(-1.70010052930962,-1.,-1.03852922490789));
#34563=CARTESIAN_POINT('Ctrl Pts',(-1.70010052930962,1.,-1.03852922490789));
#34564=CARTESIAN_POINT('Ctrl Pts',(-1.69623414782771,-1.,-1.03384646003588));
#34565=CARTESIAN_POINT('Ctrl Pts',(-1.69623414782771,1.,-1.03384646003588));
#34566=CARTESIAN_POINT('Ctrl Pts',(-1.69231840863458,-1.,-1.02919977579147));
#34567=CARTESIAN_POINT('Ctrl Pts',(-1.69231840863458,1.,-1.02919977579147));
#34568=CARTESIAN_POINT('Ctrl Pts',(-1.68836910178447,-1.,-1.02460180535255));
#34569=CARTESIAN_POINT('Ctrl Pts',(-1.68836910178447,1.,-1.02460180535255));
#34570=CARTESIAN_POINT('Ctrl Pts',(-1.68440578021706,-1.,-1.02006795074201));
#34571=CARTESIAN_POINT('Ctrl Pts',(-1.68440578021706,1.,-1.02006795074201));
#34572=CARTESIAN_POINT('Ctrl Pts',(-1.68044289894798,-1.,-1.01561026162773));
#34573=CARTESIAN_POINT('Ctrl Pts',(-1.68044289894798,1.,-1.01561026162773));
#34574=CARTESIAN_POINT('Ctrl Pts',(-1.67648246776464,-1.,-1.01123236493511));
#34575=CARTESIAN_POINT('Ctrl Pts',(-1.67648246776464,1.,-1.01123236493511));
#34576=CARTESIAN_POINT('Ctrl Pts',(-1.67250335383293,-1.,-1.00692206696414));
#34577=CARTESIAN_POINT('Ctrl Pts',(-1.67250335383293,1.,-1.00692206696414));
#34578=CARTESIAN_POINT('Ctrl Pts',(-1.66846059277303,-1.,-1.00265091003727));
#34579=CARTESIAN_POINT('Ctrl Pts',(-1.66846059277303,1.,-1.00265091003727));
#34580=CARTESIAN_POINT('Ctrl Pts',(-1.66430758030376,-1.,-0.998389654952758));
#34581=CARTESIAN_POINT('Ctrl Pts',(-1.66430758030376,1.,-0.998389654952758));
#34582=CARTESIAN_POINT('Ctrl Pts',(-1.66001553809947,-1.,-0.994121836661306));
#34583=CARTESIAN_POINT('Ctrl Pts',(-1.66001553809947,1.,-0.994121836661306));
#34584=CARTESIAN_POINT('Ctrl Pts',(-1.65559044289699,-1.,-0.989855627854165));
#34585=CARTESIAN_POINT('Ctrl Pts',(-1.65559044289699,1.,-0.989855627854165));
#34586=CARTESIAN_POINT('Ctrl Pts',(-1.65110016612638,-1.,-0.985642622920821));
#34587=CARTESIAN_POINT('Ctrl Pts',(-1.65110016612638,1.,-0.985642622920821));
#34588=CARTESIAN_POINT('Ctrl Pts',(-1.64665139190656,-1.,-0.981562530939489));
#34589=CARTESIAN_POINT('Ctrl Pts',(-1.64665139190656,1.,-0.981562530939489));
#34590=CARTESIAN_POINT('Ctrl Pts',(-1.64233990826687,-1.,-0.977689794119416));
#34591=CARTESIAN_POINT('Ctrl Pts',(-1.64233990826687,1.,-0.977689794119416));
#34592=CARTESIAN_POINT('Ctrl Pts',(-1.63820952658144,-1.,-0.974066058287418));
#34593=CARTESIAN_POINT('Ctrl Pts',(-1.63820952658144,1.,-0.974066058287418));
#34594=CARTESIAN_POINT('Ctrl Pts',(-1.63420665729798,-1.,-0.970669715997509));
#34595=CARTESIAN_POINT('Ctrl Pts',(-1.63420665729798,1.,-0.970669715997509));
#34596=CARTESIAN_POINT('Ctrl Pts',(-1.63013849959461,-1.,-0.967387853230345));
#34597=CARTESIAN_POINT('Ctrl Pts',(-1.63013849959461,1.,-0.967387853230345));
#34598=CARTESIAN_POINT('Ctrl Pts',(-1.62571930670187,-1.,-0.964046107040536));
#34599=CARTESIAN_POINT('Ctrl Pts',(-1.62571930670187,1.,-0.964046107040536));
#34600=CARTESIAN_POINT('Ctrl Pts',(-1.62061638140221,-1.,-0.960438326101729));
#34601=CARTESIAN_POINT('Ctrl Pts',(-1.62061638140221,1.,-0.960438326101729));
#34602=CARTESIAN_POINT('Ctrl Pts',(-1.61449324337085,-1.,-0.956354422920671));
#34603=CARTESIAN_POINT('Ctrl Pts',(-1.61449324337085,1.,-0.956354422920671));
#34604=CARTESIAN_POINT('Ctrl Pts',(-1.60706069896936,-1.,-0.951613284356035));
#34605=CARTESIAN_POINT('Ctrl Pts',(-1.60706069896936,1.,-0.951613284356035));
#34606=CARTESIAN_POINT('Ctrl Pts',(-1.59810042043673,-1.,-0.946078063315257));
#34607=CARTESIAN_POINT('Ctrl Pts',(-1.59810042043673,1.,-0.946078063315257));
#34608=CARTESIAN_POINT('Ctrl Pts',(-1.58744937487176,-1.,-0.939646377893399));
#34609=CARTESIAN_POINT('Ctrl Pts',(-1.58744937487176,1.,-0.939646377893399));
#34610=CARTESIAN_POINT('Ctrl Pts',(-1.57499388382243,-1.,-0.932246680108685));
#34611=CARTESIAN_POINT('Ctrl Pts',(-1.57499388382243,1.,-0.932246680108685));
#34612=CARTESIAN_POINT('Ctrl Pts',(-1.56065988578893,-1.,-0.923832188944341));
#34613=CARTESIAN_POINT('Ctrl Pts',(-1.56065988578893,1.,-0.923832188944341));
#34614=CARTESIAN_POINT('Ctrl Pts',(-1.54440491149498,-1.,-0.914375919026456));
#34615=CARTESIAN_POINT('Ctrl Pts',(-1.54440491149498,1.,-0.914375919026456));
#34616=CARTESIAN_POINT('Ctrl Pts',(-1.52984849887993,-1.,-0.905967409625651));
#34617=CARTESIAN_POINT('Ctrl Pts',(-1.52984849887993,1.,-0.905967409625651));
#34618=CARTESIAN_POINT('Ctrl Pts',(-1.51805569590094,-1.,-0.899185047483511));
#34619=CARTESIAN_POINT('Ctrl Pts',(-1.51805569590094,1.,-0.899185047483511));
#34620=CARTESIAN_POINT('Ctrl Pts',(-1.50980486806688,-1.,-0.894452006964543));
#34621=CARTESIAN_POINT('Ctrl Pts',(-1.50980486806688,1.,-0.894452006964543));
#34622=CARTESIAN_POINT('Ctrl Pts',(-1.5055822144029,-1.,-0.892032620296855));
#34623=CARTESIAN_POINT('Ctrl Pts',(-1.5055822144029,1.,-0.892032620296855));
#34624=CARTESIAN_POINT('',(-1.81978687191668,1.,-1.23627494547115));
#34625=CARTESIAN_POINT('Ctrl Pts',(-1.81978687191668,1.,-1.23627494547115));
#34626=CARTESIAN_POINT('Ctrl Pts',(-1.81925017193666,1.,-1.23509651170476));
#34627=CARTESIAN_POINT('Ctrl Pts',(-1.81817389921279,1.,-1.2327422452705));
#34628=CARTESIAN_POINT('Ctrl Pts',(-1.8165508718364,1.,-1.2292186489137));
#34629=CARTESIAN_POINT('Ctrl Pts',(-1.81436959210434,1.,-1.2245361330495));
#34630=CARTESIAN_POINT('Ctrl Pts',(-1.81161420806656,1.,-1.21870906103557));
#34631=CARTESIAN_POINT('Ctrl Pts',(-1.80882996917129,1.,-1.21290815708314));
#34632=CARTESIAN_POINT('Ctrl Pts',(-1.80601678480707,1.,-1.20713356605475));
#34633=CARTESIAN_POINT('Ctrl Pts',(-1.80317454838603,1.,-1.20138548938974));
#34634=CARTESIAN_POINT('Ctrl Pts',(-1.80030314369879,1.,-1.19566418930242));
#34635=CARTESIAN_POINT('Ctrl Pts',(-1.79740245923478,1.,-1.18996997934445));
#34636=CARTESIAN_POINT('Ctrl Pts',(-1.79447240321515,1.,-1.18430321697432));
#34637=CARTESIAN_POINT('Ctrl Pts',(-1.79151291552689,1.,-1.17866429440809));
#34638=CARTESIAN_POINT('Ctrl Pts',(-1.78852398877616,1.,-1.17305363177328));
#34639=CARTESIAN_POINT('Ctrl Pts',(-1.78550566040443,1.,-1.16747166312303));
#34640=CARTESIAN_POINT('Ctrl Pts',(-1.78245795881009,1.,-1.16191881298499));
#34641=CARTESIAN_POINT('Ctrl Pts',(-1.77938085564275,1.,-1.15639547194698));
#34642=CARTESIAN_POINT('Ctrl Pts',(-1.7762742255701,1.,-1.15090197841515));
#34643=CARTESIAN_POINT('Ctrl Pts',(-1.77313777896194,1.,-1.1454385822692));
#34644=CARTESIAN_POINT('Ctrl Pts',(-1.76997111386769,1.,-1.14000548336975));
#34645=CARTESIAN_POINT('Ctrl Pts',(-1.76677384551862,1.,-1.1346029180462));
#34646=CARTESIAN_POINT('Ctrl Pts',(-1.7635457196617,1.,-1.12923123555075));
#34647=CARTESIAN_POINT('Ctrl Pts',(-1.76028671825096,1.,-1.12389096855086));
#34648=CARTESIAN_POINT('Ctrl Pts',(-1.75699720772105,1.,-1.11858293216763));
#34649=CARTESIAN_POINT('Ctrl Pts',(-1.7536777209463,1.,-1.11330807582551));
#34650=CARTESIAN_POINT('Ctrl Pts',(-1.7503286607592,1.,-1.10806728183007));
#34651=CARTESIAN_POINT('Ctrl Pts',(-1.74695004214923,1.,-1.10286118991143));
#34652=CARTESIAN_POINT('Ctrl Pts',(-1.74354119236208,1.,-1.09768999241225));
#34653=CARTESIAN_POINT('Ctrl Pts',(-1.74010053962247,1.,-1.09255329056493));
#34654=CARTESIAN_POINT('Ctrl Pts',(-1.73662628326091,1.,-1.08745056285427));
#34655=CARTESIAN_POINT('Ctrl Pts',(-1.73311705663407,1.,-1.08238162784749));
#34656=CARTESIAN_POINT('Ctrl Pts',(-1.72957248977424,1.,-1.0773470373727));
#34657=CARTESIAN_POINT('Ctrl Pts',(-1.72599406198488,1.,-1.07234866990252));
#34658=CARTESIAN_POINT('Ctrl Pts',(-1.72238500928453,1.,-1.06738966975462));
#34659=CARTESIAN_POINT('Ctrl Pts',(-1.71874858456904,1.,-1.06247324680647));
#34660=CARTESIAN_POINT('Ctrl Pts',(-1.7150865442702,1.,-1.05760163192479));
#34661=CARTESIAN_POINT('Ctrl Pts',(-1.71139783543989,1.,-1.05277517202855));
#34662=CARTESIAN_POINT('Ctrl Pts',(-1.70767646263649,1.,-1.04799085404995));
#34663=CARTESIAN_POINT('Ctrl Pts',(-1.70391338707982,1.,-1.04324363334554));
#34664=CARTESIAN_POINT('Ctrl Pts',(-1.70010052930962,1.,-1.03852922490789));
#34665=CARTESIAN_POINT('Ctrl Pts',(-1.69623414782771,1.,-1.03384646003588));
#34666=CARTESIAN_POINT('Ctrl Pts',(-1.69231840863458,1.,-1.02919977579147));
#34667=CARTESIAN_POINT('Ctrl Pts',(-1.68836910178447,1.,-1.02460180535255));
#34668=CARTESIAN_POINT('Ctrl Pts',(-1.68440578021706,1.,-1.02006795074201));
#34669=CARTESIAN_POINT('Ctrl Pts',(-1.68044289894798,1.,-1.01561026162773));
#34670=CARTESIAN_POINT('Ctrl Pts',(-1.67648246776464,1.,-1.01123236493511));
#34671=CARTESIAN_POINT('Ctrl Pts',(-1.67250335383293,1.,-1.00692206696414));
#34672=CARTESIAN_POINT('Ctrl Pts',(-1.66846059277303,1.,-1.00265091003727));
#34673=CARTESIAN_POINT('Ctrl Pts',(-1.66430758030376,1.,-0.998389654952758));
#34674=CARTESIAN_POINT('Ctrl Pts',(-1.66001553809947,1.,-0.994121836661306));
#34675=CARTESIAN_POINT('Ctrl Pts',(-1.65559044289699,1.,-0.989855627854165));
#34676=CARTESIAN_POINT('Ctrl Pts',(-1.65110016612638,1.,-0.985642622920821));
#34677=CARTESIAN_POINT('Ctrl Pts',(-1.64665139190656,1.,-0.981562530939489));
#34678=CARTESIAN_POINT('Ctrl Pts',(-1.64233990826687,1.,-0.977689794119416));
#34679=CARTESIAN_POINT('Ctrl Pts',(-1.63820952658144,1.,-0.974066058287418));
#34680=CARTESIAN_POINT('Ctrl Pts',(-1.63420665729798,1.,-0.970669715997509));
#34681=CARTESIAN_POINT('Ctrl Pts',(-1.63013849959461,1.,-0.967387853230345));
#34682=CARTESIAN_POINT('Ctrl Pts',(-1.62571930670187,1.,-0.964046107040536));
#34683=CARTESIAN_POINT('Ctrl Pts',(-1.62061638140221,1.,-0.960438326101729));
#34684=CARTESIAN_POINT('Ctrl Pts',(-1.61449324337085,1.,-0.956354422920671));
#34685=CARTESIAN_POINT('Ctrl Pts',(-1.60706069896936,1.,-0.951613284356035));
#34686=CARTESIAN_POINT('Ctrl Pts',(-1.59810042043673,1.,-0.946078063315257));
#34687=CARTESIAN_POINT('Ctrl Pts',(-1.58744937487176,1.,-0.939646377893399));
#34688=CARTESIAN_POINT('Ctrl Pts',(-1.57499388382243,1.,-0.932246680108685));
#34689=CARTESIAN_POINT('Ctrl Pts',(-1.56065988578893,1.,-0.923832188944341));
#34690=CARTESIAN_POINT('Ctrl Pts',(-1.54440491149498,1.,-0.914375919026456));
#34691=CARTESIAN_POINT('Ctrl Pts',(-1.52984849887993,1.,-0.905967409625651));
#34692=CARTESIAN_POINT('Ctrl Pts',(-1.51805569590094,1.,-0.899185047483511));
#34693=CARTESIAN_POINT('Ctrl Pts',(-1.50980486806688,1.,-0.894452006964543));
#34694=CARTESIAN_POINT('Ctrl Pts',(-1.5055822144029,1.,-0.892032620296855));
#34695=CARTESIAN_POINT('',(-1.81978687191668,0.,-1.23627494547115));
#34696=CARTESIAN_POINT('Origin',(-1.73811241238545,0.,-1.34869019493419));
#34697=CARTESIAN_POINT('',(-1.73811241238545,1.,-1.34869019493419));
#34698=CARTESIAN_POINT('',(-1.81978687191668,1.,-1.23627494547115));
#34699=CARTESIAN_POINT('',(-1.73811241238545,0.,-1.34869019493419));
#34700=CARTESIAN_POINT('Ctrl Pts',(-1.31362392696032,-1.,-1.15624053661742));
#34701=CARTESIAN_POINT('Ctrl Pts',(-1.31362392696032,1.,-1.15624053661742));
#34702=CARTESIAN_POINT('Ctrl Pts',(-1.31722977216397,-1.,-1.15950888730809));
#34703=CARTESIAN_POINT('Ctrl Pts',(-1.31722977216397,1.,-1.15950888730809));
#34704=CARTESIAN_POINT('Ctrl Pts',(-1.32428080721772,-1.,-1.16589330093588));
#34705=CARTESIAN_POINT('Ctrl Pts',(-1.32428080721772,1.,-1.16589330093588));
#34706=CARTESIAN_POINT('Ctrl Pts',(-1.33437539347008,-1.,-1.17501305789857));
#34707=CARTESIAN_POINT('Ctrl Pts',(-1.33437539347008,1.,-1.17501305789857));
#34708=CARTESIAN_POINT('Ctrl Pts',(-1.34687054001093,-1.,-1.18625865667441));
#34709=CARTESIAN_POINT('Ctrl Pts',(-1.34687054001093,1.,-1.18625865667441));
#34710=CARTESIAN_POINT('Ctrl Pts',(-1.36088705043885,-1.,-1.1987959077932));
#34711=CARTESIAN_POINT('Ctrl Pts',(-1.36088705043885,1.,-1.1987959077932));
#34712=CARTESIAN_POINT('Ctrl Pts',(-1.37331915607905,-1.,-1.20982812925645));
#34713=CARTESIAN_POINT('Ctrl Pts',(-1.37331915607905,1.,-1.20982812925645));
#34714=CARTESIAN_POINT('Ctrl Pts',(-1.38420564527715,-1.,-1.21938737280852));
#34715=CARTESIAN_POINT('Ctrl Pts',(-1.38420564527715,1.,-1.21938737280852));
#34716=CARTESIAN_POINT('Ctrl Pts',(-1.39361389568796,-1.,-1.22752961899387));
#34717=CARTESIAN_POINT('Ctrl Pts',(-1.39361389568796,1.,-1.22752961899387));
#34718=CARTESIAN_POINT('Ctrl Pts',(-1.40164708206106,-1.,-1.23434087290423));
#34719=CARTESIAN_POINT('Ctrl Pts',(-1.40164708206106,1.,-1.23434087290423));
#34720=CARTESIAN_POINT('Ctrl Pts',(-1.40845295531283,-1.,-1.23994455029534));
#34721=CARTESIAN_POINT('Ctrl Pts',(-1.40845295531283,1.,-1.23994455029534));
#34722=CARTESIAN_POINT('Ctrl Pts',(-1.41422913175179,-1.,-1.24450600513056));
#34723=CARTESIAN_POINT('Ctrl Pts',(-1.41422913175179,1.,-1.24450600513056));
#34724=CARTESIAN_POINT('Ctrl Pts',(-1.41923722596025,-1.,-1.24824430986571));
#34725=CARTESIAN_POINT('Ctrl Pts',(-1.41923722596025,1.,-1.24824430986571));
#34726=CARTESIAN_POINT('Ctrl Pts',(-1.42378102115575,-1.,-1.2514145557001));
#34727=CARTESIAN_POINT('Ctrl Pts',(-1.42378102115575,1.,-1.2514145557001));
#34728=CARTESIAN_POINT('Ctrl Pts',(-1.42815938799387,-1.,-1.25426945222639));
#34729=CARTESIAN_POINT('Ctrl Pts',(-1.42815938799387,1.,-1.25426945222639));
#34730=CARTESIAN_POINT('Ctrl Pts',(-1.43262645609691,-1.,-1.25702687965755));
#34731=CARTESIAN_POINT('Ctrl Pts',(-1.43262645609691,1.,-1.25702687965755));
#34732=CARTESIAN_POINT('Ctrl Pts',(-1.43734919180848,-1.,-1.25983531012005));
#34733=CARTESIAN_POINT('Ctrl Pts',(-1.43734919180848,1.,-1.25983531012005));
#34734=CARTESIAN_POINT('Ctrl Pts',(-1.44236470511303,-1.,-1.26273903323859));
#34735=CARTESIAN_POINT('Ctrl Pts',(-1.44236470511303,1.,-1.26273903323859));
#34736=CARTESIAN_POINT('Ctrl Pts',(-1.44761985001662,-1.,-1.26570925118868));
#34737=CARTESIAN_POINT('Ctrl Pts',(-1.44761985001662,1.,-1.26570925118868));
#34738=CARTESIAN_POINT('Ctrl Pts',(-1.45301422764247,-1.,-1.2686778680489));
#34739=CARTESIAN_POINT('Ctrl Pts',(-1.45301422764247,1.,-1.2686778680489));
#34740=CARTESIAN_POINT('Ctrl Pts',(-1.45843906294697,-1.,-1.27156805265289));
#34741=CARTESIAN_POINT('Ctrl Pts',(-1.45843906294697,1.,-1.27156805265289));
#34742=CARTESIAN_POINT('Ctrl Pts',(-1.46382431332476,-1.,-1.27433119897822));
#34743=CARTESIAN_POINT('Ctrl Pts',(-1.46382431332476,1.,-1.27433119897822));
#34744=CARTESIAN_POINT('Ctrl Pts',(-1.46916035917133,-1.,-1.27696414831089));
#34745=CARTESIAN_POINT('Ctrl Pts',(-1.46916035917133,1.,-1.27696414831089));
#34746=CARTESIAN_POINT('Ctrl Pts',(-1.4744717526707,-1.,-1.2794891824849));
#34747=CARTESIAN_POINT('Ctrl Pts',(-1.4744717526707,1.,-1.2794891824849));
#34748=CARTESIAN_POINT('Ctrl Pts',(-1.47980070347095,-1.,-1.28194158939517));
#34749=CARTESIAN_POINT('Ctrl Pts',(-1.47980070347095,1.,-1.28194158939517));
#34750=CARTESIAN_POINT('Ctrl Pts',(-1.4851881711891,-1.,-1.28435533880201));
#34751=CARTESIAN_POINT('Ctrl Pts',(-1.4851881711891,1.,-1.28435533880201));
#34752=CARTESIAN_POINT('Ctrl Pts',(-1.4906522831278,-1.,-1.2867467611644));
#34753=CARTESIAN_POINT('Ctrl Pts',(-1.4906522831278,1.,-1.2867467611644));
#34754=CARTESIAN_POINT('Ctrl Pts',(-1.49618896881754,-1.,-1.28911506584254));
#34755=CARTESIAN_POINT('Ctrl Pts',(-1.49618896881754,1.,-1.28911506584254));
#34756=CARTESIAN_POINT('Ctrl Pts',(-1.50178230149776,-1.,-1.29145022885181));
#34757=CARTESIAN_POINT('Ctrl Pts',(-1.50178230149776,1.,-1.29145022885181));
#34758=CARTESIAN_POINT('Ctrl Pts',(-1.50741159078365,-1.,-1.29373841372842));
#34759=CARTESIAN_POINT('Ctrl Pts',(-1.50741159078365,1.,-1.29373841372842));
#34760=CARTESIAN_POINT('Ctrl Pts',(-1.51305994241402,-1.,-1.29596850710509));
#34761=CARTESIAN_POINT('Ctrl Pts',(-1.51305994241402,1.,-1.29596850710509));
#34762=CARTESIAN_POINT('Ctrl Pts',(-1.51872184912724,-1.,-1.29813791800747));
#34763=CARTESIAN_POINT('Ctrl Pts',(-1.51872184912724,1.,-1.29813791800747));
#34764=CARTESIAN_POINT('Ctrl Pts',(-1.52439957861062,-1.,-1.30024984366328));
#34765=CARTESIAN_POINT('Ctrl Pts',(-1.52439957861062,1.,-1.30024984366328));
#34766=CARTESIAN_POINT('Ctrl Pts',(-1.53009970283891,-1.,-1.30231064395568));
#34767=CARTESIAN_POINT('Ctrl Pts',(-1.53009970283891,1.,-1.30231064395568));
#34768=CARTESIAN_POINT('Ctrl Pts',(-1.53582981268977,-1.,-1.30432735639489));
#34769=CARTESIAN_POINT('Ctrl Pts',(-1.53582981268977,1.,-1.30432735639489));
#34770=CARTESIAN_POINT('Ctrl Pts',(-1.54159462645432,-1.,-1.30630475189556));
#34771=CARTESIAN_POINT('Ctrl Pts',(-1.54159462645432,1.,-1.30630475189556));
#34772=CARTESIAN_POINT('Ctrl Pts',(-1.54739413957185,-1.,-1.30824393907473));
#34773=CARTESIAN_POINT('Ctrl Pts',(-1.54739413957185,1.,-1.30824393907473));
#34774=CARTESIAN_POINT('Ctrl Pts',(-1.55322568759481,-1.,-1.31014393684222));
#34775=CARTESIAN_POINT('Ctrl Pts',(-1.55322568759481,1.,-1.31014393684222));
#34776=CARTESIAN_POINT('Ctrl Pts',(-1.55908521254821,-1.,-1.31200264341696));
#34777=CARTESIAN_POINT('Ctrl Pts',(-1.55908521254821,1.,-1.31200264341696));
#34778=CARTESIAN_POINT('Ctrl Pts',(-1.56496872402353,-1.,-1.31381795281002));
#34779=CARTESIAN_POINT('Ctrl Pts',(-1.56496872402353,1.,-1.31381795281002));
#34780=CARTESIAN_POINT('Ctrl Pts',(-1.57087397835723,-1.,-1.31558903860016));
#34781=CARTESIAN_POINT('Ctrl Pts',(-1.57087397835723,1.,-1.31558903860016));
#34782=CARTESIAN_POINT('Ctrl Pts',(-1.5768005650559,-1.,-1.31731642317187));
#34783=CARTESIAN_POINT('Ctrl Pts',(-1.5768005650559,1.,-1.31731642317187));
#34784=CARTESIAN_POINT('Ctrl Pts',(-1.58274907898834,-1.,-1.31900135021432));
#34785=CARTESIAN_POINT('Ctrl Pts',(-1.58274907898834,1.,-1.31900135021432));
#34786=CARTESIAN_POINT('Ctrl Pts',(-1.58872057258245,-1.,-1.32064537110892));
#34787=CARTESIAN_POINT('Ctrl Pts',(-1.58872057258245,1.,-1.32064537110892));
#34788=CARTESIAN_POINT('Ctrl Pts',(-1.59471591079403,-1.,-1.32224985747682));
#34789=CARTESIAN_POINT('Ctrl Pts',(-1.59471591079403,1.,-1.32224985747682));
#34790=CARTESIAN_POINT('Ctrl Pts',(-1.60073511858687,-1.,-1.32381550858256));
#34791=CARTESIAN_POINT('Ctrl Pts',(-1.60073511858687,1.,-1.32381550858256));
#34792=CARTESIAN_POINT('Ctrl Pts',(-1.60677758290954,-1.,-1.32534250785782));
#34793=CARTESIAN_POINT('Ctrl Pts',(-1.60677758290954,1.,-1.32534250785782));
#34794=CARTESIAN_POINT('Ctrl Pts',(-1.6128423401575,-1.,-1.32683074483356));
#34795=CARTESIAN_POINT('Ctrl Pts',(-1.6128423401575,1.,-1.32683074483356));
#34796=CARTESIAN_POINT('Ctrl Pts',(-1.61892832270724,-1.,-1.32828000610449));
#34797=CARTESIAN_POINT('Ctrl Pts',(-1.61892832270724,1.,-1.32828000610449));
#34798=CARTESIAN_POINT('Ctrl Pts',(-1.62503464209797,-1.,-1.3296901950568));
#34799=CARTESIAN_POINT('Ctrl Pts',(-1.62503464209797,1.,-1.3296901950568));
#34800=CARTESIAN_POINT('Ctrl Pts',(-1.63116079730923,-1.,-1.33106149345645));
#34801=CARTESIAN_POINT('Ctrl Pts',(-1.63116079730923,1.,-1.33106149345645));
#34802=CARTESIAN_POINT('Ctrl Pts',(-1.63730653475089,-1.,-1.33239425103724));
#34803=CARTESIAN_POINT('Ctrl Pts',(-1.63730653475089,1.,-1.33239425103724));
#34804=CARTESIAN_POINT('Ctrl Pts',(-1.6434717485603,-1.,-1.33368890676572));
#34805=CARTESIAN_POINT('Ctrl Pts',(-1.6434717485603,1.,-1.33368890676572));
#34806=CARTESIAN_POINT('Ctrl Pts',(-1.6496563728683,-1.,-1.33494590467993));
#34807=CARTESIAN_POINT('Ctrl Pts',(-1.6496563728683,1.,-1.33494590467993));
#34808=CARTESIAN_POINT('Ctrl Pts',(-1.65586025952593,-1.,-1.33616559745172));
#34809=CARTESIAN_POINT('Ctrl Pts',(-1.65586025952593,1.,-1.33616559745172));
#34810=CARTESIAN_POINT('Ctrl Pts',(-1.66208312541983,-1.,-1.33734820885262));
#34811=CARTESIAN_POINT('Ctrl Pts',(-1.66208312541983,1.,-1.33734820885262));
#34812=CARTESIAN_POINT('Ctrl Pts',(-1.66832460783989,-1.,-1.33849388654388));
#34813=CARTESIAN_POINT('Ctrl Pts',(-1.66832460783989,1.,-1.33849388654388));
#34814=CARTESIAN_POINT('Ctrl Pts',(-1.67458429426086,-1.,-1.3396027347034));
#34815=CARTESIAN_POINT('Ctrl Pts',(-1.67458429426086,1.,-1.3396027347034));
#34816=CARTESIAN_POINT('Ctrl Pts',(-1.68086176030362,-1.,-1.34067485185203));
#34817=CARTESIAN_POINT('Ctrl Pts',(-1.68086176030362,1.,-1.34067485185203));
#34818=CARTESIAN_POINT('Ctrl Pts',(-1.68715660868764,-1.,-1.341710374848));
#34819=CARTESIAN_POINT('Ctrl Pts',(-1.68715660868764,1.,-1.341710374848));
#34820=CARTESIAN_POINT('Ctrl Pts',(-1.6934684849687,-1.,-1.34270948206319));
#34821=CARTESIAN_POINT('Ctrl Pts',(-1.6934684849687,1.,-1.34270948206319));
#34822=CARTESIAN_POINT('Ctrl Pts',(-1.69979707754427,-1.,-1.34367237124483));
#34823=CARTESIAN_POINT('Ctrl Pts',(-1.69979707754427,1.,-1.34367237124483));
#34824=CARTESIAN_POINT('Ctrl Pts',(-1.70614212266738,-1.,-1.34459924533831));
#34825=CARTESIAN_POINT('Ctrl Pts',(-1.70614212266738,1.,-1.34459924533831));
#34826=CARTESIAN_POINT('Ctrl Pts',(-1.71250340686822,-1.,-1.34549029589416));
#34827=CARTESIAN_POINT('Ctrl Pts',(-1.71250340686822,1.,-1.34549029589416));
#34828=CARTESIAN_POINT('Ctrl Pts',(-1.7188807715049,-1.,-1.34634568653227));
#34829=CARTESIAN_POINT('Ctrl Pts',(-1.7188807715049,1.,-1.34634568653227));
#34830=CARTESIAN_POINT('Ctrl Pts',(-1.72527410680674,-1.,-1.34716554819527));
#34831=CARTESIAN_POINT('Ctrl Pts',(-1.72527410680674,1.,-1.34716554819527));
#34832=CARTESIAN_POINT('Ctrl Pts',(-1.7304014965394,-1.,-1.34779309152035));
#34833=CARTESIAN_POINT('Ctrl Pts',(-1.7304014965394,1.,-1.34779309152035));
#34834=CARTESIAN_POINT('Ctrl Pts',(-1.73425417885907,-1.,-1.34824783112887));
#34835=CARTESIAN_POINT('Ctrl Pts',(-1.73425417885907,1.,-1.34824783112887));
#34836=CARTESIAN_POINT('Ctrl Pts',(-1.73682580585691,-1.,-1.34854391898045));
#34837=CARTESIAN_POINT('Ctrl Pts',(-1.73682580585691,1.,-1.34854391898045));
#34838=CARTESIAN_POINT('Ctrl Pts',(-1.73811241238545,-1.,-1.34869019493419));
#34839=CARTESIAN_POINT('Ctrl Pts',(-1.73811241238545,1.,-1.34869019493419));
#34840=CARTESIAN_POINT('',(-1.31362392696032,1.,-1.15624053661742));
#34841=CARTESIAN_POINT('Ctrl Pts',(-1.31362392696032,1.,-1.15624053661742));
#34842=CARTESIAN_POINT('Ctrl Pts',(-1.31722977216397,1.,-1.15950888730809));
#34843=CARTESIAN_POINT('Ctrl Pts',(-1.32428080721772,1.,-1.16589330093588));
#34844=CARTESIAN_POINT('Ctrl Pts',(-1.33437539347008,1.,-1.17501305789857));
#34845=CARTESIAN_POINT('Ctrl Pts',(-1.34687054001093,1.,-1.18625865667441));
#34846=CARTESIAN_POINT('Ctrl Pts',(-1.36088705043885,1.,-1.1987959077932));
#34847=CARTESIAN_POINT('Ctrl Pts',(-1.37331915607905,1.,-1.20982812925645));
#34848=CARTESIAN_POINT('Ctrl Pts',(-1.38420564527715,1.,-1.21938737280852));
#34849=CARTESIAN_POINT('Ctrl Pts',(-1.39361389568796,1.,-1.22752961899387));
#34850=CARTESIAN_POINT('Ctrl Pts',(-1.40164708206106,1.,-1.23434087290423));
#34851=CARTESIAN_POINT('Ctrl Pts',(-1.40845295531283,1.,-1.23994455029534));
#34852=CARTESIAN_POINT('Ctrl Pts',(-1.41422913175179,1.,-1.24450600513056));
#34853=CARTESIAN_POINT('Ctrl Pts',(-1.41923722596025,1.,-1.24824430986571));
#34854=CARTESIAN_POINT('Ctrl Pts',(-1.42378102115575,1.,-1.2514145557001));
#34855=CARTESIAN_POINT('Ctrl Pts',(-1.42815938799387,1.,-1.25426945222639));
#34856=CARTESIAN_POINT('Ctrl Pts',(-1.43262645609691,1.,-1.25702687965755));
#34857=CARTESIAN_POINT('Ctrl Pts',(-1.43734919180848,1.,-1.25983531012005));
#34858=CARTESIAN_POINT('Ctrl Pts',(-1.44236470511303,1.,-1.26273903323859));
#34859=CARTESIAN_POINT('Ctrl Pts',(-1.44761985001662,1.,-1.26570925118868));
#34860=CARTESIAN_POINT('Ctrl Pts',(-1.45301422764247,1.,-1.2686778680489));
#34861=CARTESIAN_POINT('Ctrl Pts',(-1.45843906294697,1.,-1.27156805265289));
#34862=CARTESIAN_POINT('Ctrl Pts',(-1.46382431332476,1.,-1.27433119897822));
#34863=CARTESIAN_POINT('Ctrl Pts',(-1.46916035917133,1.,-1.27696414831089));
#34864=CARTESIAN_POINT('Ctrl Pts',(-1.4744717526707,1.,-1.2794891824849));
#34865=CARTESIAN_POINT('Ctrl Pts',(-1.47980070347095,1.,-1.28194158939517));
#34866=CARTESIAN_POINT('Ctrl Pts',(-1.4851881711891,1.,-1.28435533880201));
#34867=CARTESIAN_POINT('Ctrl Pts',(-1.4906522831278,1.,-1.2867467611644));
#34868=CARTESIAN_POINT('Ctrl Pts',(-1.49618896881754,1.,-1.28911506584254));
#34869=CARTESIAN_POINT('Ctrl Pts',(-1.50178230149776,1.,-1.29145022885181));
#34870=CARTESIAN_POINT('Ctrl Pts',(-1.50741159078365,1.,-1.29373841372842));
#34871=CARTESIAN_POINT('Ctrl Pts',(-1.51305994241402,1.,-1.29596850710509));
#34872=CARTESIAN_POINT('Ctrl Pts',(-1.51872184912724,1.,-1.29813791800747));
#34873=CARTESIAN_POINT('Ctrl Pts',(-1.52439957861062,1.,-1.30024984366328));
#34874=CARTESIAN_POINT('Ctrl Pts',(-1.53009970283891,1.,-1.30231064395568));
#34875=CARTESIAN_POINT('Ctrl Pts',(-1.53582981268977,1.,-1.30432735639489));
#34876=CARTESIAN_POINT('Ctrl Pts',(-1.54159462645432,1.,-1.30630475189556));
#34877=CARTESIAN_POINT('Ctrl Pts',(-1.54739413957185,1.,-1.30824393907473));
#34878=CARTESIAN_POINT('Ctrl Pts',(-1.55322568759481,1.,-1.31014393684222));
#34879=CARTESIAN_POINT('Ctrl Pts',(-1.55908521254821,1.,-1.31200264341696));
#34880=CARTESIAN_POINT('Ctrl Pts',(-1.56496872402353,1.,-1.31381795281002));
#34881=CARTESIAN_POINT('Ctrl Pts',(-1.57087397835723,1.,-1.31558903860016));
#34882=CARTESIAN_POINT('Ctrl Pts',(-1.5768005650559,1.,-1.31731642317187));
#34883=CARTESIAN_POINT('Ctrl Pts',(-1.58274907898834,1.,-1.31900135021432));
#34884=CARTESIAN_POINT('Ctrl Pts',(-1.58872057258245,1.,-1.32064537110892));
#34885=CARTESIAN_POINT('Ctrl Pts',(-1.59471591079403,1.,-1.32224985747682));
#34886=CARTESIAN_POINT('Ctrl Pts',(-1.60073511858687,1.,-1.32381550858256));
#34887=CARTESIAN_POINT('Ctrl Pts',(-1.60677758290954,1.,-1.32534250785782));
#34888=CARTESIAN_POINT('Ctrl Pts',(-1.6128423401575,1.,-1.32683074483356));
#34889=CARTESIAN_POINT('Ctrl Pts',(-1.61892832270724,1.,-1.32828000610449));
#34890=CARTESIAN_POINT('Ctrl Pts',(-1.62503464209797,1.,-1.3296901950568));
#34891=CARTESIAN_POINT('Ctrl Pts',(-1.63116079730923,1.,-1.33106149345645));
#34892=CARTESIAN_POINT('Ctrl Pts',(-1.63730653475089,1.,-1.33239425103724));
#34893=CARTESIAN_POINT('Ctrl Pts',(-1.6434717485603,1.,-1.33368890676572));
#34894=CARTESIAN_POINT('Ctrl Pts',(-1.6496563728683,1.,-1.33494590467993));
#34895=CARTESIAN_POINT('Ctrl Pts',(-1.65586025952593,1.,-1.33616559745172));
#34896=CARTESIAN_POINT('Ctrl Pts',(-1.66208312541983,1.,-1.33734820885262));
#34897=CARTESIAN_POINT('Ctrl Pts',(-1.66832460783989,1.,-1.33849388654388));
#34898=CARTESIAN_POINT('Ctrl Pts',(-1.67458429426086,1.,-1.3396027347034));
#34899=CARTESIAN_POINT('Ctrl Pts',(-1.68086176030362,1.,-1.34067485185203));
#34900=CARTESIAN_POINT('Ctrl Pts',(-1.68715660868764,1.,-1.341710374848));
#34901=CARTESIAN_POINT('Ctrl Pts',(-1.6934684849687,1.,-1.34270948206319));
#34902=CARTESIAN_POINT('Ctrl Pts',(-1.69979707754427,1.,-1.34367237124483));
#34903=CARTESIAN_POINT('Ctrl Pts',(-1.70614212266738,1.,-1.34459924533831));
#34904=CARTESIAN_POINT('Ctrl Pts',(-1.71250340686822,1.,-1.34549029589416));
#34905=CARTESIAN_POINT('Ctrl Pts',(-1.7188807715049,1.,-1.34634568653227));
#34906=CARTESIAN_POINT('Ctrl Pts',(-1.72527410680674,1.,-1.34716554819527));
#34907=CARTESIAN_POINT('Ctrl Pts',(-1.7304014965394,1.,-1.34779309152035));
#34908=CARTESIAN_POINT('Ctrl Pts',(-1.73425417885907,1.,-1.34824783112887));
#34909=CARTESIAN_POINT('Ctrl Pts',(-1.73682580585691,1.,-1.34854391898045));
#34910=CARTESIAN_POINT('Ctrl Pts',(-1.73811241238545,1.,-1.34869019493419));
#34911=CARTESIAN_POINT('',(-1.31362392696032,0.,-1.15624053661742));
#34912=CARTESIAN_POINT('Origin',(0.,0.,0.));
#34913=CARTESIAN_POINT('',(-1.15624053661742,1.,-1.31362392696033));
#34914=CARTESIAN_POINT('Origin',(0.,1.,0.));
#34915=CARTESIAN_POINT('',(-1.15624053661742,0.,-1.31362392696033));
#34916=CARTESIAN_POINT('Ctrl Pts',(-1.34869019493419,-1.,-1.73811241238545));
#34917=CARTESIAN_POINT('Ctrl Pts',(-1.34869019493419,1.,-1.73811241238545));
#34918=CARTESIAN_POINT('Ctrl Pts',(-1.34854391898145,-1.,-1.73682580585819));
#34919=CARTESIAN_POINT('Ctrl Pts',(-1.34854391898145,1.,-1.73682580585819));
#34920=CARTESIAN_POINT('Ctrl Pts',(-1.34824783113158,-1.,-1.73425417886255));
#34921=CARTESIAN_POINT('Ctrl Pts',(-1.34824783113158,1.,-1.73425417886255));
#34922=CARTESIAN_POINT('Ctrl Pts',(-1.3477930915247,-1.,-1.73040149654497));
#34923=CARTESIAN_POINT('Ctrl Pts',(-1.3477930915247,1.,-1.73040149654497));
#34924=CARTESIAN_POINT('Ctrl Pts',(-1.34716554820013,-1.,-1.72527410681298));
#34925=CARTESIAN_POINT('Ctrl Pts',(-1.34716554820013,1.,-1.72527410681298));
#34926=CARTESIAN_POINT('Ctrl Pts',(-1.34634568653586,-1.,-1.7188807715095));
#34927=CARTESIAN_POINT('Ctrl Pts',(-1.34634568653586,1.,-1.7188807715095));
#34928=CARTESIAN_POINT('Ctrl Pts',(-1.34549029589563,-1.,-1.71250340687011));
#34929=CARTESIAN_POINT('Ctrl Pts',(-1.34549029589563,1.,-1.71250340687011));
#34930=CARTESIAN_POINT('Ctrl Pts',(-1.34459924533783,-1.,-1.70614212266676));
#34931=CARTESIAN_POINT('Ctrl Pts',(-1.34459924533783,1.,-1.70614212266676));
#34932=CARTESIAN_POINT('Ctrl Pts',(-1.34367237124322,-1.,-1.69979707754221));
#34933=CARTESIAN_POINT('Ctrl Pts',(-1.34367237124322,1.,-1.69979707754221));
#34934=CARTESIAN_POINT('Ctrl Pts',(-1.34270948206139,-1.,-1.6934684849664));
#34935=CARTESIAN_POINT('Ctrl Pts',(-1.34270948206139,1.,-1.6934684849664));
#34936=CARTESIAN_POINT('Ctrl Pts',(-1.34171037484673,-1.,-1.68715660868602));
#34937=CARTESIAN_POINT('Ctrl Pts',(-1.34171037484673,1.,-1.68715660868602));
#34938=CARTESIAN_POINT('Ctrl Pts',(-1.3406748518516,-1.,-1.68086176030308));
#34939=CARTESIAN_POINT('Ctrl Pts',(-1.3406748518516,1.,-1.68086176030308));
#34940=CARTESIAN_POINT('Ctrl Pts',(-1.33960273470372,-1.,-1.67458429426126));
#34941=CARTESIAN_POINT('Ctrl Pts',(-1.33960273470372,1.,-1.67458429426126));
#34942=CARTESIAN_POINT('Ctrl Pts',(-1.33849388654458,-1.,-1.66832460784078));
#34943=CARTESIAN_POINT('Ctrl Pts',(-1.33849388654458,1.,-1.66832460784078));
#34944=CARTESIAN_POINT('Ctrl Pts',(-1.33734820885331,-1.,-1.66208312542073));
#34945=CARTESIAN_POINT('Ctrl Pts',(-1.33734820885331,1.,-1.66208312542073));
#34946=CARTESIAN_POINT('Ctrl Pts',(-1.33616559745217,-1.,-1.65586025952651));
#34947=CARTESIAN_POINT('Ctrl Pts',(-1.33616559745217,1.,-1.65586025952651));
#34948=CARTESIAN_POINT('Ctrl Pts',(-1.33494590468003,-1.,-1.64965637286843));
#34949=CARTESIAN_POINT('Ctrl Pts',(-1.33494590468003,1.,-1.64965637286843));
#34950=CARTESIAN_POINT('Ctrl Pts',(-1.33368890676554,-1.,-1.64347174856007));
#34951=CARTESIAN_POINT('Ctrl Pts',(-1.33368890676554,1.,-1.64347174856007));
#34952=CARTESIAN_POINT('Ctrl Pts',(-1.33239425103694,-1.,-1.6373065347505));
#34953=CARTESIAN_POINT('Ctrl Pts',(-1.33239425103694,1.,-1.6373065347505));
#34954=CARTESIAN_POINT('Ctrl Pts',(-1.33106149345618,-1.,-1.63116079730887));
#34955=CARTESIAN_POINT('Ctrl Pts',(-1.33106149345618,1.,-1.63116079730887));
#34956=CARTESIAN_POINT('Ctrl Pts',(-1.32969019505665,-1.,-1.62503464209777));
#34957=CARTESIAN_POINT('Ctrl Pts',(-1.32969019505665,1.,-1.62503464209777));
#34958=CARTESIAN_POINT('Ctrl Pts',(-1.32828000610448,-1.,-1.61892832270723));
#34959=CARTESIAN_POINT('Ctrl Pts',(-1.32828000610448,1.,-1.61892832270723));
#34960=CARTESIAN_POINT('Ctrl Pts',(-1.32683074483365,-1.,-1.61284234015762));
#34961=CARTESIAN_POINT('Ctrl Pts',(-1.32683074483365,1.,-1.61284234015762));
#34962=CARTESIAN_POINT('Ctrl Pts',(-1.32534250785794,-1.,-1.6067775829097));
#34963=CARTESIAN_POINT('Ctrl Pts',(-1.32534250785794,1.,-1.6067775829097));
#34964=CARTESIAN_POINT('Ctrl Pts',(-1.32381550858266,-1.,-1.600735118587));
#34965=CARTESIAN_POINT('Ctrl Pts',(-1.32381550858266,1.,-1.600735118587));
#34966=CARTESIAN_POINT('Ctrl Pts',(-1.32224985747686,-1.,-1.59471591079408));
#34967=CARTESIAN_POINT('Ctrl Pts',(-1.32224985747686,1.,-1.59471591079408));
#34968=CARTESIAN_POINT('Ctrl Pts',(-1.32064537110891,-1.,-1.58872057258244));
#34969=CARTESIAN_POINT('Ctrl Pts',(-1.32064537110891,1.,-1.58872057258244));
#34970=CARTESIAN_POINT('Ctrl Pts',(-1.31900135021428,-1.,-1.58274907898829));
#34971=CARTESIAN_POINT('Ctrl Pts',(-1.31900135021428,1.,-1.58274907898829));
#34972=CARTESIAN_POINT('Ctrl Pts',(-1.31731642317183,-1.,-1.57680056505585));
#34973=CARTESIAN_POINT('Ctrl Pts',(-1.31731642317183,1.,-1.57680056505585));
#34974=CARTESIAN_POINT('Ctrl Pts',(-1.31558903860015,-1.,-1.57087397835721));
#34975=CARTESIAN_POINT('Ctrl Pts',(-1.31558903860015,1.,-1.57087397835721));
#34976=CARTESIAN_POINT('Ctrl Pts',(-1.31381795281002,-1.,-1.56496872402352));
#34977=CARTESIAN_POINT('Ctrl Pts',(-1.31381795281002,1.,-1.56496872402352));
#34978=CARTESIAN_POINT('Ctrl Pts',(-1.31200264341696,-1.,-1.55908521254822));
#34979=CARTESIAN_POINT('Ctrl Pts',(-1.31200264341696,1.,-1.55908521254822));
#34980=CARTESIAN_POINT('Ctrl Pts',(-1.31014393684221,-1.,-1.55322568759481));
#34981=CARTESIAN_POINT('Ctrl Pts',(-1.31014393684221,1.,-1.55322568759481));
#34982=CARTESIAN_POINT('Ctrl Pts',(-1.30824393907471,-1.,-1.54739413957183));
#34983=CARTESIAN_POINT('Ctrl Pts',(-1.30824393907471,1.,-1.54739413957183));
#34984=CARTESIAN_POINT('Ctrl Pts',(-1.30630475189553,-1.,-1.54159462645428));
#34985=CARTESIAN_POINT('Ctrl Pts',(-1.30630475189553,1.,-1.54159462645428));
#34986=CARTESIAN_POINT('Ctrl Pts',(-1.30432735639487,-1.,-1.53582981268976));
#34987=CARTESIAN_POINT('Ctrl Pts',(-1.30432735639487,1.,-1.53582981268976));
#34988=CARTESIAN_POINT('Ctrl Pts',(-1.3023106439557,-1.,-1.53009970283893));
#34989=CARTESIAN_POINT('Ctrl Pts',(-1.3023106439557,1.,-1.53009970283893));
#34990=CARTESIAN_POINT('Ctrl Pts',(-1.30024984366334,-1.,-1.5243995786107));
#34991=CARTESIAN_POINT('Ctrl Pts',(-1.30024984366334,1.,-1.5243995786107));
#34992=CARTESIAN_POINT('Ctrl Pts',(-1.29813791800757,-1.,-1.51872184912735));
#34993=CARTESIAN_POINT('Ctrl Pts',(-1.29813791800757,1.,-1.51872184912735));
#34994=CARTESIAN_POINT('Ctrl Pts',(-1.29596850710518,-1.,-1.51305994241412));
#34995=CARTESIAN_POINT('Ctrl Pts',(-1.29596850710518,1.,-1.51305994241412));
#34996=CARTESIAN_POINT('Ctrl Pts',(-1.29373841372843,-1.,-1.50741159078367));
#34997=CARTESIAN_POINT('Ctrl Pts',(-1.29373841372843,1.,-1.50741159078367));
#34998=CARTESIAN_POINT('Ctrl Pts',(-1.29145022885171,-1.,-1.50178230149764));
#34999=CARTESIAN_POINT('Ctrl Pts',(-1.29145022885171,1.,-1.50178230149764));
#35000=CARTESIAN_POINT('Ctrl Pts',(-1.28911506584232,-1.,-1.49618896881729));
#35001=CARTESIAN_POINT('Ctrl Pts',(-1.28911506584232,1.,-1.49618896881729));
#35002=CARTESIAN_POINT('Ctrl Pts',(-1.28674676116415,-1.,-1.4906522831275));
#35003=CARTESIAN_POINT('Ctrl Pts',(-1.28674676116415,1.,-1.4906522831275));
#35004=CARTESIAN_POINT('Ctrl Pts',(-1.28435533880184,-1.,-1.48518817118891));
#35005=CARTESIAN_POINT('Ctrl Pts',(-1.28435533880184,1.,-1.48518817118891));
#35006=CARTESIAN_POINT('Ctrl Pts',(-1.28194158939522,-1.,-1.47980070347102));
#35007=CARTESIAN_POINT('Ctrl Pts',(-1.28194158939522,1.,-1.47980070347102));
#35008=CARTESIAN_POINT('Ctrl Pts',(-1.27948918248524,-1.,-1.4744717526711));
#35009=CARTESIAN_POINT('Ctrl Pts',(-1.27948918248524,1.,-1.4744717526711));
#35010=CARTESIAN_POINT('Ctrl Pts',(-1.27696414831144,-1.,-1.46916035917197));
#35011=CARTESIAN_POINT('Ctrl Pts',(-1.27696414831144,1.,-1.46916035917197));
#35012=CARTESIAN_POINT('Ctrl Pts',(-1.27433119897877,-1.,-1.4638243133254));
#35013=CARTESIAN_POINT('Ctrl Pts',(-1.27433119897877,1.,-1.4638243133254));
#35014=CARTESIAN_POINT('Ctrl Pts',(-1.27156805265312,-1.,-1.45843906294725));
#35015=CARTESIAN_POINT('Ctrl Pts',(-1.27156805265312,1.,-1.45843906294725));
#35016=CARTESIAN_POINT('Ctrl Pts',(-1.26867786804854,-1.,-1.45301422764205));
#35017=CARTESIAN_POINT('Ctrl Pts',(-1.26867786804854,1.,-1.45301422764205));
#35018=CARTESIAN_POINT('Ctrl Pts',(-1.26570925118767,-1.,-1.44761985001544));
#35019=CARTESIAN_POINT('Ctrl Pts',(-1.26570925118767,1.,-1.44761985001544));
#35020=CARTESIAN_POINT('Ctrl Pts',(-1.26273903323723,-1.,-1.44236470511145));
#35021=CARTESIAN_POINT('Ctrl Pts',(-1.26273903323723,1.,-1.44236470511145));
#35022=CARTESIAN_POINT('Ctrl Pts',(-1.25983531011894,-1.,-1.43734919180719));
#35023=CARTESIAN_POINT('Ctrl Pts',(-1.25983531011894,1.,-1.43734919180719));
#35024=CARTESIAN_POINT('Ctrl Pts',(-1.25702687965744,-1.,-1.43262645609679));
#35025=CARTESIAN_POINT('Ctrl Pts',(-1.25702687965744,1.,-1.43262645609679));
#35026=CARTESIAN_POINT('Ctrl Pts',(-1.25426945222783,-1.,-1.42815938799555));
#35027=CARTESIAN_POINT('Ctrl Pts',(-1.25426945222783,1.,-1.42815938799555));
#35028=CARTESIAN_POINT('Ctrl Pts',(-1.25141455570299,-1.,-1.42378102115911));
#35029=CARTESIAN_POINT('Ctrl Pts',(-1.25141455570299,1.,-1.42378102115911));
#35030=CARTESIAN_POINT('Ctrl Pts',(-1.24824430986911,-1.,-1.41923722596421));
#35031=CARTESIAN_POINT('Ctrl Pts',(-1.24824430986911,1.,-1.41923722596421));
#35032=CARTESIAN_POINT('Ctrl Pts',(-1.24450600513278,-1.,-1.41422913175437));
#35033=CARTESIAN_POINT('Ctrl Pts',(-1.24450600513278,1.,-1.41422913175437));
#35034=CARTESIAN_POINT('Ctrl Pts',(-1.23994455029421,-1.,-1.40845295531151));
#35035=CARTESIAN_POINT('Ctrl Pts',(-1.23994455029421,1.,-1.40845295531151));
#35036=CARTESIAN_POINT('Ctrl Pts',(-1.23434087289768,-1.,-1.40164708205345));
#35037=CARTESIAN_POINT('Ctrl Pts',(-1.23434087289768,1.,-1.40164708205345));
#35038=CARTESIAN_POINT('Ctrl Pts',(-1.22752961898063,-1.,-1.39361389567257));
#35039=CARTESIAN_POINT('Ctrl Pts',(-1.22752961898063,1.,-1.39361389567257));
#35040=CARTESIAN_POINT('Ctrl Pts',(-1.21938737278853,-1.,-1.38420564525391));
#35041=CARTESIAN_POINT('Ctrl Pts',(-1.21938737278853,1.,-1.38420564525391));
#35042=CARTESIAN_POINT('Ctrl Pts',(-1.20982812923113,-1.,-1.37331915604962));
#35043=CARTESIAN_POINT('Ctrl Pts',(-1.20982812923113,1.,-1.37331915604962));
#35044=CARTESIAN_POINT('Ctrl Pts',(-1.1987959077656,-1.,-1.36088705040677));
#35045=CARTESIAN_POINT('Ctrl Pts',(-1.1987959077656,1.,-1.36088705040677));
#35046=CARTESIAN_POINT('Ctrl Pts',(-1.18625865664915,-1.,-1.34687053998157));
#35047=CARTESIAN_POINT('Ctrl Pts',(-1.18625865664915,1.,-1.34687053998157));
#35048=CARTESIAN_POINT('Ctrl Pts',(-1.17501305787994,-1.,-1.33437539344842));
#35049=CARTESIAN_POINT('Ctrl Pts',(-1.17501305787994,1.,-1.33437539344842));
#35050=CARTESIAN_POINT('Ctrl Pts',(-1.16589330092532,-1.,-1.32428080720544));
#35051=CARTESIAN_POINT('Ctrl Pts',(-1.16589330092532,1.,-1.32428080720544));
#35052=CARTESIAN_POINT('Ctrl Pts',(-1.15950888730433,-1.,-1.3172297721596));
#35053=CARTESIAN_POINT('Ctrl Pts',(-1.15950888730433,1.,-1.3172297721596));
#35054=CARTESIAN_POINT('Ctrl Pts',(-1.15624053661742,-1.,-1.31362392696033));
#35055=CARTESIAN_POINT('Ctrl Pts',(-1.15624053661742,1.,-1.31362392696033));
#35056=CARTESIAN_POINT('',(-1.34869019493419,1.,-1.73811241238545));
#35057=CARTESIAN_POINT('Ctrl Pts',(-1.34869019493419,1.,-1.73811241238545));
#35058=CARTESIAN_POINT('Ctrl Pts',(-1.34854391898145,1.,-1.73682580585819));
#35059=CARTESIAN_POINT('Ctrl Pts',(-1.34824783113158,1.,-1.73425417886255));
#35060=CARTESIAN_POINT('Ctrl Pts',(-1.3477930915247,1.,-1.73040149654497));
#35061=CARTESIAN_POINT('Ctrl Pts',(-1.34716554820013,1.,-1.72527410681298));
#35062=CARTESIAN_POINT('Ctrl Pts',(-1.34634568653586,1.,-1.7188807715095));
#35063=CARTESIAN_POINT('Ctrl Pts',(-1.34549029589563,1.,-1.71250340687011));
#35064=CARTESIAN_POINT('Ctrl Pts',(-1.34459924533783,1.,-1.70614212266676));
#35065=CARTESIAN_POINT('Ctrl Pts',(-1.34367237124322,1.,-1.69979707754221));
#35066=CARTESIAN_POINT('Ctrl Pts',(-1.34270948206139,1.,-1.6934684849664));
#35067=CARTESIAN_POINT('Ctrl Pts',(-1.34171037484673,1.,-1.68715660868602));
#35068=CARTESIAN_POINT('Ctrl Pts',(-1.3406748518516,1.,-1.68086176030308));
#35069=CARTESIAN_POINT('Ctrl Pts',(-1.33960273470372,1.,-1.67458429426126));
#35070=CARTESIAN_POINT('Ctrl Pts',(-1.33849388654458,1.,-1.66832460784078));
#35071=CARTESIAN_POINT('Ctrl Pts',(-1.33734820885331,1.,-1.66208312542073));
#35072=CARTESIAN_POINT('Ctrl Pts',(-1.33616559745217,1.,-1.65586025952651));
#35073=CARTESIAN_POINT('Ctrl Pts',(-1.33494590468003,1.,-1.64965637286843));
#35074=CARTESIAN_POINT('Ctrl Pts',(-1.33368890676554,1.,-1.64347174856007));
#35075=CARTESIAN_POINT('Ctrl Pts',(-1.33239425103694,1.,-1.6373065347505));
#35076=CARTESIAN_POINT('Ctrl Pts',(-1.33106149345618,1.,-1.63116079730887));
#35077=CARTESIAN_POINT('Ctrl Pts',(-1.32969019505665,1.,-1.62503464209777));
#35078=CARTESIAN_POINT('Ctrl Pts',(-1.32828000610448,1.,-1.61892832270723));
#35079=CARTESIAN_POINT('Ctrl Pts',(-1.32683074483365,1.,-1.61284234015762));
#35080=CARTESIAN_POINT('Ctrl Pts',(-1.32534250785794,1.,-1.6067775829097));
#35081=CARTESIAN_POINT('Ctrl Pts',(-1.32381550858266,1.,-1.600735118587));
#35082=CARTESIAN_POINT('Ctrl Pts',(-1.32224985747686,1.,-1.59471591079408));
#35083=CARTESIAN_POINT('Ctrl Pts',(-1.32064537110891,1.,-1.58872057258244));
#35084=CARTESIAN_POINT('Ctrl Pts',(-1.31900135021428,1.,-1.58274907898829));
#35085=CARTESIAN_POINT('Ctrl Pts',(-1.31731642317183,1.,-1.57680056505585));
#35086=CARTESIAN_POINT('Ctrl Pts',(-1.31558903860015,1.,-1.57087397835721));
#35087=CARTESIAN_POINT('Ctrl Pts',(-1.31381795281002,1.,-1.56496872402352));
#35088=CARTESIAN_POINT('Ctrl Pts',(-1.31200264341696,1.,-1.55908521254822));
#35089=CARTESIAN_POINT('Ctrl Pts',(-1.31014393684221,1.,-1.55322568759481));
#35090=CARTESIAN_POINT('Ctrl Pts',(-1.30824393907471,1.,-1.54739413957183));
#35091=CARTESIAN_POINT('Ctrl Pts',(-1.30630475189553,1.,-1.54159462645428));
#35092=CARTESIAN_POINT('Ctrl Pts',(-1.30432735639487,1.,-1.53582981268976));
#35093=CARTESIAN_POINT('Ctrl Pts',(-1.3023106439557,1.,-1.53009970283893));
#35094=CARTESIAN_POINT('Ctrl Pts',(-1.30024984366334,1.,-1.5243995786107));
#35095=CARTESIAN_POINT('Ctrl Pts',(-1.29813791800757,1.,-1.51872184912735));
#35096=CARTESIAN_POINT('Ctrl Pts',(-1.29596850710518,1.,-1.51305994241412));
#35097=CARTESIAN_POINT('Ctrl Pts',(-1.29373841372843,1.,-1.50741159078367));
#35098=CARTESIAN_POINT('Ctrl Pts',(-1.29145022885171,1.,-1.50178230149764));
#35099=CARTESIAN_POINT('Ctrl Pts',(-1.28911506584232,1.,-1.49618896881729));
#35100=CARTESIAN_POINT('Ctrl Pts',(-1.28674676116415,1.,-1.4906522831275));
#35101=CARTESIAN_POINT('Ctrl Pts',(-1.28435533880184,1.,-1.48518817118891));
#35102=CARTESIAN_POINT('Ctrl Pts',(-1.28194158939522,1.,-1.47980070347102));
#35103=CARTESIAN_POINT('Ctrl Pts',(-1.27948918248524,1.,-1.4744717526711));
#35104=CARTESIAN_POINT('Ctrl Pts',(-1.27696414831144,1.,-1.46916035917197));
#35105=CARTESIAN_POINT('Ctrl Pts',(-1.27433119897877,1.,-1.4638243133254));
#35106=CARTESIAN_POINT('Ctrl Pts',(-1.27156805265312,1.,-1.45843906294725));
#35107=CARTESIAN_POINT('Ctrl Pts',(-1.26867786804854,1.,-1.45301422764205));
#35108=CARTESIAN_POINT('Ctrl Pts',(-1.26570925118767,1.,-1.44761985001544));
#35109=CARTESIAN_POINT('Ctrl Pts',(-1.26273903323723,1.,-1.44236470511145));
#35110=CARTESIAN_POINT('Ctrl Pts',(-1.25983531011894,1.,-1.43734919180719));
#35111=CARTESIAN_POINT('Ctrl Pts',(-1.25702687965744,1.,-1.43262645609679));
#35112=CARTESIAN_POINT('Ctrl Pts',(-1.25426945222783,1.,-1.42815938799555));
#35113=CARTESIAN_POINT('Ctrl Pts',(-1.25141455570299,1.,-1.42378102115911));
#35114=CARTESIAN_POINT('Ctrl Pts',(-1.24824430986911,1.,-1.41923722596421));
#35115=CARTESIAN_POINT('Ctrl Pts',(-1.24450600513278,1.,-1.41422913175437));
#35116=CARTESIAN_POINT('Ctrl Pts',(-1.23994455029421,1.,-1.40845295531151));
#35117=CARTESIAN_POINT('Ctrl Pts',(-1.23434087289768,1.,-1.40164708205345));
#35118=CARTESIAN_POINT('Ctrl Pts',(-1.22752961898063,1.,-1.39361389567257));
#35119=CARTESIAN_POINT('Ctrl Pts',(-1.21938737278853,1.,-1.38420564525391));
#35120=CARTESIAN_POINT('Ctrl Pts',(-1.20982812923113,1.,-1.37331915604962));
#35121=CARTESIAN_POINT('Ctrl Pts',(-1.1987959077656,1.,-1.36088705040677));
#35122=CARTESIAN_POINT('Ctrl Pts',(-1.18625865664915,1.,-1.34687053998157));
#35123=CARTESIAN_POINT('Ctrl Pts',(-1.17501305787994,1.,-1.33437539344842));
#35124=CARTESIAN_POINT('Ctrl Pts',(-1.16589330092532,1.,-1.32428080720544));
#35125=CARTESIAN_POINT('Ctrl Pts',(-1.15950888730433,1.,-1.3172297721596));
#35126=CARTESIAN_POINT('Ctrl Pts',(-1.15624053661742,1.,-1.31362392696033));
#35127=CARTESIAN_POINT('',(-1.34869019493419,0.,-1.73811241238545));
#35128=CARTESIAN_POINT('Origin',(-1.23627494547115,0.,-1.81978687191668));
#35129=CARTESIAN_POINT('',(-1.23627494547115,1.,-1.81978687191668));
#35130=CARTESIAN_POINT('',(-1.34869019493419,1.,-1.73811241238545));
#35131=CARTESIAN_POINT('',(-1.23627494547115,0.,-1.81978687191668));
#35132=CARTESIAN_POINT('Ctrl Pts',(-0.892032620296855,-1.,-1.5055822144029));
#35133=CARTESIAN_POINT('Ctrl Pts',(-0.892032620296855,1.,-1.5055822144029));
#35134=CARTESIAN_POINT('Ctrl Pts',(-0.894452006967538,-1.,-1.50980486807181));
#35135=CARTESIAN_POINT('Ctrl Pts',(-0.894452006967538,1.,-1.50980486807181));
#35136=CARTESIAN_POINT('Ctrl Pts',(-0.89918504749193,-1.,-1.51805569591479));
#35137=CARTESIAN_POINT('Ctrl Pts',(-0.89918504749193,1.,-1.51805569591479));
#35138=CARTESIAN_POINT('Ctrl Pts',(-0.905967409640499,-1.,-1.52984849890434));
#35139=CARTESIAN_POINT('Ctrl Pts',(-0.905967409640499,1.,-1.52984849890434));
#35140=CARTESIAN_POINT('Ctrl Pts',(-0.91437591904658,-1.,-1.54440491152808));
#35141=CARTESIAN_POINT('Ctrl Pts',(-0.91437591904658,1.,-1.54440491152808));
#35142=CARTESIAN_POINT('Ctrl Pts',(-0.923832188966322,-1.,-1.56065988582509));
#35143=CARTESIAN_POINT('Ctrl Pts',(-0.923832188966322,1.,-1.56065988582509));
#35144=CARTESIAN_POINT('Ctrl Pts',(-0.932246680128849,-1.,-1.57499388385561));
#35145=CARTESIAN_POINT('Ctrl Pts',(-0.932246680128849,1.,-1.57499388385561));
#35146=CARTESIAN_POINT('Ctrl Pts',(-0.939646377909319,-1.,-1.58744937489796));
#35147=CARTESIAN_POINT('Ctrl Pts',(-0.939646377909319,1.,-1.58744937489796));
#35148=CARTESIAN_POINT('Ctrl Pts',(-0.946078063325796,-1.,-1.59810042045408));
#35149=CARTESIAN_POINT('Ctrl Pts',(-0.946078063325796,1.,-1.59810042045408));
#35150=CARTESIAN_POINT('Ctrl Pts',(-0.951613284361248,-1.,-1.60706069897794));
#35151=CARTESIAN_POINT('Ctrl Pts',(-0.951613284361248,1.,-1.60706069897794));
#35152=CARTESIAN_POINT('Ctrl Pts',(-0.956354422921573,-1.,-1.61449324337233));
#35153=CARTESIAN_POINT('Ctrl Pts',(-0.956354422921573,1.,-1.61449324337233));
#35154=CARTESIAN_POINT('Ctrl Pts',(-0.960438326099958,-1.,-1.62061638139929));
#35155=CARTESIAN_POINT('Ctrl Pts',(-0.960438326099958,1.,-1.62061638139929));
#35156=CARTESIAN_POINT('Ctrl Pts',(-0.964046107037821,-1.,-1.6257193066974));
#35157=CARTESIAN_POINT('Ctrl Pts',(-0.964046107037821,1.,-1.6257193066974));
#35158=CARTESIAN_POINT('Ctrl Pts',(-0.967387853228041,-1.,-1.63013849959083));
#35159=CARTESIAN_POINT('Ctrl Pts',(-0.967387853228041,1.,-1.63013849959083));
#35160=CARTESIAN_POINT('Ctrl Pts',(-0.970669715996356,-1.,-1.63420665729609));
#35161=CARTESIAN_POINT('Ctrl Pts',(-0.970669715996356,1.,-1.63420665729609));
#35162=CARTESIAN_POINT('Ctrl Pts',(-0.974066058287501,-1.,-1.63820952658157));
#35163=CARTESIAN_POINT('Ctrl Pts',(-0.974066058287501,1.,-1.63820952658157));
#35164=CARTESIAN_POINT('Ctrl Pts',(-0.977689794120297,-1.,-1.64233990826831));
#35165=CARTESIAN_POINT('Ctrl Pts',(-0.977689794120297,1.,-1.64233990826831));
#35166=CARTESIAN_POINT('Ctrl Pts',(-0.981562530940574,-1.,-1.64665139190834));
#35167=CARTESIAN_POINT('Ctrl Pts',(-0.981562530940574,1.,-1.64665139190834));
#35168=CARTESIAN_POINT('Ctrl Pts',(-0.985642622921626,-1.,-1.6511001661277));
#35169=CARTESIAN_POINT('Ctrl Pts',(-0.985642622921626,1.,-1.6511001661277));
#35170=CARTESIAN_POINT('Ctrl Pts',(-0.98985562785445,-1.,-1.65559044289746));
#35171=CARTESIAN_POINT('Ctrl Pts',(-0.98985562785445,1.,-1.65559044289746));
#35172=CARTESIAN_POINT('Ctrl Pts',(-0.994121836661116,-1.,-1.66001553809916));
#35173=CARTESIAN_POINT('Ctrl Pts',(-0.994121836661116,1.,-1.66001553809916));
#35174=CARTESIAN_POINT('Ctrl Pts',(-0.998389654952317,-1.,-1.66430758030304));
#35175=CARTESIAN_POINT('Ctrl Pts',(-0.998389654952317,1.,-1.66430758030304));
#35176=CARTESIAN_POINT('Ctrl Pts',(-1.00265091003682,-1.,-1.66846059277231));
#35177=CARTESIAN_POINT('Ctrl Pts',(-1.00265091003682,1.,-1.66846059277231));
#35178=CARTESIAN_POINT('Ctrl Pts',(-1.00692206696387,-1.,-1.67250335383248));
#35179=CARTESIAN_POINT('Ctrl Pts',(-1.00692206696387,1.,-1.67250335383248));
#35180=CARTESIAN_POINT('Ctrl Pts',(-1.01123236493507,-1.,-1.67648246776457));
#35181=CARTESIAN_POINT('Ctrl Pts',(-1.01123236493507,1.,-1.67648246776457));
#35182=CARTESIAN_POINT('Ctrl Pts',(-1.01561026162787,-1.,-1.6804428989482));
#35183=CARTESIAN_POINT('Ctrl Pts',(-1.01561026162787,1.,-1.6804428989482));
#35184=CARTESIAN_POINT('Ctrl Pts',(-1.02006795074222,-1.,-1.68440578021739));
#35185=CARTESIAN_POINT('Ctrl Pts',(-1.02006795074222,1.,-1.68440578021739));
#35186=CARTESIAN_POINT('Ctrl Pts',(-1.02460180535272,-1.,-1.68836910178475));
#35187=CARTESIAN_POINT('Ctrl Pts',(-1.02460180535272,1.,-1.68836910178475));
#35188=CARTESIAN_POINT('Ctrl Pts',(-1.02919977579155,-1.,-1.69231840863471));
#35189=CARTESIAN_POINT('Ctrl Pts',(-1.02919977579155,1.,-1.69231840863471));
#35190=CARTESIAN_POINT('Ctrl Pts',(-1.03384646003587,-1.,-1.69623414782769));
#35191=CARTESIAN_POINT('Ctrl Pts',(-1.03384646003587,1.,-1.69623414782769));
#35192=CARTESIAN_POINT('Ctrl Pts',(-1.03852922490782,-1.,-1.70010052930951));
#35193=CARTESIAN_POINT('Ctrl Pts',(-1.03852922490782,1.,-1.70010052930951));
#35194=CARTESIAN_POINT('Ctrl Pts',(-1.04324363334546,-1.,-1.70391338707969));
#35195=CARTESIAN_POINT('Ctrl Pts',(-1.04324363334546,1.,-1.70391338707969));
#35196=CARTESIAN_POINT('Ctrl Pts',(-1.0479908540499,-1.,-1.70767646263641));
#35197=CARTESIAN_POINT('Ctrl Pts',(-1.0479908540499,1.,-1.70767646263641));
#35198=CARTESIAN_POINT('Ctrl Pts',(-1.05277517202854,-1.,-1.71139783543986));
#35199=CARTESIAN_POINT('Ctrl Pts',(-1.05277517202854,1.,-1.71139783543986));
#35200=CARTESIAN_POINT('Ctrl Pts',(-1.05760163192481,-1.,-1.71508654427022));
#35201=CARTESIAN_POINT('Ctrl Pts',(-1.05760163192481,1.,-1.71508654427022));
#35202=CARTESIAN_POINT('Ctrl Pts',(-1.0624732468065,-1.,-1.71874858456908));
#35203=CARTESIAN_POINT('Ctrl Pts',(-1.0624732468065,1.,-1.71874858456908));
#35204=CARTESIAN_POINT('Ctrl Pts',(-1.06738966975463,-1.,-1.72238500928456));
#35205=CARTESIAN_POINT('Ctrl Pts',(-1.06738966975463,1.,-1.72238500928456));
#35206=CARTESIAN_POINT('Ctrl Pts',(-1.07234866990252,-1.,-1.72599406198489));
#35207=CARTESIAN_POINT('Ctrl Pts',(-1.07234866990252,1.,-1.72599406198489));
#35208=CARTESIAN_POINT('Ctrl Pts',(-1.0773470373727,-1.,-1.72957248977424));
#35209=CARTESIAN_POINT('Ctrl Pts',(-1.0773470373727,1.,-1.72957248977424));
#35210=CARTESIAN_POINT('Ctrl Pts',(-1.08238162784749,-1.,-1.73311705663407));
#35211=CARTESIAN_POINT('Ctrl Pts',(-1.08238162784749,1.,-1.73311705663407));
#35212=CARTESIAN_POINT('Ctrl Pts',(-1.08745056285429,-1.,-1.73662628326093));
#35213=CARTESIAN_POINT('Ctrl Pts',(-1.08745056285429,1.,-1.73662628326093));
#35214=CARTESIAN_POINT('Ctrl Pts',(-1.09255329056496,-1.,-1.74010053962252));
#35215=CARTESIAN_POINT('Ctrl Pts',(-1.09255329056496,1.,-1.74010053962252));
#35216=CARTESIAN_POINT('Ctrl Pts',(-1.09768999241229,-1.,-1.74354119236212));
#35217=CARTESIAN_POINT('Ctrl Pts',(-1.09768999241229,1.,-1.74354119236212));
#35218=CARTESIAN_POINT('Ctrl Pts',(-1.10286118991144,-1.,-1.74695004214924));
#35219=CARTESIAN_POINT('Ctrl Pts',(-1.10286118991144,1.,-1.74695004214924));
#35220=CARTESIAN_POINT('Ctrl Pts',(-1.10806728183003,-1.,-1.75032866075914));
#35221=CARTESIAN_POINT('Ctrl Pts',(-1.10806728183003,1.,-1.75032866075914));
#35222=CARTESIAN_POINT('Ctrl Pts',(-1.11330807582542,-1.,-1.75367772094617));
#35223=CARTESIAN_POINT('Ctrl Pts',(-1.11330807582542,1.,-1.75367772094617));
#35224=CARTESIAN_POINT('Ctrl Pts',(-1.11858293216752,-1.,-1.75699720772089));
#35225=CARTESIAN_POINT('Ctrl Pts',(-1.11858293216752,1.,-1.75699720772089));
#35226=CARTESIAN_POINT('Ctrl Pts',(-1.12389096855078,-1.,-1.76028671825084));
#35227=CARTESIAN_POINT('Ctrl Pts',(-1.12389096855078,1.,-1.76028671825084));
#35228=CARTESIAN_POINT('Ctrl Pts',(-1.12923123555076,-1.,-1.76354571966171));
#35229=CARTESIAN_POINT('Ctrl Pts',(-1.12923123555076,1.,-1.76354571966171));
#35230=CARTESIAN_POINT('Ctrl Pts',(-1.13460291804635,-1.,-1.76677384551883));
#35231=CARTESIAN_POINT('Ctrl Pts',(-1.13460291804635,1.,-1.76677384551883));
#35232=CARTESIAN_POINT('Ctrl Pts',(-1.14000548337,-1.,-1.76997111386806));
#35233=CARTESIAN_POINT('Ctrl Pts',(-1.14000548337,1.,-1.76997111386806));
#35234=CARTESIAN_POINT('Ctrl Pts',(-1.14543858226948,-1.,-1.77313777896234));
#35235=CARTESIAN_POINT('Ctrl Pts',(-1.14543858226948,1.,-1.77313777896234));
#35236=CARTESIAN_POINT('Ctrl Pts',(-1.15090197841531,-1.,-1.77627422557034));
#35237=CARTESIAN_POINT('Ctrl Pts',(-1.15090197841531,1.,-1.77627422557034));
#35238=CARTESIAN_POINT('Ctrl Pts',(-1.15639547194689,-1.,-1.77938085564261));
#35239=CARTESIAN_POINT('Ctrl Pts',(-1.15639547194689,1.,-1.77938085564261));
#35240=CARTESIAN_POINT('Ctrl Pts',(-1.16191881298458,-1.,-1.78245795880949));
#35241=CARTESIAN_POINT('Ctrl Pts',(-1.16191881298458,1.,-1.78245795880949));
#35242=CARTESIAN_POINT('Ctrl Pts',(-1.16747166312239,-1.,-1.78550566040349));
#35243=CARTESIAN_POINT('Ctrl Pts',(-1.16747166312239,1.,-1.78550566040349));
#35244=CARTESIAN_POINT('Ctrl Pts',(-1.17305363177265,-1.,-1.78852398877523));
#35245=CARTESIAN_POINT('Ctrl Pts',(-1.17305363177265,1.,-1.78852398877523));
#35246=CARTESIAN_POINT('Ctrl Pts',(-1.17866429440781,-1.,-1.79151291552646));
#35247=CARTESIAN_POINT('Ctrl Pts',(-1.17866429440781,1.,-1.79151291552646));
#35248=CARTESIAN_POINT('Ctrl Pts',(-1.18430321697471,-1.,-1.79447240321572));
#35249=CARTESIAN_POINT('Ctrl Pts',(-1.18430321697471,1.,-1.79447240321572));
#35250=CARTESIAN_POINT('Ctrl Pts',(-1.1899699793456,-1.,-1.79740245923649));
#35251=CARTESIAN_POINT('Ctrl Pts',(-1.1899699793456,1.,-1.79740245923649));
#35252=CARTESIAN_POINT('Ctrl Pts',(-1.19566418930405,-1.,-1.80030314370121));
#35253=CARTESIAN_POINT('Ctrl Pts',(-1.19566418930405,1.,-1.80030314370121));
#35254=CARTESIAN_POINT('Ctrl Pts',(-1.2013854893912,-1.,-1.8031745483882));
#35255=CARTESIAN_POINT('Ctrl Pts',(-1.2013854893912,1.,-1.8031745483882));
#35256=CARTESIAN_POINT('Ctrl Pts',(-1.20713356605519,-1.,-1.80601678480772));
#35257=CARTESIAN_POINT('Ctrl Pts',(-1.20713356605519,1.,-1.80601678480772));
#35258=CARTESIAN_POINT('Ctrl Pts',(-1.2129081570818,-1.,-1.80882996916931));
#35259=CARTESIAN_POINT('Ctrl Pts',(-1.2129081570818,1.,-1.80882996916931));
#35260=CARTESIAN_POINT('Ctrl Pts',(-1.2187090610323,-1.,-1.81161420806172));
#35261=CARTESIAN_POINT('Ctrl Pts',(-1.2187090610323,1.,-1.81161420806172));
#35262=CARTESIAN_POINT('Ctrl Pts',(-1.22453613304507,-1.,-1.81436959209778));
#35263=CARTESIAN_POINT('Ctrl Pts',(-1.22453613304507,1.,-1.81436959209778));
#35264=CARTESIAN_POINT('Ctrl Pts',(-1.22921864890975,-1.,-1.81655087183054));
#35265=CARTESIAN_POINT('Ctrl Pts',(-1.22921864890975,1.,-1.81655087183054));
#35266=CARTESIAN_POINT('Ctrl Pts',(-1.23274224526804,-1.,-1.81817389920914));
#35267=CARTESIAN_POINT('Ctrl Pts',(-1.23274224526804,1.,-1.81817389920914));
#35268=CARTESIAN_POINT('Ctrl Pts',(-1.23509651170384,-1.,-1.81925017193531));
#35269=CARTESIAN_POINT('Ctrl Pts',(-1.23509651170384,1.,-1.81925017193531));
#35270=CARTESIAN_POINT('Ctrl Pts',(-1.23627494547115,-1.,-1.81978687191668));
#35271=CARTESIAN_POINT('Ctrl Pts',(-1.23627494547115,1.,-1.81978687191668));
#35272=CARTESIAN_POINT('',(-0.892032620296855,1.,-1.5055822144029));
#35273=CARTESIAN_POINT('Ctrl Pts',(-0.892032620296855,1.,-1.5055822144029));
#35274=CARTESIAN_POINT('Ctrl Pts',(-0.894452006967538,1.,-1.50980486807181));
#35275=CARTESIAN_POINT('Ctrl Pts',(-0.89918504749193,1.,-1.51805569591479));
#35276=CARTESIAN_POINT('Ctrl Pts',(-0.905967409640499,1.,-1.52984849890434));
#35277=CARTESIAN_POINT('Ctrl Pts',(-0.91437591904658,1.,-1.54440491152808));
#35278=CARTESIAN_POINT('Ctrl Pts',(-0.923832188966322,1.,-1.56065988582509));
#35279=CARTESIAN_POINT('Ctrl Pts',(-0.932246680128849,1.,-1.57499388385561));
#35280=CARTESIAN_POINT('Ctrl Pts',(-0.939646377909319,1.,-1.58744937489796));
#35281=CARTESIAN_POINT('Ctrl Pts',(-0.946078063325796,1.,-1.59810042045408));
#35282=CARTESIAN_POINT('Ctrl Pts',(-0.951613284361248,1.,-1.60706069897794));
#35283=CARTESIAN_POINT('Ctrl Pts',(-0.956354422921573,1.,-1.61449324337233));
#35284=CARTESIAN_POINT('Ctrl Pts',(-0.960438326099958,1.,-1.62061638139929));
#35285=CARTESIAN_POINT('Ctrl Pts',(-0.964046107037821,1.,-1.6257193066974));
#35286=CARTESIAN_POINT('Ctrl Pts',(-0.967387853228041,1.,-1.63013849959083));
#35287=CARTESIAN_POINT('Ctrl Pts',(-0.970669715996356,1.,-1.63420665729609));
#35288=CARTESIAN_POINT('Ctrl Pts',(-0.974066058287501,1.,-1.63820952658157));
#35289=CARTESIAN_POINT('Ctrl Pts',(-0.977689794120297,1.,-1.64233990826831));
#35290=CARTESIAN_POINT('Ctrl Pts',(-0.981562530940574,1.,-1.64665139190834));
#35291=CARTESIAN_POINT('Ctrl Pts',(-0.985642622921626,1.,-1.6511001661277));
#35292=CARTESIAN_POINT('Ctrl Pts',(-0.98985562785445,1.,-1.65559044289746));
#35293=CARTESIAN_POINT('Ctrl Pts',(-0.994121836661116,1.,-1.66001553809916));
#35294=CARTESIAN_POINT('Ctrl Pts',(-0.998389654952317,1.,-1.66430758030304));
#35295=CARTESIAN_POINT('Ctrl Pts',(-1.00265091003682,1.,-1.66846059277231));
#35296=CARTESIAN_POINT('Ctrl Pts',(-1.00692206696387,1.,-1.67250335383248));
#35297=CARTESIAN_POINT('Ctrl Pts',(-1.01123236493507,1.,-1.67648246776457));
#35298=CARTESIAN_POINT('Ctrl Pts',(-1.01561026162787,1.,-1.6804428989482));
#35299=CARTESIAN_POINT('Ctrl Pts',(-1.02006795074222,1.,-1.68440578021739));
#35300=CARTESIAN_POINT('Ctrl Pts',(-1.02460180535272,1.,-1.68836910178475));
#35301=CARTESIAN_POINT('Ctrl Pts',(-1.02919977579155,1.,-1.69231840863471));
#35302=CARTESIAN_POINT('Ctrl Pts',(-1.03384646003587,1.,-1.69623414782769));
#35303=CARTESIAN_POINT('Ctrl Pts',(-1.03852922490782,1.,-1.70010052930951));
#35304=CARTESIAN_POINT('Ctrl Pts',(-1.04324363334546,1.,-1.70391338707969));
#35305=CARTESIAN_POINT('Ctrl Pts',(-1.0479908540499,1.,-1.70767646263641));
#35306=CARTESIAN_POINT('Ctrl Pts',(-1.05277517202854,1.,-1.71139783543986));
#35307=CARTESIAN_POINT('Ctrl Pts',(-1.05760163192481,1.,-1.71508654427022));
#35308=CARTESIAN_POINT('Ctrl Pts',(-1.0624732468065,1.,-1.71874858456908));
#35309=CARTESIAN_POINT('Ctrl Pts',(-1.06738966975463,1.,-1.72238500928456));
#35310=CARTESIAN_POINT('Ctrl Pts',(-1.07234866990252,1.,-1.72599406198489));
#35311=CARTESIAN_POINT('Ctrl Pts',(-1.0773470373727,1.,-1.72957248977424));
#35312=CARTESIAN_POINT('Ctrl Pts',(-1.08238162784749,1.,-1.73311705663407));
#35313=CARTESIAN_POINT('Ctrl Pts',(-1.08745056285429,1.,-1.73662628326093));
#35314=CARTESIAN_POINT('Ctrl Pts',(-1.09255329056496,1.,-1.74010053962252));
#35315=CARTESIAN_POINT('Ctrl Pts',(-1.09768999241229,1.,-1.74354119236212));
#35316=CARTESIAN_POINT('Ctrl Pts',(-1.10286118991144,1.,-1.74695004214924));
#35317=CARTESIAN_POINT('Ctrl Pts',(-1.10806728183003,1.,-1.75032866075914));
#35318=CARTESIAN_POINT('Ctrl Pts',(-1.11330807582542,1.,-1.75367772094617));
#35319=CARTESIAN_POINT('Ctrl Pts',(-1.11858293216752,1.,-1.75699720772089));
#35320=CARTESIAN_POINT('Ctrl Pts',(-1.12389096855078,1.,-1.76028671825084));
#35321=CARTESIAN_POINT('Ctrl Pts',(-1.12923123555076,1.,-1.76354571966171));
#35322=CARTESIAN_POINT('Ctrl Pts',(-1.13460291804635,1.,-1.76677384551883));
#35323=CARTESIAN_POINT('Ctrl Pts',(-1.14000548337,1.,-1.76997111386806));
#35324=CARTESIAN_POINT('Ctrl Pts',(-1.14543858226948,1.,-1.77313777896234));
#35325=CARTESIAN_POINT('Ctrl Pts',(-1.15090197841531,1.,-1.77627422557034));
#35326=CARTESIAN_POINT('Ctrl Pts',(-1.15639547194689,1.,-1.77938085564261));
#35327=CARTESIAN_POINT('Ctrl Pts',(-1.16191881298458,1.,-1.78245795880949));
#35328=CARTESIAN_POINT('Ctrl Pts',(-1.16747166312239,1.,-1.78550566040349));
#35329=CARTESIAN_POINT('Ctrl Pts',(-1.17305363177265,1.,-1.78852398877523));
#35330=CARTESIAN_POINT('Ctrl Pts',(-1.17866429440781,1.,-1.79151291552646));
#35331=CARTESIAN_POINT('Ctrl Pts',(-1.18430321697471,1.,-1.79447240321572));
#35332=CARTESIAN_POINT('Ctrl Pts',(-1.1899699793456,1.,-1.79740245923649));
#35333=CARTESIAN_POINT('Ctrl Pts',(-1.19566418930405,1.,-1.80030314370121));
#35334=CARTESIAN_POINT('Ctrl Pts',(-1.2013854893912,1.,-1.8031745483882));
#35335=CARTESIAN_POINT('Ctrl Pts',(-1.20713356605519,1.,-1.80601678480772));
#35336=CARTESIAN_POINT('Ctrl Pts',(-1.2129081570818,1.,-1.80882996916931));
#35337=CARTESIAN_POINT('Ctrl Pts',(-1.2187090610323,1.,-1.81161420806172));
#35338=CARTESIAN_POINT('Ctrl Pts',(-1.22453613304507,1.,-1.81436959209778));
#35339=CARTESIAN_POINT('Ctrl Pts',(-1.22921864890975,1.,-1.81655087183054));
#35340=CARTESIAN_POINT('Ctrl Pts',(-1.23274224526804,1.,-1.81817389920914));
#35341=CARTESIAN_POINT('Ctrl Pts',(-1.23509651170384,1.,-1.81925017193531));
#35342=CARTESIAN_POINT('Ctrl Pts',(-1.23627494547115,1.,-1.81978687191668));
#35343=CARTESIAN_POINT('',(-0.892032620296856,0.,-1.5055822144029));
#35344=CARTESIAN_POINT('Origin',(0.,0.,0.));
#35345=CARTESIAN_POINT('',(-0.693717979106305,1.,-1.60662857109684));
#35346=CARTESIAN_POINT('Origin',(0.,1.,0.));
#35347=CARTESIAN_POINT('',(-0.693717979106306,0.,-1.60662857109684));
#35348=CARTESIAN_POINT('Ctrl Pts',(-0.745574324794401,-1.,-2.0698113262342));
#35349=CARTESIAN_POINT('Ctrl Pts',(-0.745574324794401,1.,-2.0698113262342));
#35350=CARTESIAN_POINT('Ctrl Pts',(-0.745832791378367,-1.,-2.06854248895728));
#35351=CARTESIAN_POINT('Ctrl Pts',(-0.745832791378367,1.,-2.06854248895728));
#35352=CARTESIAN_POINT('Ctrl Pts',(-0.7463458715442,-1.,-2.06600523016815));
#35353=CARTESIAN_POINT('Ctrl Pts',(-0.7463458715442,1.,-2.06600523016815));
#35354=CARTESIAN_POINT('Ctrl Pts',(-0.747103932787919,-1.,-2.06220058927826));
#35355=CARTESIAN_POINT('Ctrl Pts',(-0.747103932787919,1.,-2.06220058927826));
#35356=CARTESIAN_POINT('Ctrl Pts',(-0.748091554183802,-1.,-2.05713023031006));
#35357=CARTESIAN_POINT('Ctrl Pts',(-0.748091554183802,1.,-2.05713023031006));
#35358=CARTESIAN_POINT('Ctrl Pts',(-0.749287468665046,-1.,-2.05079645592154));
#35359=CARTESIAN_POINT('Ctrl Pts',(-0.749287468665046,1.,-2.05079645592154));
#35360=CARTESIAN_POINT('Ctrl Pts',(-0.750444657875576,-1.,-2.04446689147979));
#35361=CARTESIAN_POINT('Ctrl Pts',(-0.750444657875576,1.,-2.04446689147979));
#35362=CARTESIAN_POINT('Ctrl Pts',(-0.751562963361115,-1.,-2.03814160092099));
#35363=CARTESIAN_POINT('Ctrl Pts',(-0.751562963361115,1.,-2.03814160092099));
#35364=CARTESIAN_POINT('Ctrl Pts',(-0.752642180487211,-1.,-2.03182068456221));
#35365=CARTESIAN_POINT('Ctrl Pts',(-0.752642180487211,1.,-2.03182068456221));
#35366=CARTESIAN_POINT('Ctrl Pts',(-0.753682061112768,-1.,-2.02550428623313));
#35367=CARTESIAN_POINT('Ctrl Pts',(-0.753682061112768,1.,-2.02550428623313));
#35368=CARTESIAN_POINT('Ctrl Pts',(-0.754682330722816,-1.,-2.01919259405809));
#35369=CARTESIAN_POINT('Ctrl Pts',(-0.754682330722816,1.,-2.01919259405809));
#35370=CARTESIAN_POINT('Ctrl Pts',(-0.755642704957865,-1.,-2.01288584328084));
#35371=CARTESIAN_POINT('Ctrl Pts',(-0.755642704957865,1.,-2.01288584328084));
#35372=CARTESIAN_POINT('Ctrl Pts',(-0.75656290464667,-1.,-2.0065843158773));
#35373=CARTESIAN_POINT('Ctrl Pts',(-0.75656290464667,1.,-2.0065843158773));
#35374=CARTESIAN_POINT('Ctrl Pts',(-0.757442676862724,-1.,-2.00028834739178));
#35375=CARTESIAN_POINT('Ctrl Pts',(-0.757442676862724,1.,-2.00028834739178));
#35376=CARTESIAN_POINT('Ctrl Pts',(-0.758281796766761,-1.,-1.99399831098817));
#35377=CARTESIAN_POINT('Ctrl Pts',(-0.758281796766761,1.,-1.99399831098817));
#35378=CARTESIAN_POINT('Ctrl Pts',(-0.759080037802488,-1.,-1.98771456680874));
#35379=CARTESIAN_POINT('Ctrl Pts',(-0.759080037802488,1.,-1.98771456680874));
#35380=CARTESIAN_POINT('Ctrl Pts',(-0.75983714745219,-1.,-1.98143741418172));
#35381=CARTESIAN_POINT('Ctrl Pts',(-0.75983714745219,1.,-1.98143741418172));
#35382=CARTESIAN_POINT('Ctrl Pts',(-0.760552825409757,-1.,-1.97516705321494));
#35383=CARTESIAN_POINT('Ctrl Pts',(-0.760552825409757,1.,-1.97516705321494));
#35384=CARTESIAN_POINT('Ctrl Pts',(-0.76122669048382,-1.,-1.96890351582499));
#35385=CARTESIAN_POINT('Ctrl Pts',(-0.76122669048382,1.,-1.96890351582499));
#35386=CARTESIAN_POINT('Ctrl Pts',(-0.761858300014423,-1.,-1.96264672744186));
#35387=CARTESIAN_POINT('Ctrl Pts',(-0.761858300014423,1.,-1.96264672744186));
#35388=CARTESIAN_POINT('Ctrl Pts',(-0.762447203806179,-1.,-1.95639665309869));
#35389=CARTESIAN_POINT('Ctrl Pts',(-0.762447203806179,1.,-1.95639665309869));
#35390=CARTESIAN_POINT('Ctrl Pts',(-0.762992990878769,-1.,-1.95015342590024));
#35391=CARTESIAN_POINT('Ctrl Pts',(-0.762992990878769,1.,-1.95015342590024));
#35392=CARTESIAN_POINT('Ctrl Pts',(-0.763495333538629,-1.,-1.9439174661764));
#35393=CARTESIAN_POINT('Ctrl Pts',(-0.763495333538629,1.,-1.9439174661764));
#35394=CARTESIAN_POINT('Ctrl Pts',(-0.763954049121458,-1.,-1.93768964875886));
#35395=CARTESIAN_POINT('Ctrl Pts',(-0.763954049121458,1.,-1.93768964875886));
#35396=CARTESIAN_POINT('Ctrl Pts',(-0.764369010673941,-1.,-1.93147105496382));
#35397=CARTESIAN_POINT('Ctrl Pts',(-0.764369010673941,1.,-1.93147105496382));
#35398=CARTESIAN_POINT('Ctrl Pts',(-0.764740025488211,-1.,-1.92526263537048));
#35399=CARTESIAN_POINT('Ctrl Pts',(-0.764740025488211,1.,-1.92526263537048));
#35400=CARTESIAN_POINT('Ctrl Pts',(-0.765066729667088,-1.,-1.91906491634196));
#35401=CARTESIAN_POINT('Ctrl Pts',(-0.765066729667088,1.,-1.91906491634196));
#35402=CARTESIAN_POINT('Ctrl Pts',(-0.765348465884722,-1.,-1.91287765805169));
#35403=CARTESIAN_POINT('Ctrl Pts',(-0.765348465884722,1.,-1.91287765805169));
#35404=CARTESIAN_POINT('Ctrl Pts',(-0.765584196937919,-1.,-1.90669961402356));
#35405=CARTESIAN_POINT('Ctrl Pts',(-0.765584196937919,1.,-1.90669961402356));
#35406=CARTESIAN_POINT('Ctrl Pts',(-0.765772772593386,-1.,-1.90052930393596));
#35407=CARTESIAN_POINT('Ctrl Pts',(-0.765772772593386,1.,-1.90052930393596));
#35408=CARTESIAN_POINT('Ctrl Pts',(-0.765913193856978,-1.,-1.89436577771388));
#35409=CARTESIAN_POINT('Ctrl Pts',(-0.765913193856978,1.,-1.89436577771388));
#35410=CARTESIAN_POINT('Ctrl Pts',(-0.766004837062091,-1.,-1.88820926433409));
#35411=CARTESIAN_POINT('Ctrl Pts',(-0.766004837062091,1.,-1.88820926433409));
#35412=CARTESIAN_POINT('Ctrl Pts',(-0.766047794851865,-1.,-1.88206215302561));
#35413=CARTESIAN_POINT('Ctrl Pts',(-0.766047794851865,1.,-1.88206215302561));
#35414=CARTESIAN_POINT('Ctrl Pts',(-0.766042837036744,-1.,-1.87592888967883));
#35415=CARTESIAN_POINT('Ctrl Pts',(-0.766042837036744,1.,-1.87592888967883));
#35416=CARTESIAN_POINT('Ctrl Pts',(-0.765990708546091,-1.,-1.86981398314341));
#35417=CARTESIAN_POINT('Ctrl Pts',(-0.765990708546091,1.,-1.86981398314341));
#35418=CARTESIAN_POINT('Ctrl Pts',(-0.765891519092547,-1.,-1.86372027063312));
#35419=CARTESIAN_POINT('Ctrl Pts',(-0.765891519092547,1.,-1.86372027063312));
#35420=CARTESIAN_POINT('Ctrl Pts',(-0.765744212909318,-1.,-1.85764741390394));
#35421=CARTESIAN_POINT('Ctrl Pts',(-0.765744212909318,1.,-1.85764741390394));
#35422=CARTESIAN_POINT('Ctrl Pts',(-0.765545710619062,-1.,-1.85158945130063));
#35423=CARTESIAN_POINT('Ctrl Pts',(-0.765545710619062,1.,-1.85158945130063));
#35424=CARTESIAN_POINT('Ctrl Pts',(-0.765291664862029,-1.,-1.84553698875924));
#35425=CARTESIAN_POINT('Ctrl Pts',(-0.765291664862029,1.,-1.84553698875924));
#35426=CARTESIAN_POINT('Ctrl Pts',(-0.764978057881737,-1.,-1.83948181064835));
#35427=CARTESIAN_POINT('Ctrl Pts',(-0.764978057881737,1.,-1.83948181064835));
#35428=CARTESIAN_POINT('Ctrl Pts',(-0.764602549687853,-1.,-1.83342077227142));
#35429=CARTESIAN_POINT('Ctrl Pts',(-0.764602549687853,1.,-1.83342077227142));
#35430=CARTESIAN_POINT('Ctrl Pts',(-0.764165902605995,-1.,-1.82735991200065));
#35431=CARTESIAN_POINT('Ctrl Pts',(-0.764165902605995,1.,-1.82735991200065));
#35432=CARTESIAN_POINT('Ctrl Pts',(-0.763673465462726,-1.,-1.82131873145266));
#35433=CARTESIAN_POINT('Ctrl Pts',(-0.763673465462726,1.,-1.82131873145266));
#35434=CARTESIAN_POINT('Ctrl Pts',(-0.763132003836634,-1.,-1.8153211840553));
#35435=CARTESIAN_POINT('Ctrl Pts',(-0.763132003836634,1.,-1.8153211840553));
#35436=CARTESIAN_POINT('Ctrl Pts',(-0.762546129463938,-1.,-1.80938551463965));
#35437=CARTESIAN_POINT('Ctrl Pts',(-0.762546129463938,1.,-1.80938551463965));
#35438=CARTESIAN_POINT('Ctrl Pts',(-0.761915336443547,-1.,-1.80351583877342));
#35439=CARTESIAN_POINT('Ctrl Pts',(-0.761915336443547,1.,-1.80351583877342));
#35440=CARTESIAN_POINT('Ctrl Pts',(-0.761229695230558,-1.,-1.79768986997783));
#35441=CARTESIAN_POINT('Ctrl Pts',(-0.761229695230558,1.,-1.79768986997783));
#35442=CARTESIAN_POINT('Ctrl Pts',(-0.760469555880749,-1.,-1.7918581561088));
#35443=CARTESIAN_POINT('Ctrl Pts',(-0.760469555880749,1.,-1.7918581561088));
#35444=CARTESIAN_POINT('Ctrl Pts',(-0.759614401110189,-1.,-1.78596964884604));
#35445=CARTESIAN_POINT('Ctrl Pts',(-0.759614401110189,1.,-1.78596964884604));
#35446=CARTESIAN_POINT('Ctrl Pts',(-0.758650626677518,-1.,-1.77999411220945));
#35447=CARTESIAN_POINT('Ctrl Pts',(-0.758650626677518,1.,-1.77999411220945));
#35448=CARTESIAN_POINT('Ctrl Pts',(-0.757578264077029,-1.,-1.77394167108292));
#35449=CARTESIAN_POINT('Ctrl Pts',(-0.757578264077029,1.,-1.77394167108292));
#35450=CARTESIAN_POINT('Ctrl Pts',(-0.75642189602781,-1.,-1.76789396002998));
#35451=CARTESIAN_POINT('Ctrl Pts',(-0.75642189602781,1.,-1.76789396002998));
#35452=CARTESIAN_POINT('Ctrl Pts',(-0.755220979974461,-1.,-1.76197817240128));
#35453=CARTESIAN_POINT('Ctrl Pts',(-0.755220979974461,1.,-1.76197817240128));
#35454=CARTESIAN_POINT('Ctrl Pts',(-0.754009254027829,-1.,-1.75631083600019));
#35455=CARTESIAN_POINT('Ctrl Pts',(-0.754009254027829,1.,-1.75631083600019));
#35456=CARTESIAN_POINT('Ctrl Pts',(-0.752797683531314,-1.,-1.75095139468794));
#35457=CARTESIAN_POINT('Ctrl Pts',(-0.752797683531314,1.,-1.75095139468794));
#35458=CARTESIAN_POINT('Ctrl Pts',(-0.751555614164482,-1.,-1.74585086852502));
#35459=CARTESIAN_POINT('Ctrl Pts',(-0.751555614164482,1.,-1.74585086852502));
#35460=CARTESIAN_POINT('Ctrl Pts',(-0.750193435981249,-1.,-1.74080458267114));
#35461=CARTESIAN_POINT('Ctrl Pts',(-0.750193435981249,1.,-1.74080458267114));
#35462=CARTESIAN_POINT('Ctrl Pts',(-0.74858246295687,-1.,-1.7355035168033));
#35463=CARTESIAN_POINT('Ctrl Pts',(-0.74858246295687,1.,-1.7355035168033));
#35464=CARTESIAN_POINT('Ctrl Pts',(-0.746574710097752,-1.,-1.72958533647714));
#35465=CARTESIAN_POINT('Ctrl Pts',(-0.746574710097752,1.,-1.72958533647714));
#35466=CARTESIAN_POINT('Ctrl Pts',(-0.744021445433093,-1.,-1.72268229916769));
#35467=CARTESIAN_POINT('Ctrl Pts',(-0.744021445433093,1.,-1.72268229916769));
#35468=CARTESIAN_POINT('Ctrl Pts',(-0.74079516202821,-1.,-1.71447789751001));
#35469=CARTESIAN_POINT('Ctrl Pts',(-0.74079516202821,1.,-1.71447789751001));
#35470=CARTESIAN_POINT('Ctrl Pts',(-0.736799665716932,-1.,-1.70473309004249));
#35471=CARTESIAN_POINT('Ctrl Pts',(-0.736799665716932,1.,-1.70473309004249));
#35472=CARTESIAN_POINT('Ctrl Pts',(-0.731963238685357,-1.,-1.69326921972915));
#35473=CARTESIAN_POINT('Ctrl Pts',(-0.731963238685357,1.,-1.69326921972915));
#35474=CARTESIAN_POINT('Ctrl Pts',(-0.726235967982445,-1.,-1.67996158451922));
#35475=CARTESIAN_POINT('Ctrl Pts',(-0.726235967982445,1.,-1.67996158451922));
#35476=CARTESIAN_POINT('Ctrl Pts',(-0.71958543378795,-1.,-1.66472880551777));
#35477=CARTESIAN_POINT('Ctrl Pts',(-0.71958543378795,1.,-1.66472880551777));
#35478=CARTESIAN_POINT('Ctrl Pts',(-0.711993139340447,-1.,-1.64752408828442));
#35479=CARTESIAN_POINT('Ctrl Pts',(-0.711993139340447,1.,-1.64752408828442));
#35480=CARTESIAN_POINT('Ctrl Pts',(-0.705159151977294,-1.,-1.6321654166204));
#35481=CARTESIAN_POINT('Ctrl Pts',(-0.705159151977294,1.,-1.6321654166204));
#35482=CARTESIAN_POINT('Ctrl Pts',(-0.699605146398837,-1.,-1.61974673471117));
#35483=CARTESIAN_POINT('Ctrl Pts',(-0.699605146398837,1.,-1.61974673471117));
#35484=CARTESIAN_POINT('Ctrl Pts',(-0.69571209787897,-1.,-1.61106790957619));
#35485=CARTESIAN_POINT('Ctrl Pts',(-0.69571209787897,1.,-1.61106790957619));
#35486=CARTESIAN_POINT('Ctrl Pts',(-0.693717979106305,-1.,-1.60662857109684));
#35487=CARTESIAN_POINT('Ctrl Pts',(-0.693717979106305,1.,-1.60662857109684));
#35488=CARTESIAN_POINT('',(-0.745574324794401,1.,-2.0698113262342));
#35489=CARTESIAN_POINT('Ctrl Pts',(-0.745574324794401,1.,-2.0698113262342));
#35490=CARTESIAN_POINT('Ctrl Pts',(-0.745832791378367,1.,-2.06854248895728));
#35491=CARTESIAN_POINT('Ctrl Pts',(-0.7463458715442,1.,-2.06600523016815));
#35492=CARTESIAN_POINT('Ctrl Pts',(-0.747103932787919,1.,-2.06220058927826));
#35493=CARTESIAN_POINT('Ctrl Pts',(-0.748091554183802,1.,-2.05713023031006));
#35494=CARTESIAN_POINT('Ctrl Pts',(-0.749287468665046,1.,-2.05079645592154));
#35495=CARTESIAN_POINT('Ctrl Pts',(-0.750444657875576,1.,-2.04446689147979));
#35496=CARTESIAN_POINT('Ctrl Pts',(-0.751562963361115,1.,-2.03814160092099));
#35497=CARTESIAN_POINT('Ctrl Pts',(-0.752642180487211,1.,-2.03182068456221));
#35498=CARTESIAN_POINT('Ctrl Pts',(-0.753682061112768,1.,-2.02550428623313));
#35499=CARTESIAN_POINT('Ctrl Pts',(-0.754682330722816,1.,-2.01919259405809));
#35500=CARTESIAN_POINT('Ctrl Pts',(-0.755642704957865,1.,-2.01288584328084));
#35501=CARTESIAN_POINT('Ctrl Pts',(-0.75656290464667,1.,-2.0065843158773));
#35502=CARTESIAN_POINT('Ctrl Pts',(-0.757442676862724,1.,-2.00028834739178));
#35503=CARTESIAN_POINT('Ctrl Pts',(-0.758281796766761,1.,-1.99399831098817));
#35504=CARTESIAN_POINT('Ctrl Pts',(-0.759080037802488,1.,-1.98771456680874));
#35505=CARTESIAN_POINT('Ctrl Pts',(-0.75983714745219,1.,-1.98143741418172));
#35506=CARTESIAN_POINT('Ctrl Pts',(-0.760552825409757,1.,-1.97516705321494));
#35507=CARTESIAN_POINT('Ctrl Pts',(-0.76122669048382,1.,-1.96890351582499));
#35508=CARTESIAN_POINT('Ctrl Pts',(-0.761858300014423,1.,-1.96264672744186));
#35509=CARTESIAN_POINT('Ctrl Pts',(-0.762447203806179,1.,-1.95639665309869));
#35510=CARTESIAN_POINT('Ctrl Pts',(-0.762992990878769,1.,-1.95015342590024));
#35511=CARTESIAN_POINT('Ctrl Pts',(-0.763495333538629,1.,-1.9439174661764));
#35512=CARTESIAN_POINT('Ctrl Pts',(-0.763954049121458,1.,-1.93768964875886));
#35513=CARTESIAN_POINT('Ctrl Pts',(-0.764369010673941,1.,-1.93147105496382));
#35514=CARTESIAN_POINT('Ctrl Pts',(-0.764740025488211,1.,-1.92526263537048));
#35515=CARTESIAN_POINT('Ctrl Pts',(-0.765066729667088,1.,-1.91906491634196));
#35516=CARTESIAN_POINT('Ctrl Pts',(-0.765348465884722,1.,-1.91287765805169));
#35517=CARTESIAN_POINT('Ctrl Pts',(-0.765584196937919,1.,-1.90669961402356));
#35518=CARTESIAN_POINT('Ctrl Pts',(-0.765772772593386,1.,-1.90052930393596));
#35519=CARTESIAN_POINT('Ctrl Pts',(-0.765913193856978,1.,-1.89436577771388));
#35520=CARTESIAN_POINT('Ctrl Pts',(-0.766004837062091,1.,-1.88820926433409));
#35521=CARTESIAN_POINT('Ctrl Pts',(-0.766047794851865,1.,-1.88206215302561));
#35522=CARTESIAN_POINT('Ctrl Pts',(-0.766042837036744,1.,-1.87592888967883));
#35523=CARTESIAN_POINT('Ctrl Pts',(-0.765990708546091,1.,-1.86981398314341));
#35524=CARTESIAN_POINT('Ctrl Pts',(-0.765891519092547,1.,-1.86372027063312));
#35525=CARTESIAN_POINT('Ctrl Pts',(-0.765744212909318,1.,-1.85764741390394));
#35526=CARTESIAN_POINT('Ctrl Pts',(-0.765545710619062,1.,-1.85158945130063));
#35527=CARTESIAN_POINT('Ctrl Pts',(-0.765291664862029,1.,-1.84553698875924));
#35528=CARTESIAN_POINT('Ctrl Pts',(-0.764978057881737,1.,-1.83948181064835));
#35529=CARTESIAN_POINT('Ctrl Pts',(-0.764602549687853,1.,-1.83342077227142));
#35530=CARTESIAN_POINT('Ctrl Pts',(-0.764165902605995,1.,-1.82735991200065));
#35531=CARTESIAN_POINT('Ctrl Pts',(-0.763673465462726,1.,-1.82131873145266));
#35532=CARTESIAN_POINT('Ctrl Pts',(-0.763132003836634,1.,-1.8153211840553));
#35533=CARTESIAN_POINT('Ctrl Pts',(-0.762546129463938,1.,-1.80938551463965));
#35534=CARTESIAN_POINT('Ctrl Pts',(-0.761915336443547,1.,-1.80351583877342));
#35535=CARTESIAN_POINT('Ctrl Pts',(-0.761229695230558,1.,-1.79768986997783));
#35536=CARTESIAN_POINT('Ctrl Pts',(-0.760469555880749,1.,-1.7918581561088));
#35537=CARTESIAN_POINT('Ctrl Pts',(-0.759614401110189,1.,-1.78596964884604));
#35538=CARTESIAN_POINT('Ctrl Pts',(-0.758650626677518,1.,-1.77999411220945));
#35539=CARTESIAN_POINT('Ctrl Pts',(-0.757578264077029,1.,-1.77394167108292));
#35540=CARTESIAN_POINT('Ctrl Pts',(-0.75642189602781,1.,-1.76789396002998));
#35541=CARTESIAN_POINT('Ctrl Pts',(-0.755220979974461,1.,-1.76197817240128));
#35542=CARTESIAN_POINT('Ctrl Pts',(-0.754009254027829,1.,-1.75631083600019));
#35543=CARTESIAN_POINT('Ctrl Pts',(-0.752797683531314,1.,-1.75095139468794));
#35544=CARTESIAN_POINT('Ctrl Pts',(-0.751555614164482,1.,-1.74585086852502));
#35545=CARTESIAN_POINT('Ctrl Pts',(-0.750193435981249,1.,-1.74080458267114));
#35546=CARTESIAN_POINT('Ctrl Pts',(-0.74858246295687,1.,-1.7355035168033));
#35547=CARTESIAN_POINT('Ctrl Pts',(-0.746574710097752,1.,-1.72958533647714));
#35548=CARTESIAN_POINT('Ctrl Pts',(-0.744021445433093,1.,-1.72268229916769));
#35549=CARTESIAN_POINT('Ctrl Pts',(-0.74079516202821,1.,-1.71447789751001));
#35550=CARTESIAN_POINT('Ctrl Pts',(-0.736799665716932,1.,-1.70473309004249));
#35551=CARTESIAN_POINT('Ctrl Pts',(-0.731963238685357,1.,-1.69326921972915));
#35552=CARTESIAN_POINT('Ctrl Pts',(-0.726235967982445,1.,-1.67996158451922));
#35553=CARTESIAN_POINT('Ctrl Pts',(-0.71958543378795,1.,-1.66472880551777));
#35554=CARTESIAN_POINT('Ctrl Pts',(-0.711993139340447,1.,-1.64752408828442));
#35555=CARTESIAN_POINT('Ctrl Pts',(-0.705159151977294,1.,-1.6321654166204));
#35556=CARTESIAN_POINT('Ctrl Pts',(-0.699605146398837,1.,-1.61974673471117));
#35557=CARTESIAN_POINT('Ctrl Pts',(-0.69571209787897,1.,-1.61106790957619));
#35558=CARTESIAN_POINT('Ctrl Pts',(-0.693717979106305,1.,-1.60662857109684));
#35559=CARTESIAN_POINT('',(-0.745574324794401,0.,-2.0698113262342));
#35560=CARTESIAN_POINT('Origin',(-0.61342227326009,0.,-2.11275013067528));
#35561=CARTESIAN_POINT('',(-0.61342227326009,1.,-2.11275013067528));
#35562=CARTESIAN_POINT('',(-0.745574324794401,1.,-2.0698113262342));
#35563=CARTESIAN_POINT('',(-0.61342227326009,0.,-2.11275013067528));
#35564=CARTESIAN_POINT('Ctrl Pts',(-0.383122945602004,-1.,-1.7075470150345));
#35565=CARTESIAN_POINT('Ctrl Pts',(-0.383122945602004,1.,-1.7075470150345));
#35566=CARTESIAN_POINT('Ctrl Pts',(-0.384119047315542,-1.,-1.71231062891958));
#35567=CARTESIAN_POINT('Ctrl Pts',(-0.384119047315542,1.,-1.71231062891958));
#35568=CARTESIAN_POINT('Ctrl Pts',(-0.38607079032701,-1.,-1.72162022246158));
#35569=CARTESIAN_POINT('Ctrl Pts',(-0.38607079032701,1.,-1.72162022246158));
#35570=CARTESIAN_POINT('Ctrl Pts',(-0.388877023509191,-1.,-1.7349317097561));
#35571=CARTESIAN_POINT('Ctrl Pts',(-0.388877023509191,1.,-1.7349317097561));
#35572=CARTESIAN_POINT('Ctrl Pts',(-0.392375812294307,-1.,-1.75137405313962));
#35573=CARTESIAN_POINT('Ctrl Pts',(-0.392375812294307,1.,-1.75137405313962));
#35574=CARTESIAN_POINT('Ctrl Pts',(-0.39634619612042,-1.,-1.7697556004756));
#35575=CARTESIAN_POINT('Ctrl Pts',(-0.39634619612042,1.,-1.7697556004756));
#35576=CARTESIAN_POINT('Ctrl Pts',(-0.39991940378308,-1.,-1.78598826347533));
#35577=CARTESIAN_POINT('Ctrl Pts',(-0.39991940378308,1.,-1.78598826347533));
#35578=CARTESIAN_POINT('Ctrl Pts',(-0.403107976170441,-1.,-1.80012077176221));
#35579=CARTESIAN_POINT('Ctrl Pts',(-0.403107976170441,1.,-1.80012077176221));
#35580=CARTESIAN_POINT('Ctrl Pts',(-0.405933518411838,-1.,-1.81223801813988));
#35581=CARTESIAN_POINT('Ctrl Pts',(-0.405933518411838,1.,-1.81223801813988));
#35582=CARTESIAN_POINT('Ctrl Pts',(-0.408428948108533,-1.,-1.8224702267854));
#35583=CARTESIAN_POINT('Ctrl Pts',(-0.408428948108533,1.,-1.8224702267854));
#35584=CARTESIAN_POINT('Ctrl Pts',(-0.410641256301675,-1.,-1.83100408895216));
#35585=CARTESIAN_POINT('Ctrl Pts',(-0.410641256301675,1.,-1.83100408895216));
#35586=CARTESIAN_POINT('Ctrl Pts',(-0.412633125322162,-1.,-1.83808953475839));
#35587=CARTESIAN_POINT('Ctrl Pts',(-0.412633125322162,1.,-1.83808953475839));
#35588=CARTESIAN_POINT('Ctrl Pts',(-0.41448743825434,-1.,-1.8440575707371));
#35589=CARTESIAN_POINT('Ctrl Pts',(-0.41448743825434,1.,-1.8440575707371));
#35590=CARTESIAN_POINT('Ctrl Pts',(-0.416300022038864,-1.,-1.84929312929882));
#35591=CARTESIAN_POINT('Ctrl Pts',(-0.416300022038864,1.,-1.84929312929882));
#35592=CARTESIAN_POINT('Ctrl Pts',(-0.418164129143534,-1.,-1.85417632856234));
#35593=CARTESIAN_POINT('Ctrl Pts',(-0.418164129143534,1.,-1.85417632856234));
#35594=CARTESIAN_POINT('Ctrl Pts',(-0.420157287975619,-1.,-1.85903281096686));
#35595=CARTESIAN_POINT('Ctrl Pts',(-0.420157287975619,1.,-1.85903281096686));
#35596=CARTESIAN_POINT('Ctrl Pts',(-0.422327307418275,-1.,-1.86408083334028));
#35597=CARTESIAN_POINT('Ctrl Pts',(-0.422327307418275,1.,-1.86408083334028));
#35598=CARTESIAN_POINT('Ctrl Pts',(-0.424678177291359,-1.,-1.86937803944323));
#35599=CARTESIAN_POINT('Ctrl Pts',(-0.424678177291359,1.,-1.86937803944323));
#35600=CARTESIAN_POINT('Ctrl Pts',(-0.427183828519102,-1.,-1.87486989291484));
#35601=CARTESIAN_POINT('Ctrl Pts',(-0.427183828519102,1.,-1.87486989291484));
#35602=CARTESIAN_POINT('Ctrl Pts',(-0.429803062482344,-1.,-1.88044229001832));
#35603=CARTESIAN_POINT('Ctrl Pts',(-0.429803062482344,1.,-1.88044229001832));
#35604=CARTESIAN_POINT('Ctrl Pts',(-0.432493038548748,-1.,-1.88596913666793));
#35605=CARTESIAN_POINT('Ctrl Pts',(-0.432493038548748,1.,-1.88596913666793));
#35606=CARTESIAN_POINT('Ctrl Pts',(-0.435225660963383,-1.,-1.89136993975504));
#35607=CARTESIAN_POINT('Ctrl Pts',(-0.435225660963383,1.,-1.89136993975504));
#35608=CARTESIAN_POINT('Ctrl Pts',(-0.437995003948244,-1.,-1.89663648956466));
#35609=CARTESIAN_POINT('Ctrl Pts',(-0.437995003948244,1.,-1.89663648956466));
#35610=CARTESIAN_POINT('Ctrl Pts',(-0.440807833704038,-1.,-1.90180124389086));
#35611=CARTESIAN_POINT('Ctrl Pts',(-0.440807833704038,1.,-1.90180124389086));
#35612=CARTESIAN_POINT('Ctrl Pts',(-0.443677556849151,-1.,-1.90691756144898));
#35613=CARTESIAN_POINT('Ctrl Pts',(-0.443677556849151,1.,-1.90691756144898));
#35614=CARTESIAN_POINT('Ctrl Pts',(-0.446617343485711,-1.,-1.9120369998112));
#35615=CARTESIAN_POINT('Ctrl Pts',(-0.446617343485711,1.,-1.9120369998112));
#35616=CARTESIAN_POINT('Ctrl Pts',(-0.449632260106662,-1.,-1.91718342555755));
#35617=CARTESIAN_POINT('Ctrl Pts',(-0.449632260106662,1.,-1.91718342555755));
#35618=CARTESIAN_POINT('Ctrl Pts',(-0.452719478359432,-1.,-1.92235380648502));
#35619=CARTESIAN_POINT('Ctrl Pts',(-0.452719478359432,1.,-1.92235380648502));
#35620=CARTESIAN_POINT('Ctrl Pts',(-0.455872005174371,-1.,-1.92753067150476));
#35621=CARTESIAN_POINT('Ctrl Pts',(-0.455872005174371,1.,-1.92753067150476));
#35622=CARTESIAN_POINT('Ctrl Pts',(-0.459081234547926,-1.,-1.93269066517934));
#35623=CARTESIAN_POINT('Ctrl Pts',(-0.459081234547926,1.,-1.93269066517934));
#35624=CARTESIAN_POINT('Ctrl Pts',(-0.462340031009056,-1.,-1.93781486640821));
#35625=CARTESIAN_POINT('Ctrl Pts',(-0.462340031009056,1.,-1.93781486640821));
#35626=CARTESIAN_POINT('Ctrl Pts',(-0.46564546202603,-1.,-1.9428979419619));
#35627=CARTESIAN_POINT('Ctrl Pts',(-0.46564546202603,1.,-1.9428979419619));
#35628=CARTESIAN_POINT('Ctrl Pts',(-0.468997482913135,-1.,-1.94794381136514));
#35629=CARTESIAN_POINT('Ctrl Pts',(-0.468997482913135,1.,-1.94794381136514));
#35630=CARTESIAN_POINT('Ctrl Pts',(-0.472397672264072,-1.,-1.95296148278133));
#35631=CARTESIAN_POINT('Ctrl Pts',(-0.472397672264072,1.,-1.95296148278133));
#35632=CARTESIAN_POINT('Ctrl Pts',(-0.475848034683176,-1.,-1.95796111148177));
#35633=CARTESIAN_POINT('Ctrl Pts',(-0.475848034683176,1.,-1.95796111148177));
#35634=CARTESIAN_POINT('Ctrl Pts',(-0.479349583074855,-1.,-1.96294933055943));
#35635=CARTESIAN_POINT('Ctrl Pts',(-0.479349583074855,1.,-1.96294933055943));
#35636=CARTESIAN_POINT('Ctrl Pts',(-0.482901662120691,-1.,-1.96792703422362));
#35637=CARTESIAN_POINT('Ctrl Pts',(-0.482901662120691,1.,-1.96792703422362));
#35638=CARTESIAN_POINT('Ctrl Pts',(-0.486502692907659,-1.,-1.97289186263272));
#35639=CARTESIAN_POINT('Ctrl Pts',(-0.486502692907659,1.,-1.97289186263272));
#35640=CARTESIAN_POINT('Ctrl Pts',(-0.490150627860952,-1.,-1.97783973019229));
#35641=CARTESIAN_POINT('Ctrl Pts',(-0.490150627860952,1.,-1.97783973019229));
#35642=CARTESIAN_POINT('Ctrl Pts',(-0.493843476541495,-1.,-1.98276658761821));
#35643=CARTESIAN_POINT('Ctrl Pts',(-0.493843476541495,1.,-1.98276658761821));
#35644=CARTESIAN_POINT('Ctrl Pts',(-0.497579909545574,-1.,-1.98767044752932));
#35645=CARTESIAN_POINT('Ctrl Pts',(-0.497579909545574,1.,-1.98767044752932));
#35646=CARTESIAN_POINT('Ctrl Pts',(-0.501359287727146,-1.,-1.99255149126155));
#35647=CARTESIAN_POINT('Ctrl Pts',(-0.501359287727146,1.,-1.99255149126155));
#35648=CARTESIAN_POINT('Ctrl Pts',(-0.505181361323026,-1.,-1.99741107463572));
#35649=CARTESIAN_POINT('Ctrl Pts',(-0.505181361323026,1.,-1.99741107463572));
#35650=CARTESIAN_POINT('Ctrl Pts',(-0.509046069886157,-1.,-2.00225107134734));
#35651=CARTESIAN_POINT('Ctrl Pts',(-0.509046069886157,1.,-2.00225107134734));
#35652=CARTESIAN_POINT('Ctrl Pts',(-0.512953306961792,-1.,-2.00707309946949));
#35653=CARTESIAN_POINT('Ctrl Pts',(-0.512953306961792,1.,-2.00707309946949));
#35654=CARTESIAN_POINT('Ctrl Pts',(-0.516902681728687,-1.,-2.01187773939242));
#35655=CARTESIAN_POINT('Ctrl Pts',(-0.516902681728687,1.,-2.01187773939242));
#35656=CARTESIAN_POINT('Ctrl Pts',(-0.52089359039937,-1.,-2.01666477917286));
#35657=CARTESIAN_POINT('Ctrl Pts',(-0.52089359039937,1.,-2.01666477917286));
#35658=CARTESIAN_POINT('Ctrl Pts',(-0.524925318333476,-1.,-2.02143356304698));
#35659=CARTESIAN_POINT('Ctrl Pts',(-0.524925318333476,1.,-2.02143356304698));
#35660=CARTESIAN_POINT('Ctrl Pts',(-0.528997127241914,-1.,-2.0261832908329));
#35661=CARTESIAN_POINT('Ctrl Pts',(-0.528997127241914,1.,-2.0261832908329));
#35662=CARTESIAN_POINT('Ctrl Pts',(-0.533108355132977,-1.,-2.03091336214426));
#35663=CARTESIAN_POINT('Ctrl Pts',(-0.533108355132977,1.,-2.03091336214426));
#35664=CARTESIAN_POINT('Ctrl Pts',(-0.537258489833262,-1.,-2.03562362954037));
#35665=CARTESIAN_POINT('Ctrl Pts',(-0.537258489833262,1.,-2.03562362954037));
#35666=CARTESIAN_POINT('Ctrl Pts',(-0.541447120615659,-1.,-2.04031422690527));
#35667=CARTESIAN_POINT('Ctrl Pts',(-0.541447120615659,1.,-2.04031422690527));
#35668=CARTESIAN_POINT('Ctrl Pts',(-0.54567390381743,-1.,-2.04498544714588));
#35669=CARTESIAN_POINT('Ctrl Pts',(-0.54567390381743,1.,-2.04498544714588));
#35670=CARTESIAN_POINT('Ctrl Pts',(-0.549938525150295,-1.,-2.04963761077958));
#35671=CARTESIAN_POINT('Ctrl Pts',(-0.549938525150295,1.,-2.04963761077958));
#35672=CARTESIAN_POINT('Ctrl Pts',(-0.554240657463906,-1.,-2.05427091604413));
#35673=CARTESIAN_POINT('Ctrl Pts',(-0.554240657463906,1.,-2.05427091604413));
#35674=CARTESIAN_POINT('Ctrl Pts',(-0.558579940185151,-1.,-2.05888537756462));
#35675=CARTESIAN_POINT('Ctrl Pts',(-0.558579940185151,1.,-2.05888537756462));
#35676=CARTESIAN_POINT('Ctrl Pts',(-0.562955993082261,-1.,-2.06348090160589));
#35677=CARTESIAN_POINT('Ctrl Pts',(-0.562955993082261,1.,-2.06348090160589));
#35678=CARTESIAN_POINT('Ctrl Pts',(-0.567368421181087,-1.,-2.06805732997334));
#35679=CARTESIAN_POINT('Ctrl Pts',(-0.567368421181087,1.,-2.06805732997334));
#35680=CARTESIAN_POINT('Ctrl Pts',(-0.571816823242603,-1.,-2.07261449292824));
#35681=CARTESIAN_POINT('Ctrl Pts',(-0.571816823242603,1.,-2.07261449292824));
#35682=CARTESIAN_POINT('Ctrl Pts',(-0.576300797416844,-1.,-2.07715226767559));
#35683=CARTESIAN_POINT('Ctrl Pts',(-0.576300797416844,1.,-2.07715226767559));
#35684=CARTESIAN_POINT('Ctrl Pts',(-0.580819952108063,-1.,-2.08167059018418));
#35685=CARTESIAN_POINT('Ctrl Pts',(-0.580819952108063,1.,-2.08167059018418));
#35686=CARTESIAN_POINT('Ctrl Pts',(-0.585373918991617,-1.,-2.08616943727951));
#35687=CARTESIAN_POINT('Ctrl Pts',(-0.585373918991617,1.,-2.08616943727951));
#35688=CARTESIAN_POINT('Ctrl Pts',(-0.589962365403406,-1.,-2.09064881812129));
#35689=CARTESIAN_POINT('Ctrl Pts',(-0.589962365403406,1.,-2.09064881812129));
#35690=CARTESIAN_POINT('Ctrl Pts',(-0.594585006052162,-1.,-2.0951087622027));
#35691=CARTESIAN_POINT('Ctrl Pts',(-0.594585006052162,1.,-2.0951087622027));
#35692=CARTESIAN_POINT('Ctrl Pts',(-0.599241616420533,-1.,-2.0995493086477));
#35693=CARTESIAN_POINT('Ctrl Pts',(-0.599241616420533,1.,-2.0995493086477));
#35694=CARTESIAN_POINT('Ctrl Pts',(-0.60393203073603,-1.,-2.10397049886949));
#35695=CARTESIAN_POINT('Ctrl Pts',(-0.60393203073603,1.,-2.10397049886949));
#35696=CARTESIAN_POINT('Ctrl Pts',(-0.607711315454876,-1.,-2.1074919961518));
#35697=CARTESIAN_POINT('Ctrl Pts',(-0.607711315454876,1.,-2.1074919961518));
#35698=CARTESIAN_POINT('Ctrl Pts',(-0.610560911689899,-1.,-2.11012443807238));
#35699=CARTESIAN_POINT('Ctrl Pts',(-0.610560911689899,1.,-2.11012443807238));
#35700=CARTESIAN_POINT('Ctrl Pts',(-0.6124673655618,-1.,-2.11187554259986));
#35701=CARTESIAN_POINT('Ctrl Pts',(-0.6124673655618,1.,-2.11187554259986));
#35702=CARTESIAN_POINT('Ctrl Pts',(-0.61342227326009,-1.,-2.11275013067528));
#35703=CARTESIAN_POINT('Ctrl Pts',(-0.61342227326009,1.,-2.11275013067528));
#35704=CARTESIAN_POINT('',(-0.383122945602004,1.,-1.7075470150345));
#35705=CARTESIAN_POINT('Ctrl Pts',(-0.383122945602004,1.,-1.7075470150345));
#35706=CARTESIAN_POINT('Ctrl Pts',(-0.384119047315542,1.,-1.71231062891958));
#35707=CARTESIAN_POINT('Ctrl Pts',(-0.38607079032701,1.,-1.72162022246158));
#35708=CARTESIAN_POINT('Ctrl Pts',(-0.388877023509191,1.,-1.7349317097561));
#35709=CARTESIAN_POINT('Ctrl Pts',(-0.392375812294307,1.,-1.75137405313962));
#35710=CARTESIAN_POINT('Ctrl Pts',(-0.39634619612042,1.,-1.7697556004756));
#35711=CARTESIAN_POINT('Ctrl Pts',(-0.39991940378308,1.,-1.78598826347533));
#35712=CARTESIAN_POINT('Ctrl Pts',(-0.403107976170441,1.,-1.80012077176221));
#35713=CARTESIAN_POINT('Ctrl Pts',(-0.405933518411838,1.,-1.81223801813988));
#35714=CARTESIAN_POINT('Ctrl Pts',(-0.408428948108533,1.,-1.8224702267854));
#35715=CARTESIAN_POINT('Ctrl Pts',(-0.410641256301675,1.,-1.83100408895216));
#35716=CARTESIAN_POINT('Ctrl Pts',(-0.412633125322162,1.,-1.83808953475839));
#35717=CARTESIAN_POINT('Ctrl Pts',(-0.41448743825434,1.,-1.8440575707371));
#35718=CARTESIAN_POINT('Ctrl Pts',(-0.416300022038864,1.,-1.84929312929882));
#35719=CARTESIAN_POINT('Ctrl Pts',(-0.418164129143534,1.,-1.85417632856234));
#35720=CARTESIAN_POINT('Ctrl Pts',(-0.420157287975619,1.,-1.85903281096686));
#35721=CARTESIAN_POINT('Ctrl Pts',(-0.422327307418275,1.,-1.86408083334028));
#35722=CARTESIAN_POINT('Ctrl Pts',(-0.424678177291359,1.,-1.86937803944323));
#35723=CARTESIAN_POINT('Ctrl Pts',(-0.427183828519102,1.,-1.87486989291484));
#35724=CARTESIAN_POINT('Ctrl Pts',(-0.429803062482344,1.,-1.88044229001832));
#35725=CARTESIAN_POINT('Ctrl Pts',(-0.432493038548748,1.,-1.88596913666793));
#35726=CARTESIAN_POINT('Ctrl Pts',(-0.435225660963383,1.,-1.89136993975504));
#35727=CARTESIAN_POINT('Ctrl Pts',(-0.437995003948244,1.,-1.89663648956466));
#35728=CARTESIAN_POINT('Ctrl Pts',(-0.440807833704038,1.,-1.90180124389086));
#35729=CARTESIAN_POINT('Ctrl Pts',(-0.443677556849151,1.,-1.90691756144898));
#35730=CARTESIAN_POINT('Ctrl Pts',(-0.446617343485711,1.,-1.9120369998112));
#35731=CARTESIAN_POINT('Ctrl Pts',(-0.449632260106662,1.,-1.91718342555755));
#35732=CARTESIAN_POINT('Ctrl Pts',(-0.452719478359432,1.,-1.92235380648502));
#35733=CARTESIAN_POINT('Ctrl Pts',(-0.455872005174371,1.,-1.92753067150476));
#35734=CARTESIAN_POINT('Ctrl Pts',(-0.459081234547926,1.,-1.93269066517934));
#35735=CARTESIAN_POINT('Ctrl Pts',(-0.462340031009056,1.,-1.93781486640821));
#35736=CARTESIAN_POINT('Ctrl Pts',(-0.46564546202603,1.,-1.9428979419619));
#35737=CARTESIAN_POINT('Ctrl Pts',(-0.468997482913135,1.,-1.94794381136514));
#35738=CARTESIAN_POINT('Ctrl Pts',(-0.472397672264072,1.,-1.95296148278133));
#35739=CARTESIAN_POINT('Ctrl Pts',(-0.475848034683176,1.,-1.95796111148177));
#35740=CARTESIAN_POINT('Ctrl Pts',(-0.479349583074855,1.,-1.96294933055943));
#35741=CARTESIAN_POINT('Ctrl Pts',(-0.482901662120691,1.,-1.96792703422362));
#35742=CARTESIAN_POINT('Ctrl Pts',(-0.486502692907659,1.,-1.97289186263272));
#35743=CARTESIAN_POINT('Ctrl Pts',(-0.490150627860952,1.,-1.97783973019229));
#35744=CARTESIAN_POINT('Ctrl Pts',(-0.493843476541495,1.,-1.98276658761821));
#35745=CARTESIAN_POINT('Ctrl Pts',(-0.497579909545574,1.,-1.98767044752932));
#35746=CARTESIAN_POINT('Ctrl Pts',(-0.501359287727146,1.,-1.99255149126155));
#35747=CARTESIAN_POINT('Ctrl Pts',(-0.505181361323026,1.,-1.99741107463572));
#35748=CARTESIAN_POINT('Ctrl Pts',(-0.509046069886157,1.,-2.00225107134734));
#35749=CARTESIAN_POINT('Ctrl Pts',(-0.512953306961792,1.,-2.00707309946949));
#35750=CARTESIAN_POINT('Ctrl Pts',(-0.516902681728687,1.,-2.01187773939242));
#35751=CARTESIAN_POINT('Ctrl Pts',(-0.52089359039937,1.,-2.01666477917286));
#35752=CARTESIAN_POINT('Ctrl Pts',(-0.524925318333476,1.,-2.02143356304698));
#35753=CARTESIAN_POINT('Ctrl Pts',(-0.528997127241914,1.,-2.0261832908329));
#35754=CARTESIAN_POINT('Ctrl Pts',(-0.533108355132977,1.,-2.03091336214426));
#35755=CARTESIAN_POINT('Ctrl Pts',(-0.537258489833262,1.,-2.03562362954037));
#35756=CARTESIAN_POINT('Ctrl Pts',(-0.541447120615659,1.,-2.04031422690527));
#35757=CARTESIAN_POINT('Ctrl Pts',(-0.54567390381743,1.,-2.04498544714588));
#35758=CARTESIAN_POINT('Ctrl Pts',(-0.549938525150295,1.,-2.04963761077958));
#35759=CARTESIAN_POINT('Ctrl Pts',(-0.554240657463906,1.,-2.05427091604413));
#35760=CARTESIAN_POINT('Ctrl Pts',(-0.558579940185151,1.,-2.05888537756462));
#35761=CARTESIAN_POINT('Ctrl Pts',(-0.562955993082261,1.,-2.06348090160589));
#35762=CARTESIAN_POINT('Ctrl Pts',(-0.567368421181087,1.,-2.06805732997334));
#35763=CARTESIAN_POINT('Ctrl Pts',(-0.571816823242603,1.,-2.07261449292824));
#35764=CARTESIAN_POINT('Ctrl Pts',(-0.576300797416844,1.,-2.07715226767559));
#35765=CARTESIAN_POINT('Ctrl Pts',(-0.580819952108063,1.,-2.08167059018418));
#35766=CARTESIAN_POINT('Ctrl Pts',(-0.585373918991617,1.,-2.08616943727951));
#35767=CARTESIAN_POINT('Ctrl Pts',(-0.589962365403406,1.,-2.09064881812129));
#35768=CARTESIAN_POINT('Ctrl Pts',(-0.594585006052162,1.,-2.0951087622027));
#35769=CARTESIAN_POINT('Ctrl Pts',(-0.599241616420533,1.,-2.0995493086477));
#35770=CARTESIAN_POINT('Ctrl Pts',(-0.60393203073603,1.,-2.10397049886949));
#35771=CARTESIAN_POINT('Ctrl Pts',(-0.607711315454876,1.,-2.1074919961518));
#35772=CARTESIAN_POINT('Ctrl Pts',(-0.610560911689899,1.,-2.11012443807238));
#35773=CARTESIAN_POINT('Ctrl Pts',(-0.6124673655618,1.,-2.11187554259986));
#35774=CARTESIAN_POINT('Ctrl Pts',(-0.61342227326009,1.,-2.11275013067528));
#35775=CARTESIAN_POINT('',(-0.383122945602003,0.,-1.7075470150345));
#35776=CARTESIAN_POINT('Origin',(0.,0.,0.));
#35777=CARTESIAN_POINT('',(-0.163289472382896,1.,-1.74236521665491));
#35778=CARTESIAN_POINT('Origin',(0.,1.,0.));
#35779=CARTESIAN_POINT('',(-0.163289472382896,0.,-1.74236521665491));
#35780=CARTESIAN_POINT('Ctrl Pts',(-0.0694764450219581,-1.,-2.19890268624765));
#35781=CARTESIAN_POINT('Ctrl Pts',(-0.0694764450219581,1.,-2.19890268624765));
#35782=CARTESIAN_POINT('Ctrl Pts',(-0.070114353632549,-1.,-2.19777582085423));
#35783=CARTESIAN_POINT('Ctrl Pts',(-0.070114353632549,1.,-2.19777582085423));
#35784=CARTESIAN_POINT('Ctrl Pts',(-0.0713863779526154,-1.,-2.19552129484002));
#35785=CARTESIAN_POINT('Ctrl Pts',(-0.0713863779526154,1.,-2.19552129484002));
#35786=CARTESIAN_POINT('Ctrl Pts',(-0.0732830357306725,-1.,-2.19213712013662));
#35787=CARTESIAN_POINT('Ctrl Pts',(-0.0732830357306725,1.,-2.19213712013662));
#35788=CARTESIAN_POINT('Ctrl Pts',(-0.0757891465836148,-1.,-2.1876201139953));
#35789=CARTESIAN_POINT('Ctrl Pts',(-0.0757891465836148,1.,-2.1876201139953));
#35790=CARTESIAN_POINT('Ctrl Pts',(-0.0788837727685243,-1.,-2.18196589448887));
#35791=CARTESIAN_POINT('Ctrl Pts',(-0.0788837727685243,1.,-2.18196589448887));
#35792=CARTESIAN_POINT('Ctrl Pts',(-0.0819402680872765,-1.,-2.176303712113));
#35793=CARTESIAN_POINT('Ctrl Pts',(-0.0819402680872765,1.,-2.176303712113));
#35794=CARTESIAN_POINT('Ctrl Pts',(-0.0849584620835372,-1.,-2.17063357870952));
#35795=CARTESIAN_POINT('Ctrl Pts',(-0.0849584620835372,1.,-2.17063357870952));
#35796=CARTESIAN_POINT('Ctrl Pts',(-0.0879381291386923,-1.,-2.16495552645014));
#35797=CARTESIAN_POINT('Ctrl Pts',(-0.0879381291386923,1.,-2.16495552645014));
#35798=CARTESIAN_POINT('Ctrl Pts',(-0.0908789888107265,-1.,-2.15926961544516));
#35799=CARTESIAN_POINT('Ctrl Pts',(-0.0908789888107265,1.,-2.15926961544516));
#35800=CARTESIAN_POINT('Ctrl Pts',(-0.0937807218867643,-1.,-2.1535759397817));
#35801=CARTESIAN_POINT('Ctrl Pts',(-0.0937807218867643,1.,-2.1535759397817));
#35802=CARTESIAN_POINT('Ctrl Pts',(-0.0966429852305459,-1.,-2.14787463531795));
#35803=CARTESIAN_POINT('Ctrl Pts',(-0.0966429852305459,1.,-2.14787463531795));
#35804=CARTESIAN_POINT('Ctrl Pts',(-0.0994654261990915,-1.,-2.14216588396025));
#35805=CARTESIAN_POINT('Ctrl Pts',(-0.0994654261990915,1.,-2.14216588396025));
#35806=CARTESIAN_POINT('Ctrl Pts',(-0.1022477005561,-1.,-2.13644992667165));
#35807=CARTESIAN_POINT('Ctrl Pts',(-0.1022477005561,1.,-2.13644992667165));
#35808=CARTESIAN_POINT('Ctrl Pts',(-0.104989479152739,-1.,-2.13072704887293));
#35809=CARTESIAN_POINT('Ctrl Pts',(-0.104989479152739,1.,-2.13072704887293));
#35810=CARTESIAN_POINT('Ctrl Pts',(-0.10769043523109,-1.,-2.12499752307));
#35811=CARTESIAN_POINT('Ctrl Pts',(-0.10769043523109,1.,-2.12499752307));
#35812=CARTESIAN_POINT('Ctrl Pts',(-0.110350236135025,-1.,-2.11926155590865));
#35813=CARTESIAN_POINT('Ctrl Pts',(-0.110350236135025,1.,-2.11926155590865));
#35814=CARTESIAN_POINT('Ctrl Pts',(-0.112968534419737,-1.,-2.11351924490306));
#35815=CARTESIAN_POINT('Ctrl Pts',(-0.112968534419737,1.,-2.11351924490306));
#35816=CARTESIAN_POINT('Ctrl Pts',(-0.115544957687926,-1.,-2.10777050261309));
#35817=CARTESIAN_POINT('Ctrl Pts',(-0.115544957687926,1.,-2.10777050261309));
#35818=CARTESIAN_POINT('Ctrl Pts',(-0.118079107988355,-1.,-2.102015121329));
#35819=CARTESIAN_POINT('Ctrl Pts',(-0.118079107988355,1.,-2.102015121329));
#35820=CARTESIAN_POINT('Ctrl Pts',(-0.120570567965122,-1.,-2.0962529286773));
#35821=CARTESIAN_POINT('Ctrl Pts',(-0.120570567965122,1.,-2.0962529286773));
#35822=CARTESIAN_POINT('Ctrl Pts',(-0.123018905621083,-1.,-2.09048392424825));
#35823=CARTESIAN_POINT('Ctrl Pts',(-0.123018905621083,1.,-2.09048392424825));
#35824=CARTESIAN_POINT('Ctrl Pts',(-0.125423679412061,-1.,-2.08470840653643));
#35825=CARTESIAN_POINT('Ctrl Pts',(-0.125423679412061,1.,-2.08470840653643));
#35826=CARTESIAN_POINT('Ctrl Pts',(-0.12778444527612,-1.,-2.07892715110987));
#35827=CARTESIAN_POINT('Ctrl Pts',(-0.12778444527612,1.,-2.07892715110987));
#35828=CARTESIAN_POINT('Ctrl Pts',(-0.130100748328403,-1.,-2.07314114713063));
#35829=CARTESIAN_POINT('Ctrl Pts',(-0.130100748328403,1.,-2.07314114713063));
#35830=CARTESIAN_POINT('Ctrl Pts',(-0.13237211154771,-1.,-2.06735123910326));
#35831=CARTESIAN_POINT('Ctrl Pts',(-0.13237211154771,1.,-2.06735123910326));
#35832=CARTESIAN_POINT('Ctrl Pts',(-0.134598026192106,-1.,-2.06155781517842));
#35833=CARTESIAN_POINT('Ctrl Pts',(-0.134598026192106,1.,-2.06155781517842));
#35834=CARTESIAN_POINT('Ctrl Pts',(-0.136777941218044,-1.,-2.05576044414264));
#35835=CARTESIAN_POINT('Ctrl Pts',(-0.136777941218044,1.,-2.05576044414264));
#35836=CARTESIAN_POINT('Ctrl Pts',(-0.138911255368966,-1.,-2.04995762001328));
#35837=CARTESIAN_POINT('Ctrl Pts',(-0.138911255368966,1.,-2.04995762001328));
#35838=CARTESIAN_POINT('Ctrl Pts',(-0.140997332152546,-1.,-2.04414757947916));
#35839=CARTESIAN_POINT('Ctrl Pts',(-0.140997332152546,1.,-2.04414757947916));
#35840=CARTESIAN_POINT('Ctrl Pts',(-0.143035515058209,-1.,-2.03832911025912));
#35841=CARTESIAN_POINT('Ctrl Pts',(-0.143035515058209,1.,-2.03832911025912));
#35842=CARTESIAN_POINT('Ctrl Pts',(-0.145025140186057,-1.,-2.03250223739942));
#35843=CARTESIAN_POINT('Ctrl Pts',(-0.145025140186057,1.,-2.03250223739942));
#35844=CARTESIAN_POINT('Ctrl Pts',(-0.146965557332583,-1.,-2.02666926182017));
#35845=CARTESIAN_POINT('Ctrl Pts',(-0.146965557332583,1.,-2.02666926182017));
#35846=CARTESIAN_POINT('Ctrl Pts',(-0.148856124775337,-1.,-2.02083464969894));
#35847=CARTESIAN_POINT('Ctrl Pts',(-0.148856124775337,1.,-2.02083464969894));
#35848=CARTESIAN_POINT('Ctrl Pts',(-0.150696157673078,-1.,-2.01500291940238));
#35849=CARTESIAN_POINT('Ctrl Pts',(-0.150696157673078,1.,-2.01500291940238));
#35850=CARTESIAN_POINT('Ctrl Pts',(-0.15248488362145,-1.,-2.00917680318424));
#35851=CARTESIAN_POINT('Ctrl Pts',(-0.15248488362145,1.,-2.00917680318424));
#35852=CARTESIAN_POINT('Ctrl Pts',(-0.154221403049722,-1.,-2.00335565310543));
#35853=CARTESIAN_POINT('Ctrl Pts',(-0.154221403049722,1.,-2.00335565310543));
#35854=CARTESIAN_POINT('Ctrl Pts',(-0.155904629548783,-1.,-1.99753284771497));
#35855=CARTESIAN_POINT('Ctrl Pts',(-0.155904629548783,1.,-1.99753284771497));
#35856=CARTESIAN_POINT('Ctrl Pts',(-0.157533331459227,-1.,-1.99169810931908));
#35857=CARTESIAN_POINT('Ctrl Pts',(-0.157533331459227,1.,-1.99169810931908));
#35858=CARTESIAN_POINT('Ctrl Pts',(-0.159106226437299,-1.,-1.98584238283292));
#35859=CARTESIAN_POINT('Ctrl Pts',(-0.159106226437299,1.,-1.98584238283292));
#35860=CARTESIAN_POINT('Ctrl Pts',(-0.160622060784611,-1.,-1.97996195437559));
#35861=CARTESIAN_POINT('Ctrl Pts',(-0.160622060784611,1.,-1.97996195437559));
#35862=CARTESIAN_POINT('Ctrl Pts',(-0.162079693556289,-1.,-1.97406280235188));
#35863=CARTESIAN_POINT('Ctrl Pts',(-0.162079693556289,1.,-1.97406280235188));
#35864=CARTESIAN_POINT('Ctrl Pts',(-0.163478185457734,-1.,-1.96816512677967));
#35865=CARTESIAN_POINT('Ctrl Pts',(-0.163478185457734,1.,-1.96816512677967));
#35866=CARTESIAN_POINT('Ctrl Pts',(-0.164816568920269,-1.,-1.96229379940136));
#35867=CARTESIAN_POINT('Ctrl Pts',(-0.164816568920269,1.,-1.96229379940136));
#35868=CARTESIAN_POINT('Ctrl Pts',(-0.166093592002812,-1.,-1.9564675971873));
#35869=CARTESIAN_POINT('Ctrl Pts',(-0.166093592002812,1.,-1.9564675971873));
#35870=CARTESIAN_POINT('Ctrl Pts',(-0.167307501784475,-1.,-1.95069027794294));
#35871=CARTESIAN_POINT('Ctrl Pts',(-0.167307501784475,1.,-1.95069027794294));
#35872=CARTESIAN_POINT('Ctrl Pts',(-0.168455741607556,-1.,-1.94493757756931));
#35873=CARTESIAN_POINT('Ctrl Pts',(-0.168455741607556,1.,-1.94493757756931));
#35874=CARTESIAN_POINT('Ctrl Pts',(-0.169534904817491,-1.,-1.93915639211581));
#35875=CARTESIAN_POINT('Ctrl Pts',(-0.169534904817491,1.,-1.93915639211581));
#35876=CARTESIAN_POINT('Ctrl Pts',(-0.170541253116202,-1.,-1.93329183155539));
#35877=CARTESIAN_POINT('Ctrl Pts',(-0.170541253116202,1.,-1.93329183155539));
#35878=CARTESIAN_POINT('Ctrl Pts',(-0.171471191532988,-1.,-1.92731093582036));
#35879=CARTESIAN_POINT('Ctrl Pts',(-0.171471191532988,1.,-1.92731093582036));
#35880=CARTESIAN_POINT('Ctrl Pts',(-0.172321621259514,-1.,-1.9212233439798));
#35881=CARTESIAN_POINT('Ctrl Pts',(-0.172321621259514,1.,-1.9212233439798));
#35882=CARTESIAN_POINT('Ctrl Pts',(-0.173090695383496,-1.,-1.91511429159527));
#35883=CARTESIAN_POINT('Ctrl Pts',(-0.173090695383496,1.,-1.91511429159527));
#35884=CARTESIAN_POINT('Ctrl Pts',(-0.173776635257817,-1.,-1.90911693975267));
#35885=CARTESIAN_POINT('Ctrl Pts',(-0.173776635257817,1.,-1.90911693975267));
#35886=CARTESIAN_POINT('Ctrl Pts',(-0.174375518661085,-1.,-1.90335253862834));
#35887=CARTESIAN_POINT('Ctrl Pts',(-0.174375518661085,1.,-1.90335253862834));
#35888=CARTESIAN_POINT('Ctrl Pts',(-0.174879405091263,-1.,-1.89788101117132));
#35889=CARTESIAN_POINT('Ctrl Pts',(-0.174879405091263,1.,-1.89788101117132));
#35890=CARTESIAN_POINT('Ctrl Pts',(-0.175274276190844,-1.,-1.892646301985));
#35891=CARTESIAN_POINT('Ctrl Pts',(-0.175274276190844,1.,-1.892646301985));
#35892=CARTESIAN_POINT('Ctrl Pts',(-0.175538155840648,-1.,-1.88742606273259));
#35893=CARTESIAN_POINT('Ctrl Pts',(-0.175538155840648,1.,-1.88742606273259));
#35894=CARTESIAN_POINT('Ctrl Pts',(-0.175644148889699,-1.,-1.88188663145367));
#35895=CARTESIAN_POINT('Ctrl Pts',(-0.175644148889699,1.,-1.88188663145367));
#35896=CARTESIAN_POINT('Ctrl Pts',(-0.175563480746485,-1.,-1.87563767773588));
#35897=CARTESIAN_POINT('Ctrl Pts',(-0.175563480746485,1.,-1.87563767773588));
#35898=CARTESIAN_POINT('Ctrl Pts',(-0.175268337590758,-1.,-1.86828349694799));
#35899=CARTESIAN_POINT('Ctrl Pts',(-0.175268337590758,1.,-1.86828349694799));
#35900=CARTESIAN_POINT('Ctrl Pts',(-0.17473525927603,-1.,-1.85948367088837));
#35901=CARTESIAN_POINT('Ctrl Pts',(-0.17473525927603,1.,-1.85948367088837));
#35902=CARTESIAN_POINT('Ctrl Pts',(-0.173946627587731,-1.,-1.8489811319852));
#35903=CARTESIAN_POINT('Ctrl Pts',(-0.173946627587731,1.,-1.8489811319852));
#35904=CARTESIAN_POINT('Ctrl Pts',(-0.1728894428919,-1.,-1.83658380527692));
#35905=CARTESIAN_POINT('Ctrl Pts',(-0.1728894428919,1.,-1.83658380527692));
#35906=CARTESIAN_POINT('Ctrl Pts',(-0.171554770204119,-1.,-1.82215766811545));
#35907=CARTESIAN_POINT('Ctrl Pts',(-0.171554770204119,1.,-1.82215766811545));
#35908=CARTESIAN_POINT('Ctrl Pts',(-0.169936923904608,-1.,-1.80561530629706));
#35909=CARTESIAN_POINT('Ctrl Pts',(-0.169936923904608,1.,-1.80561530629706));
#35910=CARTESIAN_POINT('Ctrl Pts',(-0.168032772805197,-1.,-1.7869064998507));
#35911=CARTESIAN_POINT('Ctrl Pts',(-0.168032772805197,1.,-1.7869064998507));
#35912=CARTESIAN_POINT('Ctrl Pts',(-0.1662793551464,-1.,-1.77018771684844));
#35913=CARTESIAN_POINT('Ctrl Pts',(-0.1662793551464,1.,-1.77018771684844));
#35914=CARTESIAN_POINT('Ctrl Pts',(-0.164834765707158,-1.,-1.75666056638427));
#35915=CARTESIAN_POINT('Ctrl Pts',(-0.164834765707158,1.,-1.75666056638427));
#35916=CARTESIAN_POINT('Ctrl Pts',(-0.163814161002002,-1.,-1.7472034950333));
#35917=CARTESIAN_POINT('Ctrl Pts',(-0.163814161002002,1.,-1.7472034950333));
#35918=CARTESIAN_POINT('Ctrl Pts',(-0.163289472382896,-1.,-1.74236521665491));
#35919=CARTESIAN_POINT('Ctrl Pts',(-0.163289472382896,1.,-1.74236521665491));
#35920=CARTESIAN_POINT('',(-0.0694764450219581,1.,-2.19890268624765));
#35921=CARTESIAN_POINT('Ctrl Pts',(-0.0694764450219581,1.,-2.19890268624765));
#35922=CARTESIAN_POINT('Ctrl Pts',(-0.070114353632549,1.,-2.19777582085423));
#35923=CARTESIAN_POINT('Ctrl Pts',(-0.0713863779526154,1.,-2.19552129484002));
#35924=CARTESIAN_POINT('Ctrl Pts',(-0.0732830357306725,1.,-2.19213712013662));
#35925=CARTESIAN_POINT('Ctrl Pts',(-0.0757891465836148,1.,-2.1876201139953));
#35926=CARTESIAN_POINT('Ctrl Pts',(-0.0788837727685243,1.,-2.18196589448887));
#35927=CARTESIAN_POINT('Ctrl Pts',(-0.0819402680872765,1.,-2.176303712113));
#35928=CARTESIAN_POINT('Ctrl Pts',(-0.0849584620835372,1.,-2.17063357870952));
#35929=CARTESIAN_POINT('Ctrl Pts',(-0.0879381291386923,1.,-2.16495552645014));
#35930=CARTESIAN_POINT('Ctrl Pts',(-0.0908789888107265,1.,-2.15926961544516));
#35931=CARTESIAN_POINT('Ctrl Pts',(-0.0937807218867643,1.,-2.1535759397817));
#35932=CARTESIAN_POINT('Ctrl Pts',(-0.0966429852305459,1.,-2.14787463531795));
#35933=CARTESIAN_POINT('Ctrl Pts',(-0.0994654261990915,1.,-2.14216588396025));
#35934=CARTESIAN_POINT('Ctrl Pts',(-0.1022477005561,1.,-2.13644992667165));
#35935=CARTESIAN_POINT('Ctrl Pts',(-0.104989479152739,1.,-2.13072704887293));
#35936=CARTESIAN_POINT('Ctrl Pts',(-0.10769043523109,1.,-2.12499752307));
#35937=CARTESIAN_POINT('Ctrl Pts',(-0.110350236135025,1.,-2.11926155590865));
#35938=CARTESIAN_POINT('Ctrl Pts',(-0.112968534419737,1.,-2.11351924490306));
#35939=CARTESIAN_POINT('Ctrl Pts',(-0.115544957687926,1.,-2.10777050261309));
#35940=CARTESIAN_POINT('Ctrl Pts',(-0.118079107988355,1.,-2.102015121329));
#35941=CARTESIAN_POINT('Ctrl Pts',(-0.120570567965122,1.,-2.0962529286773));
#35942=CARTESIAN_POINT('Ctrl Pts',(-0.123018905621083,1.,-2.09048392424825));
#35943=CARTESIAN_POINT('Ctrl Pts',(-0.125423679412061,1.,-2.08470840653643));
#35944=CARTESIAN_POINT('Ctrl Pts',(-0.12778444527612,1.,-2.07892715110987));
#35945=CARTESIAN_POINT('Ctrl Pts',(-0.130100748328403,1.,-2.07314114713063));
#35946=CARTESIAN_POINT('Ctrl Pts',(-0.13237211154771,1.,-2.06735123910326));
#35947=CARTESIAN_POINT('Ctrl Pts',(-0.134598026192106,1.,-2.06155781517842));
#35948=CARTESIAN_POINT('Ctrl Pts',(-0.136777941218044,1.,-2.05576044414264));
#35949=CARTESIAN_POINT('Ctrl Pts',(-0.138911255368966,1.,-2.04995762001328));
#35950=CARTESIAN_POINT('Ctrl Pts',(-0.140997332152546,1.,-2.04414757947916));
#35951=CARTESIAN_POINT('Ctrl Pts',(-0.143035515058209,1.,-2.03832911025912));
#35952=CARTESIAN_POINT('Ctrl Pts',(-0.145025140186057,1.,-2.03250223739942));
#35953=CARTESIAN_POINT('Ctrl Pts',(-0.146965557332583,1.,-2.02666926182017));
#35954=CARTESIAN_POINT('Ctrl Pts',(-0.148856124775337,1.,-2.02083464969894));
#35955=CARTESIAN_POINT('Ctrl Pts',(-0.150696157673078,1.,-2.01500291940238));
#35956=CARTESIAN_POINT('Ctrl Pts',(-0.15248488362145,1.,-2.00917680318424));
#35957=CARTESIAN_POINT('Ctrl Pts',(-0.154221403049722,1.,-2.00335565310543));
#35958=CARTESIAN_POINT('Ctrl Pts',(-0.155904629548783,1.,-1.99753284771497));
#35959=CARTESIAN_POINT('Ctrl Pts',(-0.157533331459227,1.,-1.99169810931908));
#35960=CARTESIAN_POINT('Ctrl Pts',(-0.159106226437299,1.,-1.98584238283292));
#35961=CARTESIAN_POINT('Ctrl Pts',(-0.160622060784611,1.,-1.97996195437559));
#35962=CARTESIAN_POINT('Ctrl Pts',(-0.162079693556289,1.,-1.97406280235188));
#35963=CARTESIAN_POINT('Ctrl Pts',(-0.163478185457734,1.,-1.96816512677967));
#35964=CARTESIAN_POINT('Ctrl Pts',(-0.164816568920269,1.,-1.96229379940136));
#35965=CARTESIAN_POINT('Ctrl Pts',(-0.166093592002812,1.,-1.9564675971873));
#35966=CARTESIAN_POINT('Ctrl Pts',(-0.167307501784475,1.,-1.95069027794294));
#35967=CARTESIAN_POINT('Ctrl Pts',(-0.168455741607556,1.,-1.94493757756931));
#35968=CARTESIAN_POINT('Ctrl Pts',(-0.169534904817491,1.,-1.93915639211581));
#35969=CARTESIAN_POINT('Ctrl Pts',(-0.170541253116202,1.,-1.93329183155539));
#35970=CARTESIAN_POINT('Ctrl Pts',(-0.171471191532988,1.,-1.92731093582036));
#35971=CARTESIAN_POINT('Ctrl Pts',(-0.172321621259514,1.,-1.9212233439798));
#35972=CARTESIAN_POINT('Ctrl Pts',(-0.173090695383496,1.,-1.91511429159527));
#35973=CARTESIAN_POINT('Ctrl Pts',(-0.173776635257817,1.,-1.90911693975267));
#35974=CARTESIAN_POINT('Ctrl Pts',(-0.174375518661085,1.,-1.90335253862834));
#35975=CARTESIAN_POINT('Ctrl Pts',(-0.174879405091263,1.,-1.89788101117132));
#35976=CARTESIAN_POINT('Ctrl Pts',(-0.175274276190844,1.,-1.892646301985));
#35977=CARTESIAN_POINT('Ctrl Pts',(-0.175538155840648,1.,-1.88742606273259));
#35978=CARTESIAN_POINT('Ctrl Pts',(-0.175644148889699,1.,-1.88188663145367));
#35979=CARTESIAN_POINT('Ctrl Pts',(-0.175563480746485,1.,-1.87563767773588));
#35980=CARTESIAN_POINT('Ctrl Pts',(-0.175268337590758,1.,-1.86828349694799));
#35981=CARTESIAN_POINT('Ctrl Pts',(-0.17473525927603,1.,-1.85948367088837));
#35982=CARTESIAN_POINT('Ctrl Pts',(-0.173946627587731,1.,-1.8489811319852));
#35983=CARTESIAN_POINT('Ctrl Pts',(-0.1728894428919,1.,-1.83658380527692));
#35984=CARTESIAN_POINT('Ctrl Pts',(-0.171554770204119,1.,-1.82215766811545));
#35985=CARTESIAN_POINT('Ctrl Pts',(-0.169936923904608,1.,-1.80561530629706));
#35986=CARTESIAN_POINT('Ctrl Pts',(-0.168032772805197,1.,-1.7869064998507));
#35987=CARTESIAN_POINT('Ctrl Pts',(-0.1662793551464,1.,-1.77018771684844));
#35988=CARTESIAN_POINT('Ctrl Pts',(-0.164834765707158,1.,-1.75666056638427));
#35989=CARTESIAN_POINT('Ctrl Pts',(-0.163814161002002,1.,-1.7472034950333));
#35990=CARTESIAN_POINT('Ctrl Pts',(-0.163289472382896,1.,-1.74236521665491));
#35991=CARTESIAN_POINT('',(-0.0694764450219581,0.,-2.19890268624765));
#35992=CARTESIAN_POINT('Origin',(0.0694764450219584,0.,-2.19890268624765));
#35993=CARTESIAN_POINT('',(0.0694764450219584,1.,-2.19890268624765));
#35994=CARTESIAN_POINT('',(-0.0694764450219581,1.,-2.19890268624765));
#35995=CARTESIAN_POINT('',(0.0694764450219584,0.,-2.19890268624765));
#35996=CARTESIAN_POINT('Ctrl Pts',(0.163289472382896,-1.,-1.74236521665491));
#35997=CARTESIAN_POINT('Ctrl Pts',(0.163289472382896,1.,-1.74236521665491));
#35998=CARTESIAN_POINT('Ctrl Pts',(0.163814161002474,-1.,-1.74720349503904));
#35999=CARTESIAN_POINT('Ctrl Pts',(0.163814161002474,1.,-1.74720349503904));
#36000=CARTESIAN_POINT('Ctrl Pts',(0.164834765708484,-1.,-1.75666056640041));
#36001=CARTESIAN_POINT('Ctrl Pts',(0.164834765708484,1.,-1.75666056640041));
#36002=CARTESIAN_POINT('Ctrl Pts',(0.166279355148738,-1.,-1.77018771687692));
#36003=CARTESIAN_POINT('Ctrl Pts',(0.166279355148738,1.,-1.77018771687692));
#36004=CARTESIAN_POINT('Ctrl Pts',(0.16803277280837,-1.,-1.78690649988931));
#36005=CARTESIAN_POINT('Ctrl Pts',(0.16803277280837,1.,-1.78690649988931));
#36006=CARTESIAN_POINT('Ctrl Pts',(0.169936923908078,-1.,-1.80561530633924));
#36007=CARTESIAN_POINT('Ctrl Pts',(0.169936923908078,1.,-1.80561530633924));
#36008=CARTESIAN_POINT('Ctrl Pts',(0.171554770207306,-1.,-1.82215766815414));
#36009=CARTESIAN_POINT('Ctrl Pts',(0.171554770207306,1.,-1.82215766815414));
#36010=CARTESIAN_POINT('Ctrl Pts',(0.17288944289442,-1.,-1.83658380530747));
#36011=CARTESIAN_POINT('Ctrl Pts',(0.17288944289442,1.,-1.83658380530747));
#36012=CARTESIAN_POINT('Ctrl Pts',(0.173946627589401,-1.,-1.84898113200543));
#36013=CARTESIAN_POINT('Ctrl Pts',(0.173946627589401,1.,-1.84898113200543));
#36014=CARTESIAN_POINT('Ctrl Pts',(0.174735259276856,-1.,-1.85948367089838));
#36015=CARTESIAN_POINT('Ctrl Pts',(0.174735259276856,1.,-1.85948367089838));
#36016=CARTESIAN_POINT('Ctrl Pts',(0.175268337590901,-1.,-1.86828349694972));
#36017=CARTESIAN_POINT('Ctrl Pts',(0.175268337590901,1.,-1.86828349694972));
#36018=CARTESIAN_POINT('Ctrl Pts',(0.175563480746205,-1.,-1.87563767773249));
#36019=CARTESIAN_POINT('Ctrl Pts',(0.175563480746205,1.,-1.87563767773249));
#36020=CARTESIAN_POINT('Ctrl Pts',(0.175644148889271,-1.,-1.88188663144846));
#36021=CARTESIAN_POINT('Ctrl Pts',(0.175644148889271,1.,-1.88188663144846));
#36022=CARTESIAN_POINT('Ctrl Pts',(0.175538155840286,-1.,-1.88742606272818));
#36023=CARTESIAN_POINT('Ctrl Pts',(0.175538155840286,1.,-1.88742606272818));
#36024=CARTESIAN_POINT('Ctrl Pts',(0.175274276190664,-1.,-1.89264630198279));
#36025=CARTESIAN_POINT('Ctrl Pts',(0.175274276190664,1.,-1.89264630198279));
#36026=CARTESIAN_POINT('Ctrl Pts',(0.174879405091277,-1.,-1.89788101117148));
#36027=CARTESIAN_POINT('Ctrl Pts',(0.174879405091277,1.,-1.89788101117148));
#36028=CARTESIAN_POINT('Ctrl Pts',(0.174375518661222,-1.,-1.90335253863003));
#36029=CARTESIAN_POINT('Ctrl Pts',(0.174375518661222,1.,-1.90335253863003));
#36030=CARTESIAN_POINT('Ctrl Pts',(0.173776635257984,-1.,-1.90911693975475));
#36031=CARTESIAN_POINT('Ctrl Pts',(0.173776635257984,1.,-1.90911693975475));
#36032=CARTESIAN_POINT('Ctrl Pts',(0.173090695383619,-1.,-1.91511429159681));
#36033=CARTESIAN_POINT('Ctrl Pts',(0.173090695383619,1.,-1.91511429159681));
#36034=CARTESIAN_POINT('Ctrl Pts',(0.172321621259557,-1.,-1.92122334398034));
#36035=CARTESIAN_POINT('Ctrl Pts',(0.172321621259557,1.,-1.92122334398034));
#36036=CARTESIAN_POINT('Ctrl Pts',(0.17147119153296,-1.,-1.92731093582));
#36037=CARTESIAN_POINT('Ctrl Pts',(0.17147119153296,1.,-1.92731093582));
#36038=CARTESIAN_POINT('Ctrl Pts',(0.170541253116136,-1.,-1.93329183155455));
#36039=CARTESIAN_POINT('Ctrl Pts',(0.170541253116136,1.,-1.93329183155455));
#36040=CARTESIAN_POINT('Ctrl Pts',(0.169534904817425,-1.,-1.93915639211497));
#36041=CARTESIAN_POINT('Ctrl Pts',(0.169534904817425,1.,-1.93915639211497));
#36042=CARTESIAN_POINT('Ctrl Pts',(0.168455741607516,-1.,-1.94493757756879));
#36043=CARTESIAN_POINT('Ctrl Pts',(0.168455741607516,1.,-1.94493757756879));
#36044=CARTESIAN_POINT('Ctrl Pts',(0.167307501784469,-1.,-1.95069027794286));
#36045=CARTESIAN_POINT('Ctrl Pts',(0.167307501784469,1.,-1.95069027794286));
#36046=CARTESIAN_POINT('Ctrl Pts',(0.166093592002833,-1.,-1.95646759718755));
#36047=CARTESIAN_POINT('Ctrl Pts',(0.166093592002833,1.,-1.95646759718755));
#36048=CARTESIAN_POINT('Ctrl Pts',(0.1648165689203,-1.,-1.96229379940174));
#36049=CARTESIAN_POINT('Ctrl Pts',(0.1648165689203,1.,-1.96229379940174));
#36050=CARTESIAN_POINT('Ctrl Pts',(0.16347818545776,-1.,-1.96816512678));
#36051=CARTESIAN_POINT('Ctrl Pts',(0.16347818545776,1.,-1.96816512678));
#36052=CARTESIAN_POINT('Ctrl Pts',(0.162079693556302,-1.,-1.97406280235204));
#36053=CARTESIAN_POINT('Ctrl Pts',(0.162079693556302,1.,-1.97406280235204));
#36054=CARTESIAN_POINT('Ctrl Pts',(0.16062206078461,-1.,-1.97996195437557));
#36055=CARTESIAN_POINT('Ctrl Pts',(0.16062206078461,1.,-1.97996195437557));
#36056=CARTESIAN_POINT('Ctrl Pts',(0.159106226437288,-1.,-1.98584238283279));
#36057=CARTESIAN_POINT('Ctrl Pts',(0.159106226437288,1.,-1.98584238283279));
#36058=CARTESIAN_POINT('Ctrl Pts',(0.157533331459215,-1.,-1.99169810931893));
#36059=CARTESIAN_POINT('Ctrl Pts',(0.157533331459215,1.,-1.99169810931893));
#36060=CARTESIAN_POINT('Ctrl Pts',(0.155904629548774,-1.,-1.99753284771487));
#36061=CARTESIAN_POINT('Ctrl Pts',(0.155904629548774,1.,-1.99753284771487));
#36062=CARTESIAN_POINT('Ctrl Pts',(0.154221403049719,-1.,-2.00335565310539));
#36063=CARTESIAN_POINT('Ctrl Pts',(0.154221403049719,1.,-2.00335565310539));
#36064=CARTESIAN_POINT('Ctrl Pts',(0.152484883621452,-1.,-2.00917680318426));
#36065=CARTESIAN_POINT('Ctrl Pts',(0.152484883621452,1.,-2.00917680318426));
#36066=CARTESIAN_POINT('Ctrl Pts',(0.150696157673084,-1.,-2.01500291940243));
#36067=CARTESIAN_POINT('Ctrl Pts',(0.150696157673084,1.,-2.01500291940243));
#36068=CARTESIAN_POINT('Ctrl Pts',(0.148856124775343,-1.,-2.02083464969897));
#36069=CARTESIAN_POINT('Ctrl Pts',(0.148856124775343,1.,-2.02083464969897));
#36070=CARTESIAN_POINT('Ctrl Pts',(0.146965557332586,-1.,-2.02666926182017));
#36071=CARTESIAN_POINT('Ctrl Pts',(0.146965557332586,1.,-2.02666926182017));
#36072=CARTESIAN_POINT('Ctrl Pts',(0.145025140186058,-1.,-2.03250223739941));
#36073=CARTESIAN_POINT('Ctrl Pts',(0.145025140186058,1.,-2.03250223739941));
#36074=CARTESIAN_POINT('Ctrl Pts',(0.143035515058208,-1.,-2.03832911025913));
#36075=CARTESIAN_POINT('Ctrl Pts',(0.143035515058208,1.,-2.03832911025913));
#36076=CARTESIAN_POINT('Ctrl Pts',(0.140997332152545,-1.,-2.04414757947919));
#36077=CARTESIAN_POINT('Ctrl Pts',(0.140997332152545,1.,-2.04414757947919));
#36078=CARTESIAN_POINT('Ctrl Pts',(0.138911255368966,-1.,-2.04995762001333));
#36079=CARTESIAN_POINT('Ctrl Pts',(0.138911255368966,1.,-2.04995762001333));
#36080=CARTESIAN_POINT('Ctrl Pts',(0.136777941218044,-1.,-2.0557604441427));
#36081=CARTESIAN_POINT('Ctrl Pts',(0.136777941218044,1.,-2.0557604441427));
#36082=CARTESIAN_POINT('Ctrl Pts',(0.134598026192107,-1.,-2.06155781517844));
#36083=CARTESIAN_POINT('Ctrl Pts',(0.134598026192107,1.,-2.06155781517844));
#36084=CARTESIAN_POINT('Ctrl Pts',(0.13237211154771,-1.,-2.06735123910319));
#36085=CARTESIAN_POINT('Ctrl Pts',(0.13237211154771,1.,-2.06735123910319));
#36086=CARTESIAN_POINT('Ctrl Pts',(0.1301007483284,-1.,-2.07314114713047));
#36087=CARTESIAN_POINT('Ctrl Pts',(0.1301007483284,1.,-2.07314114713047));
#36088=CARTESIAN_POINT('Ctrl Pts',(0.127784445276116,-1.,-2.07892715110967));
#36089=CARTESIAN_POINT('Ctrl Pts',(0.127784445276116,1.,-2.07892715110967));
#36090=CARTESIAN_POINT('Ctrl Pts',(0.125423679412058,-1.,-2.08470840653628));
#36091=CARTESIAN_POINT('Ctrl Pts',(0.125423679412058,1.,-2.08470840653628));
#36092=CARTESIAN_POINT('Ctrl Pts',(0.123018905621083,-1.,-2.09048392424826));
#36093=CARTESIAN_POINT('Ctrl Pts',(0.123018905621083,1.,-2.09048392424826));
#36094=CARTESIAN_POINT('Ctrl Pts',(0.120570567965129,-1.,-2.09625292867756));
#36095=CARTESIAN_POINT('Ctrl Pts',(0.120570567965129,1.,-2.09625292867756));
#36096=CARTESIAN_POINT('Ctrl Pts',(0.118079107988368,-1.,-2.10201512132945));
#36097=CARTESIAN_POINT('Ctrl Pts',(0.118079107988368,1.,-2.10201512132945));
#36098=CARTESIAN_POINT('Ctrl Pts',(0.11554495768794,-1.,-2.10777050261359));
#36099=CARTESIAN_POINT('Ctrl Pts',(0.11554495768794,1.,-2.10777050261359));
#36100=CARTESIAN_POINT('Ctrl Pts',(0.112968534419746,-1.,-2.11351924490335));
#36101=CARTESIAN_POINT('Ctrl Pts',(0.112968534419746,1.,-2.11351924490335));
#36102=CARTESIAN_POINT('Ctrl Pts',(0.11035023613502,-1.,-2.11926155590849));
#36103=CARTESIAN_POINT('Ctrl Pts',(0.11035023613502,1.,-2.11926155590849));
#36104=CARTESIAN_POINT('Ctrl Pts',(0.107690435231068,-1.,-2.12499752306927));
#36105=CARTESIAN_POINT('Ctrl Pts',(0.107690435231068,1.,-2.12499752306927));
#36106=CARTESIAN_POINT('Ctrl Pts',(0.104989479152703,-1.,-2.1307270488718));
#36107=CARTESIAN_POINT('Ctrl Pts',(0.104989479152703,1.,-2.1307270488718));
#36108=CARTESIAN_POINT('Ctrl Pts',(0.102247700556064,-1.,-2.13644992667052));
#36109=CARTESIAN_POINT('Ctrl Pts',(0.102247700556064,1.,-2.13644992667052));
#36110=CARTESIAN_POINT('Ctrl Pts',(0.0994654261990743,-1.,-2.14216588395974));
#36111=CARTESIAN_POINT('Ctrl Pts',(0.0994654261990743,1.,-2.14216588395974));
#36112=CARTESIAN_POINT('Ctrl Pts',(0.0966429852305689,-1.,-2.14787463531864));
#36113=CARTESIAN_POINT('Ctrl Pts',(0.0966429852305689,1.,-2.14787463531864));
#36114=CARTESIAN_POINT('Ctrl Pts',(0.0937807218868345,-1.,-2.15357593978377));
#36115=CARTESIAN_POINT('Ctrl Pts',(0.0937807218868345,1.,-2.15357593978377));
#36116=CARTESIAN_POINT('Ctrl Pts',(0.0908789888108266,-1.,-2.15926961544808));
#36117=CARTESIAN_POINT('Ctrl Pts',(0.0908789888108266,1.,-2.15926961544808));
#36118=CARTESIAN_POINT('Ctrl Pts',(0.0879381291387823,-1.,-2.16495552645275));
#36119=CARTESIAN_POINT('Ctrl Pts',(0.0879381291387823,1.,-2.16495552645275));
#36120=CARTESIAN_POINT('Ctrl Pts',(0.0849584620835643,-1.,-2.17063357871031));
#36121=CARTESIAN_POINT('Ctrl Pts',(0.0849584620835643,1.,-2.17063357871031));
#36122=CARTESIAN_POINT('Ctrl Pts',(0.0819402680871939,-1.,-2.1763037121106));
#36123=CARTESIAN_POINT('Ctrl Pts',(0.0819402680871939,1.,-2.1763037121106));
#36124=CARTESIAN_POINT('Ctrl Pts',(0.0788837727683228,-1.,-2.18196589448304));
#36125=CARTESIAN_POINT('Ctrl Pts',(0.0788837727683228,1.,-2.18196589448304));
#36126=CARTESIAN_POINT('Ctrl Pts',(0.0757891465833411,-1.,-2.1876201139874));
#36127=CARTESIAN_POINT('Ctrl Pts',(0.0757891465833411,1.,-2.1876201139874));
#36128=CARTESIAN_POINT('Ctrl Pts',(0.0732830357304276,-1.,-2.19213712012956));
#36129=CARTESIAN_POINT('Ctrl Pts',(0.0732830357304276,1.,-2.19213712012956));
#36130=CARTESIAN_POINT('Ctrl Pts',(0.0713863779524627,-1.,-2.19552129483562));
#36131=CARTESIAN_POINT('Ctrl Pts',(0.0713863779524627,1.,-2.19552129483562));
#36132=CARTESIAN_POINT('Ctrl Pts',(0.0701143536324926,-1.,-2.19777582085261));
#36133=CARTESIAN_POINT('Ctrl Pts',(0.0701143536324926,1.,-2.19777582085261));
#36134=CARTESIAN_POINT('Ctrl Pts',(0.0694764450219584,-1.,-2.19890268624765));
#36135=CARTESIAN_POINT('Ctrl Pts',(0.0694764450219584,1.,-2.19890268624765));
#36136=CARTESIAN_POINT('',(0.163289472382896,1.,-1.74236521665491));
#36137=CARTESIAN_POINT('Ctrl Pts',(0.163289472382896,1.,-1.74236521665491));
#36138=CARTESIAN_POINT('Ctrl Pts',(0.163814161002474,1.,-1.74720349503904));
#36139=CARTESIAN_POINT('Ctrl Pts',(0.164834765708484,1.,-1.75666056640041));
#36140=CARTESIAN_POINT('Ctrl Pts',(0.166279355148738,1.,-1.77018771687692));
#36141=CARTESIAN_POINT('Ctrl Pts',(0.16803277280837,1.,-1.78690649988931));
#36142=CARTESIAN_POINT('Ctrl Pts',(0.169936923908078,1.,-1.80561530633924));
#36143=CARTESIAN_POINT('Ctrl Pts',(0.171554770207306,1.,-1.82215766815414));
#36144=CARTESIAN_POINT('Ctrl Pts',(0.17288944289442,1.,-1.83658380530747));
#36145=CARTESIAN_POINT('Ctrl Pts',(0.173946627589401,1.,-1.84898113200543));
#36146=CARTESIAN_POINT('Ctrl Pts',(0.174735259276856,1.,-1.85948367089838));
#36147=CARTESIAN_POINT('Ctrl Pts',(0.175268337590901,1.,-1.86828349694972));
#36148=CARTESIAN_POINT('Ctrl Pts',(0.175563480746205,1.,-1.87563767773249));
#36149=CARTESIAN_POINT('Ctrl Pts',(0.175644148889271,1.,-1.88188663144846));
#36150=CARTESIAN_POINT('Ctrl Pts',(0.175538155840286,1.,-1.88742606272818));
#36151=CARTESIAN_POINT('Ctrl Pts',(0.175274276190664,1.,-1.89264630198279));
#36152=CARTESIAN_POINT('Ctrl Pts',(0.174879405091277,1.,-1.89788101117148));
#36153=CARTESIAN_POINT('Ctrl Pts',(0.174375518661222,1.,-1.90335253863003));
#36154=CARTESIAN_POINT('Ctrl Pts',(0.173776635257984,1.,-1.90911693975475));
#36155=CARTESIAN_POINT('Ctrl Pts',(0.173090695383619,1.,-1.91511429159681));
#36156=CARTESIAN_POINT('Ctrl Pts',(0.172321621259557,1.,-1.92122334398034));
#36157=CARTESIAN_POINT('Ctrl Pts',(0.17147119153296,1.,-1.92731093582));
#36158=CARTESIAN_POINT('Ctrl Pts',(0.170541253116136,1.,-1.93329183155455));
#36159=CARTESIAN_POINT('Ctrl Pts',(0.169534904817425,1.,-1.93915639211497));
#36160=CARTESIAN_POINT('Ctrl Pts',(0.168455741607516,1.,-1.94493757756879));
#36161=CARTESIAN_POINT('Ctrl Pts',(0.167307501784469,1.,-1.95069027794286));
#36162=CARTESIAN_POINT('Ctrl Pts',(0.166093592002833,1.,-1.95646759718755));
#36163=CARTESIAN_POINT('Ctrl Pts',(0.1648165689203,1.,-1.96229379940174));
#36164=CARTESIAN_POINT('Ctrl Pts',(0.16347818545776,1.,-1.96816512678));
#36165=CARTESIAN_POINT('Ctrl Pts',(0.162079693556302,1.,-1.97406280235204));
#36166=CARTESIAN_POINT('Ctrl Pts',(0.16062206078461,1.,-1.97996195437557));
#36167=CARTESIAN_POINT('Ctrl Pts',(0.159106226437288,1.,-1.98584238283279));
#36168=CARTESIAN_POINT('Ctrl Pts',(0.157533331459215,1.,-1.99169810931893));
#36169=CARTESIAN_POINT('Ctrl Pts',(0.155904629548774,1.,-1.99753284771487));
#36170=CARTESIAN_POINT('Ctrl Pts',(0.154221403049719,1.,-2.00335565310539));
#36171=CARTESIAN_POINT('Ctrl Pts',(0.152484883621452,1.,-2.00917680318426));
#36172=CARTESIAN_POINT('Ctrl Pts',(0.150696157673084,1.,-2.01500291940243));
#36173=CARTESIAN_POINT('Ctrl Pts',(0.148856124775343,1.,-2.02083464969897));
#36174=CARTESIAN_POINT('Ctrl Pts',(0.146965557332586,1.,-2.02666926182017));
#36175=CARTESIAN_POINT('Ctrl Pts',(0.145025140186058,1.,-2.03250223739941));
#36176=CARTESIAN_POINT('Ctrl Pts',(0.143035515058208,1.,-2.03832911025913));
#36177=CARTESIAN_POINT('Ctrl Pts',(0.140997332152545,1.,-2.04414757947919));
#36178=CARTESIAN_POINT('Ctrl Pts',(0.138911255368966,1.,-2.04995762001333));
#36179=CARTESIAN_POINT('Ctrl Pts',(0.136777941218044,1.,-2.0557604441427));
#36180=CARTESIAN_POINT('Ctrl Pts',(0.134598026192107,1.,-2.06155781517844));
#36181=CARTESIAN_POINT('Ctrl Pts',(0.13237211154771,1.,-2.06735123910319));
#36182=CARTESIAN_POINT('Ctrl Pts',(0.1301007483284,1.,-2.07314114713047));
#36183=CARTESIAN_POINT('Ctrl Pts',(0.127784445276116,1.,-2.07892715110967));
#36184=CARTESIAN_POINT('Ctrl Pts',(0.125423679412058,1.,-2.08470840653628));
#36185=CARTESIAN_POINT('Ctrl Pts',(0.123018905621083,1.,-2.09048392424826));
#36186=CARTESIAN_POINT('Ctrl Pts',(0.120570567965129,1.,-2.09625292867756));
#36187=CARTESIAN_POINT('Ctrl Pts',(0.118079107988368,1.,-2.10201512132945));
#36188=CARTESIAN_POINT('Ctrl Pts',(0.11554495768794,1.,-2.10777050261359));
#36189=CARTESIAN_POINT('Ctrl Pts',(0.112968534419746,1.,-2.11351924490335));
#36190=CARTESIAN_POINT('Ctrl Pts',(0.11035023613502,1.,-2.11926155590849));
#36191=CARTESIAN_POINT('Ctrl Pts',(0.107690435231068,1.,-2.12499752306927));
#36192=CARTESIAN_POINT('Ctrl Pts',(0.104989479152703,1.,-2.1307270488718));
#36193=CARTESIAN_POINT('Ctrl Pts',(0.102247700556064,1.,-2.13644992667052));
#36194=CARTESIAN_POINT('Ctrl Pts',(0.0994654261990743,1.,-2.14216588395974));
#36195=CARTESIAN_POINT('Ctrl Pts',(0.0966429852305689,1.,-2.14787463531864));
#36196=CARTESIAN_POINT('Ctrl Pts',(0.0937807218868345,1.,-2.15357593978377));
#36197=CARTESIAN_POINT('Ctrl Pts',(0.0908789888108266,1.,-2.15926961544808));
#36198=CARTESIAN_POINT('Ctrl Pts',(0.0879381291387823,1.,-2.16495552645275));
#36199=CARTESIAN_POINT('Ctrl Pts',(0.0849584620835643,1.,-2.17063357871031));
#36200=CARTESIAN_POINT('Ctrl Pts',(0.0819402680871939,1.,-2.1763037121106));
#36201=CARTESIAN_POINT('Ctrl Pts',(0.0788837727683228,1.,-2.18196589448304));
#36202=CARTESIAN_POINT('Ctrl Pts',(0.0757891465833411,1.,-2.1876201139874));
#36203=CARTESIAN_POINT('Ctrl Pts',(0.0732830357304276,1.,-2.19213712012956));
#36204=CARTESIAN_POINT('Ctrl Pts',(0.0713863779524627,1.,-2.19552129483562));
#36205=CARTESIAN_POINT('Ctrl Pts',(0.0701143536324926,1.,-2.19777582085261));
#36206=CARTESIAN_POINT('Ctrl Pts',(0.0694764450219584,1.,-2.19890268624765));
#36207=CARTESIAN_POINT('',(0.163289472382896,0.,-1.74236521665491));
#36208=CARTESIAN_POINT('Origin',(0.,0.,0.));
#36209=CARTESIAN_POINT('',(0.383122945602004,1.,-1.7075470150345));
#36210=CARTESIAN_POINT('Origin',(0.,1.,0.));
#36211=CARTESIAN_POINT('',(0.383122945602004,0.,-1.7075470150345));
#36212=CARTESIAN_POINT('Ctrl Pts',(0.61342227326009,-1.,-2.11275013067528));
#36213=CARTESIAN_POINT('Ctrl Pts',(0.61342227326009,1.,-2.11275013067528));
#36214=CARTESIAN_POINT('Ctrl Pts',(0.61246736556225,-1.,-2.11187554260142));
#36215=CARTESIAN_POINT('Ctrl Pts',(0.61246736556225,1.,-2.11187554260142));
#36216=CARTESIAN_POINT('Ctrl Pts',(0.610560911691113,-1.,-2.11012443807661));
#36217=CARTESIAN_POINT('Ctrl Pts',(0.610560911691113,1.,-2.11012443807661));
#36218=CARTESIAN_POINT('Ctrl Pts',(0.607711315456826,-1.,-2.10749199615859));
#36219=CARTESIAN_POINT('Ctrl Pts',(0.607711315456826,1.,-2.10749199615859));
#36220=CARTESIAN_POINT('Ctrl Pts',(0.603932030738212,-1.,-2.10397049887709));
#36221=CARTESIAN_POINT('Ctrl Pts',(0.603932030738212,1.,-2.10397049887709));
#36222=CARTESIAN_POINT('Ctrl Pts',(0.599241616422144,-1.,-2.09954930865331));
#36223=CARTESIAN_POINT('Ctrl Pts',(0.599241616422144,1.,-2.09954930865331));
#36224=CARTESIAN_POINT('Ctrl Pts',(0.594585006052823,-1.,-2.09510876220501));
#36225=CARTESIAN_POINT('Ctrl Pts',(0.594585006052823,1.,-2.09510876220501));
#36226=CARTESIAN_POINT('Ctrl Pts',(0.589962365403189,-1.,-2.09064881812053));
#36227=CARTESIAN_POINT('Ctrl Pts',(0.589962365403189,1.,-2.09064881812053));
#36228=CARTESIAN_POINT('Ctrl Pts',(0.585373918990895,-1.,-2.086169437277));
#36229=CARTESIAN_POINT('Ctrl Pts',(0.585373918990895,1.,-2.086169437277));
#36230=CARTESIAN_POINT('Ctrl Pts',(0.580819952107256,-1.,-2.08167059018138));
#36231=CARTESIAN_POINT('Ctrl Pts',(0.580819952107256,1.,-2.08167059018138));
#36232=CARTESIAN_POINT('Ctrl Pts',(0.576300797416274,-1.,-2.07715226767361));
#36233=CARTESIAN_POINT('Ctrl Pts',(0.576300797416274,1.,-2.07715226767361));
#36234=CARTESIAN_POINT('Ctrl Pts',(0.571816823242411,-1.,-2.07261449292758));
#36235=CARTESIAN_POINT('Ctrl Pts',(0.571816823242411,1.,-2.07261449292758));
#36236=CARTESIAN_POINT('Ctrl Pts',(0.567368421181229,-1.,-2.06805732997383));
#36237=CARTESIAN_POINT('Ctrl Pts',(0.567368421181229,1.,-2.06805732997383));
#36238=CARTESIAN_POINT('Ctrl Pts',(0.562955993082574,-1.,-2.06348090160697));
#36239=CARTESIAN_POINT('Ctrl Pts',(0.562955993082574,1.,-2.06348090160697));
#36240=CARTESIAN_POINT('Ctrl Pts',(0.558579940185467,-1.,-2.05888537756571));
#36241=CARTESIAN_POINT('Ctrl Pts',(0.558579940185467,1.,-2.05888537756571));
#36242=CARTESIAN_POINT('Ctrl Pts',(0.554240657464109,-1.,-2.05427091604482));
#36243=CARTESIAN_POINT('Ctrl Pts',(0.554240657464109,1.,-2.05427091604482));
#36244=CARTESIAN_POINT('Ctrl Pts',(0.549938525150342,-1.,-2.04963761077974));
#36245=CARTESIAN_POINT('Ctrl Pts',(0.549938525150342,1.,-2.04963761077974));
#36246=CARTESIAN_POINT('Ctrl Pts',(0.545673903817348,-1.,-2.0449854471456));
#36247=CARTESIAN_POINT('Ctrl Pts',(0.545673903817348,1.,-2.0449854471456));
#36248=CARTESIAN_POINT('Ctrl Pts',(0.54144712061552,-1.,-2.0403142269048));
#36249=CARTESIAN_POINT('Ctrl Pts',(0.54144712061552,1.,-2.0403142269048));
#36250=CARTESIAN_POINT('Ctrl Pts',(0.537258489833134,-1.,-2.03562362953993));
#36251=CARTESIAN_POINT('Ctrl Pts',(0.537258489833134,1.,-2.03562362953993));
#36252=CARTESIAN_POINT('Ctrl Pts',(0.533108355132905,-1.,-2.03091336214401));
#36253=CARTESIAN_POINT('Ctrl Pts',(0.533108355132905,1.,-2.03091336214401));
#36254=CARTESIAN_POINT('Ctrl Pts',(0.52899712724191,-1.,-2.02618329083289));
#36255=CARTESIAN_POINT('Ctrl Pts',(0.52899712724191,1.,-2.02618329083289));
#36256=CARTESIAN_POINT('Ctrl Pts',(0.524925318333518,-1.,-2.02143356304712));
#36257=CARTESIAN_POINT('Ctrl Pts',(0.524925318333518,1.,-2.02143356304712));
#36258=CARTESIAN_POINT('Ctrl Pts',(0.520893590399428,-1.,-2.01666477917306));
#36259=CARTESIAN_POINT('Ctrl Pts',(0.520893590399428,1.,-2.01666477917306));
#36260=CARTESIAN_POINT('Ctrl Pts',(0.516902681728733,-1.,-2.01187773939257));
#36261=CARTESIAN_POINT('Ctrl Pts',(0.516902681728733,1.,-2.01187773939257));
#36262=CARTESIAN_POINT('Ctrl Pts',(0.512953306961813,-1.,-2.00707309946955));
#36263=CARTESIAN_POINT('Ctrl Pts',(0.512953306961813,1.,-2.00707309946955));
#36264=CARTESIAN_POINT('Ctrl Pts',(0.509046069886152,-1.,-2.00225107134733));
#36265=CARTESIAN_POINT('Ctrl Pts',(0.509046069886152,1.,-2.00225107134733));
#36266=CARTESIAN_POINT('Ctrl Pts',(0.505181361323011,-1.,-1.99741107463567));
#36267=CARTESIAN_POINT('Ctrl Pts',(0.505181361323011,1.,-1.99741107463567));
#36268=CARTESIAN_POINT('Ctrl Pts',(0.501359287727129,-1.,-1.9925514912615));
#36269=CARTESIAN_POINT('Ctrl Pts',(0.501359287727129,1.,-1.9925514912615));
#36270=CARTESIAN_POINT('Ctrl Pts',(0.497579909545564,-1.,-1.98767044752929));
#36271=CARTESIAN_POINT('Ctrl Pts',(0.497579909545564,1.,-1.98767044752929));
#36272=CARTESIAN_POINT('Ctrl Pts',(0.493843476541492,-1.,-1.9827665876182));
#36273=CARTESIAN_POINT('Ctrl Pts',(0.493843476541492,1.,-1.9827665876182));
#36274=CARTESIAN_POINT('Ctrl Pts',(0.490150627860955,-1.,-1.97783973019229));
#36275=CARTESIAN_POINT('Ctrl Pts',(0.490150627860955,1.,-1.97783973019229));
#36276=CARTESIAN_POINT('Ctrl Pts',(0.486502692907661,-1.,-1.97289186263272));
#36277=CARTESIAN_POINT('Ctrl Pts',(0.486502692907661,1.,-1.97289186263272));
#36278=CARTESIAN_POINT('Ctrl Pts',(0.482901662120686,-1.,-1.96792703422358));
#36279=CARTESIAN_POINT('Ctrl Pts',(0.482901662120686,1.,-1.96792703422358));
#36280=CARTESIAN_POINT('Ctrl Pts',(0.479349583074846,-1.,-1.96294933055938));
#36281=CARTESIAN_POINT('Ctrl Pts',(0.479349583074846,1.,-1.96294933055938));
#36282=CARTESIAN_POINT('Ctrl Pts',(0.475848034683171,-1.,-1.95796111148175));
#36283=CARTESIAN_POINT('Ctrl Pts',(0.475848034683171,1.,-1.95796111148175));
#36284=CARTESIAN_POINT('Ctrl Pts',(0.472397672264079,-1.,-1.95296148278136));
#36285=CARTESIAN_POINT('Ctrl Pts',(0.472397672264079,1.,-1.95296148278136));
#36286=CARTESIAN_POINT('Ctrl Pts',(0.468997482913158,-1.,-1.94794381136524));
#36287=CARTESIAN_POINT('Ctrl Pts',(0.468997482913158,1.,-1.94794381136524));
#36288=CARTESIAN_POINT('Ctrl Pts',(0.465645462026064,-1.,-1.94289794196205));
#36289=CARTESIAN_POINT('Ctrl Pts',(0.465645462026064,1.,-1.94289794196205));
#36290=CARTESIAN_POINT('Ctrl Pts',(0.462340031009087,-1.,-1.93781486640834));
#36291=CARTESIAN_POINT('Ctrl Pts',(0.462340031009087,1.,-1.93781486640834));
#36292=CARTESIAN_POINT('Ctrl Pts',(0.459081234547931,-1.,-1.93269066517936));
#36293=CARTESIAN_POINT('Ctrl Pts',(0.459081234547931,1.,-1.93269066517936));
#36294=CARTESIAN_POINT('Ctrl Pts',(0.455872005174335,-1.,-1.92753067150461));
#36295=CARTESIAN_POINT('Ctrl Pts',(0.455872005174335,1.,-1.92753067150461));
#36296=CARTESIAN_POINT('Ctrl Pts',(0.452719478359356,-1.,-1.9223538064847));
#36297=CARTESIAN_POINT('Ctrl Pts',(0.452719478359356,1.,-1.9223538064847));
#36298=CARTESIAN_POINT('Ctrl Pts',(0.449632260106572,-1.,-1.91718342555717));
#36299=CARTESIAN_POINT('Ctrl Pts',(0.449632260106572,1.,-1.91718342555717));
#36300=CARTESIAN_POINT('Ctrl Pts',(0.446617343485651,-1.,-1.91203699981095));
#36301=CARTESIAN_POINT('Ctrl Pts',(0.446617343485651,1.,-1.91203699981095));
#36302=CARTESIAN_POINT('Ctrl Pts',(0.44367755684917,-1.,-1.90691756144906));
#36303=CARTESIAN_POINT('Ctrl Pts',(0.44367755684917,1.,-1.90691756144906));
#36304=CARTESIAN_POINT('Ctrl Pts',(0.44080783370416,-1.,-1.90180124389137));
#36305=CARTESIAN_POINT('Ctrl Pts',(0.44080783370416,1.,-1.90180124389137));
#36306=CARTESIAN_POINT('Ctrl Pts',(0.437995003948443,-1.,-1.89663648956549));
#36307=CARTESIAN_POINT('Ctrl Pts',(0.437995003948443,1.,-1.89663648956549));
#36308=CARTESIAN_POINT('Ctrl Pts',(0.43522566096358,-1.,-1.89136993975585));
#36309=CARTESIAN_POINT('Ctrl Pts',(0.43522566096358,1.,-1.89136993975585));
#36310=CARTESIAN_POINT('Ctrl Pts',(0.432493038548833,-1.,-1.88596913666828));
#36311=CARTESIAN_POINT('Ctrl Pts',(0.432493038548833,1.,-1.88596913666828));
#36312=CARTESIAN_POINT('Ctrl Pts',(0.429803062482217,-1.,-1.88044229001779));
#36313=CARTESIAN_POINT('Ctrl Pts',(0.429803062482217,1.,-1.88044229001779));
#36314=CARTESIAN_POINT('Ctrl Pts',(0.427183828518743,-1.,-1.87486989291334));
#36315=CARTESIAN_POINT('Ctrl Pts',(0.427183828518743,1.,-1.87486989291334));
#36316=CARTESIAN_POINT('Ctrl Pts',(0.424678177290876,-1.,-1.8693780394412));
#36317=CARTESIAN_POINT('Ctrl Pts',(0.424678177290876,1.,-1.8693780394412));
#36318=CARTESIAN_POINT('Ctrl Pts',(0.422327307417884,-1.,-1.86408083333863));
#36319=CARTESIAN_POINT('Ctrl Pts',(0.422327307417884,1.,-1.86408083333863));
#36320=CARTESIAN_POINT('Ctrl Pts',(0.420157287975583,-1.,-1.8590328109667));
#36321=CARTESIAN_POINT('Ctrl Pts',(0.420157287975583,1.,-1.8590328109667));
#36322=CARTESIAN_POINT('Ctrl Pts',(0.418164129144045,-1.,-1.8541763285645));
#36323=CARTESIAN_POINT('Ctrl Pts',(0.418164129144045,1.,-1.8541763285645));
#36324=CARTESIAN_POINT('Ctrl Pts',(0.416300022039885,-1.,-1.84929312930314));
#36325=CARTESIAN_POINT('Ctrl Pts',(0.416300022039885,1.,-1.84929312930314));
#36326=CARTESIAN_POINT('Ctrl Pts',(0.414487438255542,-1.,-1.84405757074218));
#36327=CARTESIAN_POINT('Ctrl Pts',(0.414487438255542,1.,-1.84405757074218));
#36328=CARTESIAN_POINT('Ctrl Pts',(0.412633125322945,-1.,-1.8380895347617));
#36329=CARTESIAN_POINT('Ctrl Pts',(0.412633125322945,1.,-1.8380895347617));
#36330=CARTESIAN_POINT('Ctrl Pts',(0.410641256301276,-1.,-1.83100408895047));
#36331=CARTESIAN_POINT('Ctrl Pts',(0.410641256301276,1.,-1.83100408895047));
#36332=CARTESIAN_POINT('Ctrl Pts',(0.408428948106227,-1.,-1.82247022677562));
#36333=CARTESIAN_POINT('Ctrl Pts',(0.408428948106227,1.,-1.82247022677562));
#36334=CARTESIAN_POINT('Ctrl Pts',(0.405933518407175,-1.,-1.81223801812013));
#36335=CARTESIAN_POINT('Ctrl Pts',(0.405933518407175,1.,-1.81223801812013));
#36336=CARTESIAN_POINT('Ctrl Pts',(0.403107976163396,-1.,-1.80012077173238));
#36337=CARTESIAN_POINT('Ctrl Pts',(0.403107976163396,1.,-1.80012077173238));
#36338=CARTESIAN_POINT('Ctrl Pts',(0.399919403774155,-1.,-1.78598826343754));
#36339=CARTESIAN_POINT('Ctrl Pts',(0.399919403774155,1.,-1.78598826343754));
#36340=CARTESIAN_POINT('Ctrl Pts',(0.396346196110688,-1.,-1.76975560043442));
#36341=CARTESIAN_POINT('Ctrl Pts',(0.396346196110688,1.,-1.76975560043442));
#36342=CARTESIAN_POINT('Ctrl Pts',(0.392375812285395,-1.,-1.75137405310193));
#36343=CARTESIAN_POINT('Ctrl Pts',(0.392375812285395,1.,-1.75137405310193));
#36344=CARTESIAN_POINT('Ctrl Pts',(0.388877023502615,-1.,-1.73493170972829));
#36345=CARTESIAN_POINT('Ctrl Pts',(0.388877023502615,1.,-1.73493170972829));
#36346=CARTESIAN_POINT('Ctrl Pts',(0.386070790323281,-1.,-1.72162022244582));
#36347=CARTESIAN_POINT('Ctrl Pts',(0.386070790323281,1.,-1.72162022244582));
#36348=CARTESIAN_POINT('Ctrl Pts',(0.384119047314215,-1.,-1.71231062891398));
#36349=CARTESIAN_POINT('Ctrl Pts',(0.384119047314215,1.,-1.71231062891398));
#36350=CARTESIAN_POINT('Ctrl Pts',(0.383122945602004,-1.,-1.7075470150345));
#36351=CARTESIAN_POINT('Ctrl Pts',(0.383122945602004,1.,-1.7075470150345));
#36352=CARTESIAN_POINT('',(0.61342227326009,1.,-2.11275013067528));
#36353=CARTESIAN_POINT('Ctrl Pts',(0.61342227326009,1.,-2.11275013067528));
#36354=CARTESIAN_POINT('Ctrl Pts',(0.61246736556225,1.,-2.11187554260142));
#36355=CARTESIAN_POINT('Ctrl Pts',(0.610560911691113,1.,-2.11012443807661));
#36356=CARTESIAN_POINT('Ctrl Pts',(0.607711315456826,1.,-2.10749199615859));
#36357=CARTESIAN_POINT('Ctrl Pts',(0.603932030738212,1.,-2.10397049887709));
#36358=CARTESIAN_POINT('Ctrl Pts',(0.599241616422144,1.,-2.09954930865331));
#36359=CARTESIAN_POINT('Ctrl Pts',(0.594585006052823,1.,-2.09510876220501));
#36360=CARTESIAN_POINT('Ctrl Pts',(0.589962365403189,1.,-2.09064881812053));
#36361=CARTESIAN_POINT('Ctrl Pts',(0.585373918990895,1.,-2.086169437277));
#36362=CARTESIAN_POINT('Ctrl Pts',(0.580819952107256,1.,-2.08167059018138));
#36363=CARTESIAN_POINT('Ctrl Pts',(0.576300797416274,1.,-2.07715226767361));
#36364=CARTESIAN_POINT('Ctrl Pts',(0.571816823242411,1.,-2.07261449292758));
#36365=CARTESIAN_POINT('Ctrl Pts',(0.567368421181229,1.,-2.06805732997383));
#36366=CARTESIAN_POINT('Ctrl Pts',(0.562955993082574,1.,-2.06348090160697));
#36367=CARTESIAN_POINT('Ctrl Pts',(0.558579940185467,1.,-2.05888537756571));
#36368=CARTESIAN_POINT('Ctrl Pts',(0.554240657464109,1.,-2.05427091604482));
#36369=CARTESIAN_POINT('Ctrl Pts',(0.549938525150342,1.,-2.04963761077974));
#36370=CARTESIAN_POINT('Ctrl Pts',(0.545673903817348,1.,-2.0449854471456));
#36371=CARTESIAN_POINT('Ctrl Pts',(0.54144712061552,1.,-2.0403142269048));
#36372=CARTESIAN_POINT('Ctrl Pts',(0.537258489833134,1.,-2.03562362953993));
#36373=CARTESIAN_POINT('Ctrl Pts',(0.533108355132905,1.,-2.03091336214401));
#36374=CARTESIAN_POINT('Ctrl Pts',(0.52899712724191,1.,-2.02618329083289));
#36375=CARTESIAN_POINT('Ctrl Pts',(0.524925318333518,1.,-2.02143356304712));
#36376=CARTESIAN_POINT('Ctrl Pts',(0.520893590399428,1.,-2.01666477917306));
#36377=CARTESIAN_POINT('Ctrl Pts',(0.516902681728733,1.,-2.01187773939257));
#36378=CARTESIAN_POINT('Ctrl Pts',(0.512953306961813,1.,-2.00707309946955));
#36379=CARTESIAN_POINT('Ctrl Pts',(0.509046069886152,1.,-2.00225107134733));
#36380=CARTESIAN_POINT('Ctrl Pts',(0.505181361323011,1.,-1.99741107463567));
#36381=CARTESIAN_POINT('Ctrl Pts',(0.501359287727129,1.,-1.9925514912615));
#36382=CARTESIAN_POINT('Ctrl Pts',(0.497579909545564,1.,-1.98767044752929));
#36383=CARTESIAN_POINT('Ctrl Pts',(0.493843476541492,1.,-1.9827665876182));
#36384=CARTESIAN_POINT('Ctrl Pts',(0.490150627860955,1.,-1.97783973019229));
#36385=CARTESIAN_POINT('Ctrl Pts',(0.486502692907661,1.,-1.97289186263272));
#36386=CARTESIAN_POINT('Ctrl Pts',(0.482901662120686,1.,-1.96792703422358));
#36387=CARTESIAN_POINT('Ctrl Pts',(0.479349583074846,1.,-1.96294933055938));
#36388=CARTESIAN_POINT('Ctrl Pts',(0.475848034683171,1.,-1.95796111148175));
#36389=CARTESIAN_POINT('Ctrl Pts',(0.472397672264079,1.,-1.95296148278136));
#36390=CARTESIAN_POINT('Ctrl Pts',(0.468997482913158,1.,-1.94794381136524));
#36391=CARTESIAN_POINT('Ctrl Pts',(0.465645462026064,1.,-1.94289794196205));
#36392=CARTESIAN_POINT('Ctrl Pts',(0.462340031009087,1.,-1.93781486640834));
#36393=CARTESIAN_POINT('Ctrl Pts',(0.459081234547931,1.,-1.93269066517936));
#36394=CARTESIAN_POINT('Ctrl Pts',(0.455872005174335,1.,-1.92753067150461));
#36395=CARTESIAN_POINT('Ctrl Pts',(0.452719478359356,1.,-1.9223538064847));
#36396=CARTESIAN_POINT('Ctrl Pts',(0.449632260106572,1.,-1.91718342555717));
#36397=CARTESIAN_POINT('Ctrl Pts',(0.446617343485651,1.,-1.91203699981095));
#36398=CARTESIAN_POINT('Ctrl Pts',(0.44367755684917,1.,-1.90691756144906));
#36399=CARTESIAN_POINT('Ctrl Pts',(0.44080783370416,1.,-1.90180124389137));
#36400=CARTESIAN_POINT('Ctrl Pts',(0.437995003948443,1.,-1.89663648956549));
#36401=CARTESIAN_POINT('Ctrl Pts',(0.43522566096358,1.,-1.89136993975585));
#36402=CARTESIAN_POINT('Ctrl Pts',(0.432493038548833,1.,-1.88596913666828));
#36403=CARTESIAN_POINT('Ctrl Pts',(0.429803062482217,1.,-1.88044229001779));
#36404=CARTESIAN_POINT('Ctrl Pts',(0.427183828518743,1.,-1.87486989291334));
#36405=CARTESIAN_POINT('Ctrl Pts',(0.424678177290876,1.,-1.8693780394412));
#36406=CARTESIAN_POINT('Ctrl Pts',(0.422327307417884,1.,-1.86408083333863));
#36407=CARTESIAN_POINT('Ctrl Pts',(0.420157287975583,1.,-1.8590328109667));
#36408=CARTESIAN_POINT('Ctrl Pts',(0.418164129144045,1.,-1.8541763285645));
#36409=CARTESIAN_POINT('Ctrl Pts',(0.416300022039885,1.,-1.84929312930314));
#36410=CARTESIAN_POINT('Ctrl Pts',(0.414487438255542,1.,-1.84405757074218));
#36411=CARTESIAN_POINT('Ctrl Pts',(0.412633125322945,1.,-1.8380895347617));
#36412=CARTESIAN_POINT('Ctrl Pts',(0.410641256301276,1.,-1.83100408895047));
#36413=CARTESIAN_POINT('Ctrl Pts',(0.408428948106227,1.,-1.82247022677562));
#36414=CARTESIAN_POINT('Ctrl Pts',(0.405933518407175,1.,-1.81223801812013));
#36415=CARTESIAN_POINT('Ctrl Pts',(0.403107976163396,1.,-1.80012077173238));
#36416=CARTESIAN_POINT('Ctrl Pts',(0.399919403774155,1.,-1.78598826343754));
#36417=CARTESIAN_POINT('Ctrl Pts',(0.396346196110688,1.,-1.76975560043442));
#36418=CARTESIAN_POINT('Ctrl Pts',(0.392375812285395,1.,-1.75137405310193));
#36419=CARTESIAN_POINT('Ctrl Pts',(0.388877023502615,1.,-1.73493170972829));
#36420=CARTESIAN_POINT('Ctrl Pts',(0.386070790323281,1.,-1.72162022244582));
#36421=CARTESIAN_POINT('Ctrl Pts',(0.384119047314215,1.,-1.71231062891398));
#36422=CARTESIAN_POINT('Ctrl Pts',(0.383122945602004,1.,-1.7075470150345));
#36423=CARTESIAN_POINT('',(0.61342227326009,0.,-2.11275013067528));
#36424=CARTESIAN_POINT('Origin',(0.745574324794401,0.,-2.0698113262342));
#36425=CARTESIAN_POINT('',(0.745574324794401,1.,-2.0698113262342));
#36426=CARTESIAN_POINT('',(0.61342227326009,1.,-2.11275013067528));
#36427=CARTESIAN_POINT('',(0.745574324794401,0.,-2.0698113262342));
#36428=CARTESIAN_POINT('Ctrl Pts',(0.693717979106306,-1.,-1.60662857109684));
#36429=CARTESIAN_POINT('Ctrl Pts',(0.693717979106306,1.,-1.60662857109684));
#36430=CARTESIAN_POINT('Ctrl Pts',(0.695712097881194,-1.,-1.61106790958151));
#36431=CARTESIAN_POINT('Ctrl Pts',(0.695712097881194,1.,-1.61106790958151));
#36432=CARTESIAN_POINT('Ctrl Pts',(0.699605146405088,-1.,-1.61974673472612));
#36433=CARTESIAN_POINT('Ctrl Pts',(0.699605146405088,1.,-1.61974673472612));
#36434=CARTESIAN_POINT('Ctrl Pts',(0.705159151988319,-1.,-1.63216541664676));
#36435=CARTESIAN_POINT('Ctrl Pts',(0.705159151988319,1.,-1.63216541664676));
#36436=CARTESIAN_POINT('Ctrl Pts',(0.711993139355394,-1.,-1.64752408832016));
#36437=CARTESIAN_POINT('Ctrl Pts',(0.711993139355394,1.,-1.64752408832016));
#36438=CARTESIAN_POINT('Ctrl Pts',(0.719585433804282,-1.,-1.6647288055568));
#36439=CARTESIAN_POINT('Ctrl Pts',(0.719585433804282,1.,-1.6647288055568));
#36440=CARTESIAN_POINT('Ctrl Pts',(0.726235967997433,-1.,-1.67996158455503));
#36441=CARTESIAN_POINT('Ctrl Pts',(0.726235967997433,1.,-1.67996158455503));
#36442=CARTESIAN_POINT('Ctrl Pts',(0.731963238697195,-1.,-1.69326921975743));
#36443=CARTESIAN_POINT('Ctrl Pts',(0.731963238697195,1.,-1.69326921975743));
#36444=CARTESIAN_POINT('Ctrl Pts',(0.736799665724771,-1.,-1.70473309006121));
#36445=CARTESIAN_POINT('Ctrl Pts',(0.736799665724771,1.,-1.70473309006121));
#36446=CARTESIAN_POINT('Ctrl Pts',(0.740795162032087,-1.,-1.71447789751927));
#36447=CARTESIAN_POINT('Ctrl Pts',(0.740795162032087,1.,-1.71447789751927));
#36448=CARTESIAN_POINT('Ctrl Pts',(0.744021445433764,-1.,-1.7226822991693));
#36449=CARTESIAN_POINT('Ctrl Pts',(0.744021445433764,1.,-1.7226822991693));
#36450=CARTESIAN_POINT('Ctrl Pts',(0.746574710096436,-1.,-1.72958533647399));
#36451=CARTESIAN_POINT('Ctrl Pts',(0.746574710096436,1.,-1.72958533647399));
#36452=CARTESIAN_POINT('Ctrl Pts',(0.748582462954854,-1.,-1.73550351679848));
#36453=CARTESIAN_POINT('Ctrl Pts',(0.748582462954854,1.,-1.73550351679848));
#36454=CARTESIAN_POINT('Ctrl Pts',(0.75019343597954,-1.,-1.74080458266705));
#36455=CARTESIAN_POINT('Ctrl Pts',(0.75019343597954,1.,-1.74080458266705));
#36456=CARTESIAN_POINT('Ctrl Pts',(0.751555614163629,-1.,-1.74585086852298));
#36457=CARTESIAN_POINT('Ctrl Pts',(0.751555614163629,1.,-1.74585086852298));
#36458=CARTESIAN_POINT('Ctrl Pts',(0.752797683531377,-1.,-1.75095139468809));
#36459=CARTESIAN_POINT('Ctrl Pts',(0.752797683531377,1.,-1.75095139468809));
#36460=CARTESIAN_POINT('Ctrl Pts',(0.75400925402848,-1.,-1.75631083600175));
#36461=CARTESIAN_POINT('Ctrl Pts',(0.75400925402848,1.,-1.75631083600175));
#36462=CARTESIAN_POINT('Ctrl Pts',(0.755220979975262,-1.,-1.7619781724032));
#36463=CARTESIAN_POINT('Ctrl Pts',(0.755220979975262,1.,-1.7619781724032));
#36464=CARTESIAN_POINT('Ctrl Pts',(0.756421896028403,-1.,-1.76789396003141));
#36465=CARTESIAN_POINT('Ctrl Pts',(0.756421896028403,1.,-1.76789396003141));
#36466=CARTESIAN_POINT('Ctrl Pts',(0.757578264077238,-1.,-1.77394167108342));
#36467=CARTESIAN_POINT('Ctrl Pts',(0.757578264077238,1.,-1.77394167108342));
#36468=CARTESIAN_POINT('Ctrl Pts',(0.75865062667738,-1.,-1.77999411220912));
#36469=CARTESIAN_POINT('Ctrl Pts',(0.75865062667738,1.,-1.77999411220912));
#36470=CARTESIAN_POINT('Ctrl Pts',(0.759614401109868,-1.,-1.78596964884527));
#36471=CARTESIAN_POINT('Ctrl Pts',(0.759614401109868,1.,-1.78596964884527));
#36472=CARTESIAN_POINT('Ctrl Pts',(0.760469555880425,-1.,-1.79185815610802));
#36473=CARTESIAN_POINT('Ctrl Pts',(0.760469555880425,1.,-1.79185815610802));
#36474=CARTESIAN_POINT('Ctrl Pts',(0.761229695230359,-1.,-1.79768986997735));
#36475=CARTESIAN_POINT('Ctrl Pts',(0.761229695230359,1.,-1.79768986997735));
#36476=CARTESIAN_POINT('Ctrl Pts',(0.761915336443515,-1.,-1.80351583877334));
#36477=CARTESIAN_POINT('Ctrl Pts',(0.761915336443515,1.,-1.80351583877334));
#36478=CARTESIAN_POINT('Ctrl Pts',(0.762546129464036,-1.,-1.80938551463989));
#36479=CARTESIAN_POINT('Ctrl Pts',(0.762546129464036,1.,-1.80938551463989));
#36480=CARTESIAN_POINT('Ctrl Pts',(0.763132003836783,-1.,-1.81532118405566));
#36481=CARTESIAN_POINT('Ctrl Pts',(0.763132003836783,1.,-1.81532118405566));
#36482=CARTESIAN_POINT('Ctrl Pts',(0.763673465462854,-1.,-1.82131873145297));
#36483=CARTESIAN_POINT('Ctrl Pts',(0.763673465462854,1.,-1.82131873145297));
#36484=CARTESIAN_POINT('Ctrl Pts',(0.764165902606055,-1.,-1.8273599120008));
#36485=CARTESIAN_POINT('Ctrl Pts',(0.764165902606055,1.,-1.8273599120008));
#36486=CARTESIAN_POINT('Ctrl Pts',(0.764602549687845,-1.,-1.8334207722714));
#36487=CARTESIAN_POINT('Ctrl Pts',(0.764602549687845,1.,-1.8334207722714));
#36488=CARTESIAN_POINT('Ctrl Pts',(0.764978057881687,-1.,-1.83948181064823));
#36489=CARTESIAN_POINT('Ctrl Pts',(0.764978057881687,1.,-1.83948181064823));
#36490=CARTESIAN_POINT('Ctrl Pts',(0.765291664861971,-1.,-1.84553698875911));
#36491=CARTESIAN_POINT('Ctrl Pts',(0.765291664861971,1.,-1.84553698875911));
#36492=CARTESIAN_POINT('Ctrl Pts',(0.765545710619023,-1.,-1.85158945130054));
#36493=CARTESIAN_POINT('Ctrl Pts',(0.765545710619023,1.,-1.85158945130054));
#36494=CARTESIAN_POINT('Ctrl Pts',(0.765744212909305,-1.,-1.85764741390391));
#36495=CARTESIAN_POINT('Ctrl Pts',(0.765744212909305,1.,-1.85764741390391));
#36496=CARTESIAN_POINT('Ctrl Pts',(0.765891519092557,-1.,-1.86372027063315));
#36497=CARTESIAN_POINT('Ctrl Pts',(0.765891519092557,1.,-1.86372027063315));
#36498=CARTESIAN_POINT('Ctrl Pts',(0.765990708546111,-1.,-1.86981398314345));
#36499=CARTESIAN_POINT('Ctrl Pts',(0.765990708546111,1.,-1.86981398314345));
#36500=CARTESIAN_POINT('Ctrl Pts',(0.766042837036759,-1.,-1.87592888967886));
#36501=CARTESIAN_POINT('Ctrl Pts',(0.766042837036759,1.,-1.87592888967886));
#36502=CARTESIAN_POINT('Ctrl Pts',(0.766047794851868,-1.,-1.88206215302561));
#36503=CARTESIAN_POINT('Ctrl Pts',(0.766047794851868,1.,-1.88206215302561));
#36504=CARTESIAN_POINT('Ctrl Pts',(0.76600483706209,-1.,-1.88820926433409));
#36505=CARTESIAN_POINT('Ctrl Pts',(0.76600483706209,1.,-1.88820926433409));
#36506=CARTESIAN_POINT('Ctrl Pts',(0.765913193856979,-1.,-1.89436577771389));
#36507=CARTESIAN_POINT('Ctrl Pts',(0.765913193856979,1.,-1.89436577771389));
#36508=CARTESIAN_POINT('Ctrl Pts',(0.765772772593395,-1.,-1.90052930393599));
#36509=CARTESIAN_POINT('Ctrl Pts',(0.765772772593395,1.,-1.90052930393599));
#36510=CARTESIAN_POINT('Ctrl Pts',(0.765584196937936,-1.,-1.90669961402362));
#36511=CARTESIAN_POINT('Ctrl Pts',(0.765584196937936,1.,-1.90669961402362));
#36512=CARTESIAN_POINT('Ctrl Pts',(0.765348465884739,-1.,-1.91287765805174));
#36513=CARTESIAN_POINT('Ctrl Pts',(0.765348465884739,1.,-1.91287765805174));
#36514=CARTESIAN_POINT('Ctrl Pts',(0.765066729667095,-1.,-1.91906491634197));
#36515=CARTESIAN_POINT('Ctrl Pts',(0.765066729667095,1.,-1.91906491634197));
#36516=CARTESIAN_POINT('Ctrl Pts',(0.764740025488189,-1.,-1.92526263537041));
#36517=CARTESIAN_POINT('Ctrl Pts',(0.764740025488189,1.,-1.92526263537041));
#36518=CARTESIAN_POINT('Ctrl Pts',(0.764369010673889,-1.,-1.93147105496367));
#36519=CARTESIAN_POINT('Ctrl Pts',(0.764369010673889,1.,-1.93147105496367));
#36520=CARTESIAN_POINT('Ctrl Pts',(0.763954049121393,-1.,-1.93768964875867));
#36521=CARTESIAN_POINT('Ctrl Pts',(0.763954049121393,1.,-1.93768964875867));
#36522=CARTESIAN_POINT('Ctrl Pts',(0.76349533353858,-1.,-1.94391746617626));
#36523=CARTESIAN_POINT('Ctrl Pts',(0.76349533353858,1.,-1.94391746617626));
#36524=CARTESIAN_POINT('Ctrl Pts',(0.762992990878774,-1.,-1.95015342590025));
#36525=CARTESIAN_POINT('Ctrl Pts',(0.762992990878774,1.,-1.95015342590025));
#36526=CARTESIAN_POINT('Ctrl Pts',(0.762447203806263,-1.,-1.95639665309893));
#36527=CARTESIAN_POINT('Ctrl Pts',(0.762447203806263,1.,-1.95639665309893));
#36528=CARTESIAN_POINT('Ctrl Pts',(0.761858300014575,-1.,-1.96264672744229));
#36529=CARTESIAN_POINT('Ctrl Pts',(0.761858300014575,1.,-1.96264672744229));
#36530=CARTESIAN_POINT('Ctrl Pts',(0.761226690483986,-1.,-1.96890351582545));
#36531=CARTESIAN_POINT('Ctrl Pts',(0.761226690483986,1.,-1.96890351582545));
#36532=CARTESIAN_POINT('Ctrl Pts',(0.760552825409855,-1.,-1.97516705321521));
#36533=CARTESIAN_POINT('Ctrl Pts',(0.760552825409855,1.,-1.97516705321521));
#36534=CARTESIAN_POINT('Ctrl Pts',(0.759837147452135,-1.,-1.98143741418156));
#36535=CARTESIAN_POINT('Ctrl Pts',(0.759837147452135,1.,-1.98143741418156));
#36536=CARTESIAN_POINT('Ctrl Pts',(0.759080037802242,-1.,-1.98771456680806));
#36537=CARTESIAN_POINT('Ctrl Pts',(0.759080037802242,1.,-1.98771456680806));
#36538=CARTESIAN_POINT('Ctrl Pts',(0.758281796766377,-1.,-1.9939983109871));
#36539=CARTESIAN_POINT('Ctrl Pts',(0.758281796766377,1.,-1.9939983109871));
#36540=CARTESIAN_POINT('Ctrl Pts',(0.757442676862341,-1.,-2.00028834739072));
#36541=CARTESIAN_POINT('Ctrl Pts',(0.757442676862341,1.,-2.00028834739072));
#36542=CARTESIAN_POINT('Ctrl Pts',(0.756562904646496,-1.,-2.00658431587682));
#36543=CARTESIAN_POINT('Ctrl Pts',(0.756562904646496,1.,-2.00658431587682));
#36544=CARTESIAN_POINT('Ctrl Pts',(0.7556427049581,-1.,-2.01288584328149));
#36545=CARTESIAN_POINT('Ctrl Pts',(0.7556427049581,1.,-2.01288584328149));
#36546=CARTESIAN_POINT('Ctrl Pts',(0.75468233072352,-1.,-2.01919259406003));
#36547=CARTESIAN_POINT('Ctrl Pts',(0.75468233072352,1.,-2.01919259406003));
#36548=CARTESIAN_POINT('Ctrl Pts',(0.753682061113765,-1.,-2.02550428623587));
#36549=CARTESIAN_POINT('Ctrl Pts',(0.753682061113765,1.,-2.02550428623587));
#36550=CARTESIAN_POINT('Ctrl Pts',(0.752642180488104,-1.,-2.03182068456467));
#36551=CARTESIAN_POINT('Ctrl Pts',(0.752642180488104,1.,-2.03182068456467));
#36552=CARTESIAN_POINT('Ctrl Pts',(0.751562963361383,-1.,-2.03814160092173));
#36553=CARTESIAN_POINT('Ctrl Pts',(0.751562963361383,1.,-2.03814160092173));
#36554=CARTESIAN_POINT('Ctrl Pts',(0.750444657874758,-1.,-2.04446689147754));
#36555=CARTESIAN_POINT('Ctrl Pts',(0.750444657874758,1.,-2.04446689147754));
#36556=CARTESIAN_POINT('Ctrl Pts',(0.749287468663053,-1.,-2.05079645591606));
#36557=CARTESIAN_POINT('Ctrl Pts',(0.749287468663053,1.,-2.05079645591606));
#36558=CARTESIAN_POINT('Ctrl Pts',(0.748091554181101,-1.,-2.05713023030263));
#36559=CARTESIAN_POINT('Ctrl Pts',(0.748091554181101,1.,-2.05713023030263));
#36560=CARTESIAN_POINT('Ctrl Pts',(0.747103932785504,-1.,-2.06220058927162));
#36561=CARTESIAN_POINT('Ctrl Pts',(0.747103932785504,1.,-2.06220058927162));
#36562=CARTESIAN_POINT('Ctrl Pts',(0.746345871542695,-1.,-2.06600523016401));
#36563=CARTESIAN_POINT('Ctrl Pts',(0.746345871542695,1.,-2.06600523016401));
#36564=CARTESIAN_POINT('Ctrl Pts',(0.74583279137781,-1.,-2.06854248895575));
#36565=CARTESIAN_POINT('Ctrl Pts',(0.74583279137781,1.,-2.06854248895575));
#36566=CARTESIAN_POINT('Ctrl Pts',(0.745574324794401,-1.,-2.0698113262342));
#36567=CARTESIAN_POINT('Ctrl Pts',(0.745574324794401,1.,-2.0698113262342));
#36568=CARTESIAN_POINT('',(0.693717979106306,1.,-1.60662857109684));
#36569=CARTESIAN_POINT('Ctrl Pts',(0.693717979106306,1.,-1.60662857109684));
#36570=CARTESIAN_POINT('Ctrl Pts',(0.695712097881194,1.,-1.61106790958151));
#36571=CARTESIAN_POINT('Ctrl Pts',(0.699605146405088,1.,-1.61974673472612));
#36572=CARTESIAN_POINT('Ctrl Pts',(0.705159151988319,1.,-1.63216541664676));
#36573=CARTESIAN_POINT('Ctrl Pts',(0.711993139355394,1.,-1.64752408832016));
#36574=CARTESIAN_POINT('Ctrl Pts',(0.719585433804282,1.,-1.6647288055568));
#36575=CARTESIAN_POINT('Ctrl Pts',(0.726235967997433,1.,-1.67996158455503));
#36576=CARTESIAN_POINT('Ctrl Pts',(0.731963238697195,1.,-1.69326921975743));
#36577=CARTESIAN_POINT('Ctrl Pts',(0.736799665724771,1.,-1.70473309006121));
#36578=CARTESIAN_POINT('Ctrl Pts',(0.740795162032087,1.,-1.71447789751927));
#36579=CARTESIAN_POINT('Ctrl Pts',(0.744021445433764,1.,-1.7226822991693));
#36580=CARTESIAN_POINT('Ctrl Pts',(0.746574710096436,1.,-1.72958533647399));
#36581=CARTESIAN_POINT('Ctrl Pts',(0.748582462954854,1.,-1.73550351679848));
#36582=CARTESIAN_POINT('Ctrl Pts',(0.75019343597954,1.,-1.74080458266705));
#36583=CARTESIAN_POINT('Ctrl Pts',(0.751555614163629,1.,-1.74585086852298));
#36584=CARTESIAN_POINT('Ctrl Pts',(0.752797683531377,1.,-1.75095139468809));
#36585=CARTESIAN_POINT('Ctrl Pts',(0.75400925402848,1.,-1.75631083600175));
#36586=CARTESIAN_POINT('Ctrl Pts',(0.755220979975262,1.,-1.7619781724032));
#36587=CARTESIAN_POINT('Ctrl Pts',(0.756421896028403,1.,-1.76789396003141));
#36588=CARTESIAN_POINT('Ctrl Pts',(0.757578264077238,1.,-1.77394167108342));
#36589=CARTESIAN_POINT('Ctrl Pts',(0.75865062667738,1.,-1.77999411220912));
#36590=CARTESIAN_POINT('Ctrl Pts',(0.759614401109868,1.,-1.78596964884527));
#36591=CARTESIAN_POINT('Ctrl Pts',(0.760469555880425,1.,-1.79185815610802));
#36592=CARTESIAN_POINT('Ctrl Pts',(0.761229695230359,1.,-1.79768986997735));
#36593=CARTESIAN_POINT('Ctrl Pts',(0.761915336443515,1.,-1.80351583877334));
#36594=CARTESIAN_POINT('Ctrl Pts',(0.762546129464036,1.,-1.80938551463989));
#36595=CARTESIAN_POINT('Ctrl Pts',(0.763132003836783,1.,-1.81532118405566));
#36596=CARTESIAN_POINT('Ctrl Pts',(0.763673465462854,1.,-1.82131873145297));
#36597=CARTESIAN_POINT('Ctrl Pts',(0.764165902606055,1.,-1.8273599120008));
#36598=CARTESIAN_POINT('Ctrl Pts',(0.764602549687845,1.,-1.8334207722714));
#36599=CARTESIAN_POINT('Ctrl Pts',(0.764978057881687,1.,-1.83948181064823));
#36600=CARTESIAN_POINT('Ctrl Pts',(0.765291664861971,1.,-1.84553698875911));
#36601=CARTESIAN_POINT('Ctrl Pts',(0.765545710619023,1.,-1.85158945130054));
#36602=CARTESIAN_POINT('Ctrl Pts',(0.765744212909305,1.,-1.85764741390391));
#36603=CARTESIAN_POINT('Ctrl Pts',(0.765891519092557,1.,-1.86372027063315));
#36604=CARTESIAN_POINT('Ctrl Pts',(0.765990708546111,1.,-1.86981398314345));
#36605=CARTESIAN_POINT('Ctrl Pts',(0.766042837036759,1.,-1.87592888967886));
#36606=CARTESIAN_POINT('Ctrl Pts',(0.766047794851868,1.,-1.88206215302561));
#36607=CARTESIAN_POINT('Ctrl Pts',(0.76600483706209,1.,-1.88820926433409));
#36608=CARTESIAN_POINT('Ctrl Pts',(0.765913193856979,1.,-1.89436577771389));
#36609=CARTESIAN_POINT('Ctrl Pts',(0.765772772593395,1.,-1.90052930393599));
#36610=CARTESIAN_POINT('Ctrl Pts',(0.765584196937936,1.,-1.90669961402362));
#36611=CARTESIAN_POINT('Ctrl Pts',(0.765348465884739,1.,-1.91287765805174));
#36612=CARTESIAN_POINT('Ctrl Pts',(0.765066729667095,1.,-1.91906491634197));
#36613=CARTESIAN_POINT('Ctrl Pts',(0.764740025488189,1.,-1.92526263537041));
#36614=CARTESIAN_POINT('Ctrl Pts',(0.764369010673889,1.,-1.93147105496367));
#36615=CARTESIAN_POINT('Ctrl Pts',(0.763954049121393,1.,-1.93768964875867));
#36616=CARTESIAN_POINT('Ctrl Pts',(0.76349533353858,1.,-1.94391746617626));
#36617=CARTESIAN_POINT('Ctrl Pts',(0.762992990878774,1.,-1.95015342590025));
#36618=CARTESIAN_POINT('Ctrl Pts',(0.762447203806263,1.,-1.95639665309893));
#36619=CARTESIAN_POINT('Ctrl Pts',(0.761858300014575,1.,-1.96264672744229));
#36620=CARTESIAN_POINT('Ctrl Pts',(0.761226690483986,1.,-1.96890351582545));
#36621=CARTESIAN_POINT('Ctrl Pts',(0.760552825409855,1.,-1.97516705321521));
#36622=CARTESIAN_POINT('Ctrl Pts',(0.759837147452135,1.,-1.98143741418156));
#36623=CARTESIAN_POINT('Ctrl Pts',(0.759080037802242,1.,-1.98771456680806));
#36624=CARTESIAN_POINT('Ctrl Pts',(0.758281796766377,1.,-1.9939983109871));
#36625=CARTESIAN_POINT('Ctrl Pts',(0.757442676862341,1.,-2.00028834739072));
#36626=CARTESIAN_POINT('Ctrl Pts',(0.756562904646496,1.,-2.00658431587682));
#36627=CARTESIAN_POINT('Ctrl Pts',(0.7556427049581,1.,-2.01288584328149));
#36628=CARTESIAN_POINT('Ctrl Pts',(0.75468233072352,1.,-2.01919259406003));
#36629=CARTESIAN_POINT('Ctrl Pts',(0.753682061113765,1.,-2.02550428623587));
#36630=CARTESIAN_POINT('Ctrl Pts',(0.752642180488104,1.,-2.03182068456467));
#36631=CARTESIAN_POINT('Ctrl Pts',(0.751562963361383,1.,-2.03814160092173));
#36632=CARTESIAN_POINT('Ctrl Pts',(0.750444657874758,1.,-2.04446689147754));
#36633=CARTESIAN_POINT('Ctrl Pts',(0.749287468663053,1.,-2.05079645591606));
#36634=CARTESIAN_POINT('Ctrl Pts',(0.748091554181101,1.,-2.05713023030263));
#36635=CARTESIAN_POINT('Ctrl Pts',(0.747103932785504,1.,-2.06220058927162));
#36636=CARTESIAN_POINT('Ctrl Pts',(0.746345871542695,1.,-2.06600523016401));
#36637=CARTESIAN_POINT('Ctrl Pts',(0.74583279137781,1.,-2.06854248895575));
#36638=CARTESIAN_POINT('Ctrl Pts',(0.745574324794401,1.,-2.0698113262342));
#36639=CARTESIAN_POINT('',(0.693717979106306,0.,-1.60662857109684));
#36640=CARTESIAN_POINT('Origin',(0.,0.,0.));
#36641=CARTESIAN_POINT('',(0.892032620296855,1.,-1.5055822144029));
#36642=CARTESIAN_POINT('Origin',(0.,1.,0.));
#36643=CARTESIAN_POINT('',(0.892032620296855,0.,-1.5055822144029));
#36644=CARTESIAN_POINT('Ctrl Pts',(1.23627494547115,-1.,-1.81978687191668));
#36645=CARTESIAN_POINT('Ctrl Pts',(1.23627494547115,1.,-1.81978687191668));
#36646=CARTESIAN_POINT('Ctrl Pts',(1.23509651170476,-1.,-1.81925017193666));
#36647=CARTESIAN_POINT('Ctrl Pts',(1.23509651170476,1.,-1.81925017193666));
#36648=CARTESIAN_POINT('Ctrl Pts',(1.2327422452705,-1.,-1.81817389921279));
#36649=CARTESIAN_POINT('Ctrl Pts',(1.2327422452705,1.,-1.81817389921279));
#36650=CARTESIAN_POINT('Ctrl Pts',(1.2292186489137,-1.,-1.8165508718364));
#36651=CARTESIAN_POINT('Ctrl Pts',(1.2292186489137,1.,-1.8165508718364));
#36652=CARTESIAN_POINT('Ctrl Pts',(1.2245361330495,-1.,-1.81436959210434));
#36653=CARTESIAN_POINT('Ctrl Pts',(1.2245361330495,1.,-1.81436959210434));
#36654=CARTESIAN_POINT('Ctrl Pts',(1.21870906103557,-1.,-1.81161420806656));
#36655=CARTESIAN_POINT('Ctrl Pts',(1.21870906103557,1.,-1.81161420806656));
#36656=CARTESIAN_POINT('Ctrl Pts',(1.21290815708314,-1.,-1.80882996917129));
#36657=CARTESIAN_POINT('Ctrl Pts',(1.21290815708314,1.,-1.80882996917129));
#36658=CARTESIAN_POINT('Ctrl Pts',(1.20713356605475,-1.,-1.80601678480707));
#36659=CARTESIAN_POINT('Ctrl Pts',(1.20713356605475,1.,-1.80601678480707));
#36660=CARTESIAN_POINT('Ctrl Pts',(1.20138548938974,-1.,-1.80317454838603));
#36661=CARTESIAN_POINT('Ctrl Pts',(1.20138548938974,1.,-1.80317454838603));
#36662=CARTESIAN_POINT('Ctrl Pts',(1.19566418930242,-1.,-1.80030314369879));
#36663=CARTESIAN_POINT('Ctrl Pts',(1.19566418930242,1.,-1.80030314369879));
#36664=CARTESIAN_POINT('Ctrl Pts',(1.18996997934445,-1.,-1.79740245923478));
#36665=CARTESIAN_POINT('Ctrl Pts',(1.18996997934445,1.,-1.79740245923478));
#36666=CARTESIAN_POINT('Ctrl Pts',(1.18430321697432,-1.,-1.79447240321515));
#36667=CARTESIAN_POINT('Ctrl Pts',(1.18430321697432,1.,-1.79447240321515));
#36668=CARTESIAN_POINT('Ctrl Pts',(1.17866429440809,-1.,-1.79151291552689));
#36669=CARTESIAN_POINT('Ctrl Pts',(1.17866429440809,1.,-1.79151291552689));
#36670=CARTESIAN_POINT('Ctrl Pts',(1.17305363177328,-1.,-1.78852398877617));
#36671=CARTESIAN_POINT('Ctrl Pts',(1.17305363177328,1.,-1.78852398877617));
#36672=CARTESIAN_POINT('Ctrl Pts',(1.16747166312303,-1.,-1.78550566040443));
#36673=CARTESIAN_POINT('Ctrl Pts',(1.16747166312303,1.,-1.78550566040443));
#36674=CARTESIAN_POINT('Ctrl Pts',(1.16191881298499,-1.,-1.78245795881009));
#36675=CARTESIAN_POINT('Ctrl Pts',(1.16191881298499,1.,-1.78245795881009));
#36676=CARTESIAN_POINT('Ctrl Pts',(1.15639547194698,-1.,-1.77938085564275));
#36677=CARTESIAN_POINT('Ctrl Pts',(1.15639547194698,1.,-1.77938085564275));
#36678=CARTESIAN_POINT('Ctrl Pts',(1.15090197841514,-1.,-1.7762742255701));
#36679=CARTESIAN_POINT('Ctrl Pts',(1.15090197841514,1.,-1.7762742255701));
#36680=CARTESIAN_POINT('Ctrl Pts',(1.1454385822692,-1.,-1.77313777896194));
#36681=CARTESIAN_POINT('Ctrl Pts',(1.1454385822692,1.,-1.77313777896194));
#36682=CARTESIAN_POINT('Ctrl Pts',(1.14000548336975,-1.,-1.76997111386769));
#36683=CARTESIAN_POINT('Ctrl Pts',(1.14000548336975,1.,-1.76997111386769));
#36684=CARTESIAN_POINT('Ctrl Pts',(1.1346029180462,-1.,-1.76677384551862));
#36685=CARTESIAN_POINT('Ctrl Pts',(1.1346029180462,1.,-1.76677384551862));
#36686=CARTESIAN_POINT('Ctrl Pts',(1.12923123555075,-1.,-1.7635457196617));
#36687=CARTESIAN_POINT('Ctrl Pts',(1.12923123555075,1.,-1.7635457196617));
#36688=CARTESIAN_POINT('Ctrl Pts',(1.12389096855086,-1.,-1.76028671825096));
#36689=CARTESIAN_POINT('Ctrl Pts',(1.12389096855086,1.,-1.76028671825096));
#36690=CARTESIAN_POINT('Ctrl Pts',(1.11858293216763,-1.,-1.75699720772105));
#36691=CARTESIAN_POINT('Ctrl Pts',(1.11858293216763,1.,-1.75699720772105));
#36692=CARTESIAN_POINT('Ctrl Pts',(1.11330807582551,-1.,-1.7536777209463));
#36693=CARTESIAN_POINT('Ctrl Pts',(1.11330807582551,1.,-1.7536777209463));
#36694=CARTESIAN_POINT('Ctrl Pts',(1.10806728183007,-1.,-1.7503286607592));
#36695=CARTESIAN_POINT('Ctrl Pts',(1.10806728183007,1.,-1.7503286607592));
#36696=CARTESIAN_POINT('Ctrl Pts',(1.10286118991143,-1.,-1.74695004214923));
#36697=CARTESIAN_POINT('Ctrl Pts',(1.10286118991143,1.,-1.74695004214923));
#36698=CARTESIAN_POINT('Ctrl Pts',(1.09768999241225,-1.,-1.74354119236208));
#36699=CARTESIAN_POINT('Ctrl Pts',(1.09768999241225,1.,-1.74354119236208));
#36700=CARTESIAN_POINT('Ctrl Pts',(1.09255329056493,-1.,-1.74010053962247));
#36701=CARTESIAN_POINT('Ctrl Pts',(1.09255329056493,1.,-1.74010053962247));
#36702=CARTESIAN_POINT('Ctrl Pts',(1.08745056285427,-1.,-1.73662628326091));
#36703=CARTESIAN_POINT('Ctrl Pts',(1.08745056285427,1.,-1.73662628326091));
#36704=CARTESIAN_POINT('Ctrl Pts',(1.08238162784749,-1.,-1.73311705663407));
#36705=CARTESIAN_POINT('Ctrl Pts',(1.08238162784749,1.,-1.73311705663407));
#36706=CARTESIAN_POINT('Ctrl Pts',(1.0773470373727,-1.,-1.72957248977424));
#36707=CARTESIAN_POINT('Ctrl Pts',(1.0773470373727,1.,-1.72957248977424));
#36708=CARTESIAN_POINT('Ctrl Pts',(1.07234866990252,-1.,-1.72599406198488));
#36709=CARTESIAN_POINT('Ctrl Pts',(1.07234866990252,1.,-1.72599406198488));
#36710=CARTESIAN_POINT('Ctrl Pts',(1.06738966975462,-1.,-1.72238500928453));
#36711=CARTESIAN_POINT('Ctrl Pts',(1.06738966975462,1.,-1.72238500928453));
#36712=CARTESIAN_POINT('Ctrl Pts',(1.06247324680647,-1.,-1.71874858456904));
#36713=CARTESIAN_POINT('Ctrl Pts',(1.06247324680647,1.,-1.71874858456904));
#36714=CARTESIAN_POINT('Ctrl Pts',(1.05760163192479,-1.,-1.7150865442702));
#36715=CARTESIAN_POINT('Ctrl Pts',(1.05760163192479,1.,-1.7150865442702));
#36716=CARTESIAN_POINT('Ctrl Pts',(1.05277517202855,-1.,-1.71139783543989));
#36717=CARTESIAN_POINT('Ctrl Pts',(1.05277517202855,1.,-1.71139783543989));
#36718=CARTESIAN_POINT('Ctrl Pts',(1.04799085404995,-1.,-1.70767646263649));
#36719=CARTESIAN_POINT('Ctrl Pts',(1.04799085404995,1.,-1.70767646263649));
#36720=CARTESIAN_POINT('Ctrl Pts',(1.04324363334554,-1.,-1.70391338707982));
#36721=CARTESIAN_POINT('Ctrl Pts',(1.04324363334554,1.,-1.70391338707982));
#36722=CARTESIAN_POINT('Ctrl Pts',(1.03852922490789,-1.,-1.70010052930962));
#36723=CARTESIAN_POINT('Ctrl Pts',(1.03852922490789,1.,-1.70010052930962));
#36724=CARTESIAN_POINT('Ctrl Pts',(1.03384646003588,-1.,-1.69623414782771));
#36725=CARTESIAN_POINT('Ctrl Pts',(1.03384646003588,1.,-1.69623414782771));
#36726=CARTESIAN_POINT('Ctrl Pts',(1.02919977579147,-1.,-1.69231840863458));
#36727=CARTESIAN_POINT('Ctrl Pts',(1.02919977579147,1.,-1.69231840863458));
#36728=CARTESIAN_POINT('Ctrl Pts',(1.02460180535255,-1.,-1.68836910178447));
#36729=CARTESIAN_POINT('Ctrl Pts',(1.02460180535255,1.,-1.68836910178447));
#36730=CARTESIAN_POINT('Ctrl Pts',(1.02006795074201,-1.,-1.68440578021706));
#36731=CARTESIAN_POINT('Ctrl Pts',(1.02006795074201,1.,-1.68440578021706));
#36732=CARTESIAN_POINT('Ctrl Pts',(1.01561026162773,-1.,-1.68044289894798));
#36733=CARTESIAN_POINT('Ctrl Pts',(1.01561026162773,1.,-1.68044289894798));
#36734=CARTESIAN_POINT('Ctrl Pts',(1.01123236493511,-1.,-1.67648246776464));
#36735=CARTESIAN_POINT('Ctrl Pts',(1.01123236493511,1.,-1.67648246776464));
#36736=CARTESIAN_POINT('Ctrl Pts',(1.00692206696414,-1.,-1.67250335383293));
#36737=CARTESIAN_POINT('Ctrl Pts',(1.00692206696414,1.,-1.67250335383293));
#36738=CARTESIAN_POINT('Ctrl Pts',(1.00265091003727,-1.,-1.66846059277303));
#36739=CARTESIAN_POINT('Ctrl Pts',(1.00265091003727,1.,-1.66846059277303));
#36740=CARTESIAN_POINT('Ctrl Pts',(0.998389654952757,-1.,-1.66430758030376));
#36741=CARTESIAN_POINT('Ctrl Pts',(0.998389654952757,1.,-1.66430758030376));
#36742=CARTESIAN_POINT('Ctrl Pts',(0.994121836661305,-1.,-1.66001553809947));
#36743=CARTESIAN_POINT('Ctrl Pts',(0.994121836661305,1.,-1.66001553809947));
#36744=CARTESIAN_POINT('Ctrl Pts',(0.989855627854164,-1.,-1.65559044289699));
#36745=CARTESIAN_POINT('Ctrl Pts',(0.989855627854164,1.,-1.65559044289699));
#36746=CARTESIAN_POINT('Ctrl Pts',(0.98564262292082,-1.,-1.65110016612638));
#36747=CARTESIAN_POINT('Ctrl Pts',(0.98564262292082,1.,-1.65110016612638));
#36748=CARTESIAN_POINT('Ctrl Pts',(0.981562530939489,-1.,-1.64665139190656));
#36749=CARTESIAN_POINT('Ctrl Pts',(0.981562530939489,1.,-1.64665139190656));
#36750=CARTESIAN_POINT('Ctrl Pts',(0.977689794119416,-1.,-1.64233990826687));
#36751=CARTESIAN_POINT('Ctrl Pts',(0.977689794119416,1.,-1.64233990826687));
#36752=CARTESIAN_POINT('Ctrl Pts',(0.974066058287418,-1.,-1.63820952658144));
#36753=CARTESIAN_POINT('Ctrl Pts',(0.974066058287418,1.,-1.63820952658144));
#36754=CARTESIAN_POINT('Ctrl Pts',(0.970669715997509,-1.,-1.63420665729798));
#36755=CARTESIAN_POINT('Ctrl Pts',(0.970669715997509,1.,-1.63420665729798));
#36756=CARTESIAN_POINT('Ctrl Pts',(0.967387853230345,-1.,-1.63013849959462));
#36757=CARTESIAN_POINT('Ctrl Pts',(0.967387853230345,1.,-1.63013849959462));
#36758=CARTESIAN_POINT('Ctrl Pts',(0.964046107040535,-1.,-1.62571930670187));
#36759=CARTESIAN_POINT('Ctrl Pts',(0.964046107040535,1.,-1.62571930670187));
#36760=CARTESIAN_POINT('Ctrl Pts',(0.960438326101728,-1.,-1.62061638140221));
#36761=CARTESIAN_POINT('Ctrl Pts',(0.960438326101728,1.,-1.62061638140221));
#36762=CARTESIAN_POINT('Ctrl Pts',(0.95635442292067,-1.,-1.61449324337085));
#36763=CARTESIAN_POINT('Ctrl Pts',(0.95635442292067,1.,-1.61449324337085));
#36764=CARTESIAN_POINT('Ctrl Pts',(0.951613284356035,-1.,-1.60706069896936));
#36765=CARTESIAN_POINT('Ctrl Pts',(0.951613284356035,1.,-1.60706069896936));
#36766=CARTESIAN_POINT('Ctrl Pts',(0.946078063315257,-1.,-1.59810042043673));
#36767=CARTESIAN_POINT('Ctrl Pts',(0.946078063315257,1.,-1.59810042043673));
#36768=CARTESIAN_POINT('Ctrl Pts',(0.939646377893399,-1.,-1.58744937487176));
#36769=CARTESIAN_POINT('Ctrl Pts',(0.939646377893399,1.,-1.58744937487176));
#36770=CARTESIAN_POINT('Ctrl Pts',(0.932246680108685,-1.,-1.57499388382243));
#36771=CARTESIAN_POINT('Ctrl Pts',(0.932246680108685,1.,-1.57499388382243));
#36772=CARTESIAN_POINT('Ctrl Pts',(0.923832188944341,-1.,-1.56065988578893));
#36773=CARTESIAN_POINT('Ctrl Pts',(0.923832188944341,1.,-1.56065988578893));
#36774=CARTESIAN_POINT('Ctrl Pts',(0.914375919026456,-1.,-1.54440491149498));
#36775=CARTESIAN_POINT('Ctrl Pts',(0.914375919026456,1.,-1.54440491149498));
#36776=CARTESIAN_POINT('Ctrl Pts',(0.905967409625651,-1.,-1.52984849887993));
#36777=CARTESIAN_POINT('Ctrl Pts',(0.905967409625651,1.,-1.52984849887993));
#36778=CARTESIAN_POINT('Ctrl Pts',(0.89918504748351,-1.,-1.51805569590094));
#36779=CARTESIAN_POINT('Ctrl Pts',(0.89918504748351,1.,-1.51805569590094));
#36780=CARTESIAN_POINT('Ctrl Pts',(0.894452006964543,-1.,-1.50980486806688));
#36781=CARTESIAN_POINT('Ctrl Pts',(0.894452006964543,1.,-1.50980486806688));
#36782=CARTESIAN_POINT('Ctrl Pts',(0.892032620296855,-1.,-1.5055822144029));
#36783=CARTESIAN_POINT('Ctrl Pts',(0.892032620296855,1.,-1.5055822144029));
#36784=CARTESIAN_POINT('',(1.23627494547115,1.,-1.81978687191668));
#36785=CARTESIAN_POINT('Ctrl Pts',(1.23627494547115,1.,-1.81978687191668));
#36786=CARTESIAN_POINT('Ctrl Pts',(1.23509651170476,1.,-1.81925017193666));
#36787=CARTESIAN_POINT('Ctrl Pts',(1.2327422452705,1.,-1.81817389921279));
#36788=CARTESIAN_POINT('Ctrl Pts',(1.2292186489137,1.,-1.8165508718364));
#36789=CARTESIAN_POINT('Ctrl Pts',(1.2245361330495,1.,-1.81436959210434));
#36790=CARTESIAN_POINT('Ctrl Pts',(1.21870906103557,1.,-1.81161420806656));
#36791=CARTESIAN_POINT('Ctrl Pts',(1.21290815708314,1.,-1.80882996917129));
#36792=CARTESIAN_POINT('Ctrl Pts',(1.20713356605475,1.,-1.80601678480707));
#36793=CARTESIAN_POINT('Ctrl Pts',(1.20138548938974,1.,-1.80317454838603));
#36794=CARTESIAN_POINT('Ctrl Pts',(1.19566418930242,1.,-1.80030314369879));
#36795=CARTESIAN_POINT('Ctrl Pts',(1.18996997934445,1.,-1.79740245923478));
#36796=CARTESIAN_POINT('Ctrl Pts',(1.18430321697432,1.,-1.79447240321515));
#36797=CARTESIAN_POINT('Ctrl Pts',(1.17866429440809,1.,-1.79151291552689));
#36798=CARTESIAN_POINT('Ctrl Pts',(1.17305363177328,1.,-1.78852398877617));
#36799=CARTESIAN_POINT('Ctrl Pts',(1.16747166312303,1.,-1.78550566040443));
#36800=CARTESIAN_POINT('Ctrl Pts',(1.16191881298499,1.,-1.78245795881009));
#36801=CARTESIAN_POINT('Ctrl Pts',(1.15639547194698,1.,-1.77938085564275));
#36802=CARTESIAN_POINT('Ctrl Pts',(1.15090197841514,1.,-1.7762742255701));
#36803=CARTESIAN_POINT('Ctrl Pts',(1.1454385822692,1.,-1.77313777896194));
#36804=CARTESIAN_POINT('Ctrl Pts',(1.14000548336975,1.,-1.76997111386769));
#36805=CARTESIAN_POINT('Ctrl Pts',(1.1346029180462,1.,-1.76677384551862));
#36806=CARTESIAN_POINT('Ctrl Pts',(1.12923123555075,1.,-1.7635457196617));
#36807=CARTESIAN_POINT('Ctrl Pts',(1.12389096855086,1.,-1.76028671825096));
#36808=CARTESIAN_POINT('Ctrl Pts',(1.11858293216763,1.,-1.75699720772105));
#36809=CARTESIAN_POINT('Ctrl Pts',(1.11330807582551,1.,-1.7536777209463));
#36810=CARTESIAN_POINT('Ctrl Pts',(1.10806728183007,1.,-1.7503286607592));
#36811=CARTESIAN_POINT('Ctrl Pts',(1.10286118991143,1.,-1.74695004214923));
#36812=CARTESIAN_POINT('Ctrl Pts',(1.09768999241225,1.,-1.74354119236208));
#36813=CARTESIAN_POINT('Ctrl Pts',(1.09255329056493,1.,-1.74010053962247));
#36814=CARTESIAN_POINT('Ctrl Pts',(1.08745056285427,1.,-1.73662628326091));
#36815=CARTESIAN_POINT('Ctrl Pts',(1.08238162784749,1.,-1.73311705663407));
#36816=CARTESIAN_POINT('Ctrl Pts',(1.0773470373727,1.,-1.72957248977424));
#36817=CARTESIAN_POINT('Ctrl Pts',(1.07234866990252,1.,-1.72599406198488));
#36818=CARTESIAN_POINT('Ctrl Pts',(1.06738966975462,1.,-1.72238500928453));
#36819=CARTESIAN_POINT('Ctrl Pts',(1.06247324680647,1.,-1.71874858456904));
#36820=CARTESIAN_POINT('Ctrl Pts',(1.05760163192479,1.,-1.7150865442702));
#36821=CARTESIAN_POINT('Ctrl Pts',(1.05277517202855,1.,-1.71139783543989));
#36822=CARTESIAN_POINT('Ctrl Pts',(1.04799085404995,1.,-1.70767646263649));
#36823=CARTESIAN_POINT('Ctrl Pts',(1.04324363334554,1.,-1.70391338707982));
#36824=CARTESIAN_POINT('Ctrl Pts',(1.03852922490789,1.,-1.70010052930962));
#36825=CARTESIAN_POINT('Ctrl Pts',(1.03384646003588,1.,-1.69623414782771));
#36826=CARTESIAN_POINT('Ctrl Pts',(1.02919977579147,1.,-1.69231840863458));
#36827=CARTESIAN_POINT('Ctrl Pts',(1.02460180535255,1.,-1.68836910178447));
#36828=CARTESIAN_POINT('Ctrl Pts',(1.02006795074201,1.,-1.68440578021706));
#36829=CARTESIAN_POINT('Ctrl Pts',(1.01561026162773,1.,-1.68044289894798));
#36830=CARTESIAN_POINT('Ctrl Pts',(1.01123236493511,1.,-1.67648246776464));
#36831=CARTESIAN_POINT('Ctrl Pts',(1.00692206696414,1.,-1.67250335383293));
#36832=CARTESIAN_POINT('Ctrl Pts',(1.00265091003727,1.,-1.66846059277303));
#36833=CARTESIAN_POINT('Ctrl Pts',(0.998389654952757,1.,-1.66430758030376));
#36834=CARTESIAN_POINT('Ctrl Pts',(0.994121836661305,1.,-1.66001553809947));
#36835=CARTESIAN_POINT('Ctrl Pts',(0.989855627854164,1.,-1.65559044289699));
#36836=CARTESIAN_POINT('Ctrl Pts',(0.98564262292082,1.,-1.65110016612638));
#36837=CARTESIAN_POINT('Ctrl Pts',(0.981562530939489,1.,-1.64665139190656));
#36838=CARTESIAN_POINT('Ctrl Pts',(0.977689794119416,1.,-1.64233990826687));
#36839=CARTESIAN_POINT('Ctrl Pts',(0.974066058287418,1.,-1.63820952658144));
#36840=CARTESIAN_POINT('Ctrl Pts',(0.970669715997509,1.,-1.63420665729798));
#36841=CARTESIAN_POINT('Ctrl Pts',(0.967387853230345,1.,-1.63013849959462));
#36842=CARTESIAN_POINT('Ctrl Pts',(0.964046107040535,1.,-1.62571930670187));
#36843=CARTESIAN_POINT('Ctrl Pts',(0.960438326101728,1.,-1.62061638140221));
#36844=CARTESIAN_POINT('Ctrl Pts',(0.95635442292067,1.,-1.61449324337085));
#36845=CARTESIAN_POINT('Ctrl Pts',(0.951613284356035,1.,-1.60706069896936));
#36846=CARTESIAN_POINT('Ctrl Pts',(0.946078063315257,1.,-1.59810042043673));
#36847=CARTESIAN_POINT('Ctrl Pts',(0.939646377893399,1.,-1.58744937487176));
#36848=CARTESIAN_POINT('Ctrl Pts',(0.932246680108685,1.,-1.57499388382243));
#36849=CARTESIAN_POINT('Ctrl Pts',(0.923832188944341,1.,-1.56065988578893));
#36850=CARTESIAN_POINT('Ctrl Pts',(0.914375919026456,1.,-1.54440491149498));
#36851=CARTESIAN_POINT('Ctrl Pts',(0.905967409625651,1.,-1.52984849887993));
#36852=CARTESIAN_POINT('Ctrl Pts',(0.89918504748351,1.,-1.51805569590094));
#36853=CARTESIAN_POINT('Ctrl Pts',(0.894452006964543,1.,-1.50980486806688));
#36854=CARTESIAN_POINT('Ctrl Pts',(0.892032620296855,1.,-1.5055822144029));
#36855=CARTESIAN_POINT('',(1.23627494547115,0.,-1.81978687191668));
#36856=CARTESIAN_POINT('Origin',(1.34869019493419,0.,-1.73811241238545));
#36857=CARTESIAN_POINT('',(1.34869019493419,1.,-1.73811241238545));
#36858=CARTESIAN_POINT('',(1.23627494547115,1.,-1.81978687191668));
#36859=CARTESIAN_POINT('',(1.34869019493419,0.,-1.73811241238545));
#36860=CARTESIAN_POINT('Ctrl Pts',(1.15624053661742,-1.,-1.31362392696032));
#36861=CARTESIAN_POINT('Ctrl Pts',(1.15624053661742,1.,-1.31362392696032));
#36862=CARTESIAN_POINT('Ctrl Pts',(1.15950888730809,-1.,-1.31722977216397));
#36863=CARTESIAN_POINT('Ctrl Pts',(1.15950888730809,1.,-1.31722977216397));
#36864=CARTESIAN_POINT('Ctrl Pts',(1.16589330093588,-1.,-1.32428080721772));
#36865=CARTESIAN_POINT('Ctrl Pts',(1.16589330093588,1.,-1.32428080721772));
#36866=CARTESIAN_POINT('Ctrl Pts',(1.17501305789857,-1.,-1.33437539347008));
#36867=CARTESIAN_POINT('Ctrl Pts',(1.17501305789857,1.,-1.33437539347008));
#36868=CARTESIAN_POINT('Ctrl Pts',(1.18625865667441,-1.,-1.34687054001093));
#36869=CARTESIAN_POINT('Ctrl Pts',(1.18625865667441,1.,-1.34687054001093));
#36870=CARTESIAN_POINT('Ctrl Pts',(1.1987959077932,-1.,-1.36088705043885));
#36871=CARTESIAN_POINT('Ctrl Pts',(1.1987959077932,1.,-1.36088705043885));
#36872=CARTESIAN_POINT('Ctrl Pts',(1.20982812925645,-1.,-1.37331915607905));
#36873=CARTESIAN_POINT('Ctrl Pts',(1.20982812925645,1.,-1.37331915607905));
#36874=CARTESIAN_POINT('Ctrl Pts',(1.21938737280852,-1.,-1.38420564527715));
#36875=CARTESIAN_POINT('Ctrl Pts',(1.21938737280852,1.,-1.38420564527715));
#36876=CARTESIAN_POINT('Ctrl Pts',(1.22752961899387,-1.,-1.39361389568796));
#36877=CARTESIAN_POINT('Ctrl Pts',(1.22752961899387,1.,-1.39361389568796));
#36878=CARTESIAN_POINT('Ctrl Pts',(1.23434087290423,-1.,-1.40164708206106));
#36879=CARTESIAN_POINT('Ctrl Pts',(1.23434087290423,1.,-1.40164708206106));
#36880=CARTESIAN_POINT('Ctrl Pts',(1.23994455029534,-1.,-1.40845295531283));
#36881=CARTESIAN_POINT('Ctrl Pts',(1.23994455029534,1.,-1.40845295531283));
#36882=CARTESIAN_POINT('Ctrl Pts',(1.24450600513056,-1.,-1.41422913175179));
#36883=CARTESIAN_POINT('Ctrl Pts',(1.24450600513056,1.,-1.41422913175179));
#36884=CARTESIAN_POINT('Ctrl Pts',(1.24824430986571,-1.,-1.41923722596025));
#36885=CARTESIAN_POINT('Ctrl Pts',(1.24824430986571,1.,-1.41923722596025));
#36886=CARTESIAN_POINT('Ctrl Pts',(1.2514145557001,-1.,-1.42378102115575));
#36887=CARTESIAN_POINT('Ctrl Pts',(1.2514145557001,1.,-1.42378102115575));
#36888=CARTESIAN_POINT('Ctrl Pts',(1.25426945222639,-1.,-1.42815938799387));
#36889=CARTESIAN_POINT('Ctrl Pts',(1.25426945222639,1.,-1.42815938799387));
#36890=CARTESIAN_POINT('Ctrl Pts',(1.25702687965755,-1.,-1.43262645609691));
#36891=CARTESIAN_POINT('Ctrl Pts',(1.25702687965755,1.,-1.43262645609691));
#36892=CARTESIAN_POINT('Ctrl Pts',(1.25983531012005,-1.,-1.43734919180848));
#36893=CARTESIAN_POINT('Ctrl Pts',(1.25983531012005,1.,-1.43734919180848));
#36894=CARTESIAN_POINT('Ctrl Pts',(1.26273903323858,-1.,-1.44236470511303));
#36895=CARTESIAN_POINT('Ctrl Pts',(1.26273903323858,1.,-1.44236470511303));
#36896=CARTESIAN_POINT('Ctrl Pts',(1.26570925118868,-1.,-1.44761985001662));
#36897=CARTESIAN_POINT('Ctrl Pts',(1.26570925118868,1.,-1.44761985001662));
#36898=CARTESIAN_POINT('Ctrl Pts',(1.2686778680489,-1.,-1.45301422764247));
#36899=CARTESIAN_POINT('Ctrl Pts',(1.2686778680489,1.,-1.45301422764247));
#36900=CARTESIAN_POINT('Ctrl Pts',(1.27156805265289,-1.,-1.45843906294697));
#36901=CARTESIAN_POINT('Ctrl Pts',(1.27156805265289,1.,-1.45843906294697));
#36902=CARTESIAN_POINT('Ctrl Pts',(1.27433119897822,-1.,-1.46382431332476));
#36903=CARTESIAN_POINT('Ctrl Pts',(1.27433119897822,1.,-1.46382431332476));
#36904=CARTESIAN_POINT('Ctrl Pts',(1.27696414831089,-1.,-1.46916035917133));
#36905=CARTESIAN_POINT('Ctrl Pts',(1.27696414831089,1.,-1.46916035917133));
#36906=CARTESIAN_POINT('Ctrl Pts',(1.2794891824849,-1.,-1.4744717526707));
#36907=CARTESIAN_POINT('Ctrl Pts',(1.2794891824849,1.,-1.4744717526707));
#36908=CARTESIAN_POINT('Ctrl Pts',(1.28194158939517,-1.,-1.47980070347096));
#36909=CARTESIAN_POINT('Ctrl Pts',(1.28194158939517,1.,-1.47980070347096));
#36910=CARTESIAN_POINT('Ctrl Pts',(1.28435533880201,-1.,-1.4851881711891));
#36911=CARTESIAN_POINT('Ctrl Pts',(1.28435533880201,1.,-1.4851881711891));
#36912=CARTESIAN_POINT('Ctrl Pts',(1.2867467611644,-1.,-1.4906522831278));
#36913=CARTESIAN_POINT('Ctrl Pts',(1.2867467611644,1.,-1.4906522831278));
#36914=CARTESIAN_POINT('Ctrl Pts',(1.28911506584254,-1.,-1.49618896881754));
#36915=CARTESIAN_POINT('Ctrl Pts',(1.28911506584254,1.,-1.49618896881754));
#36916=CARTESIAN_POINT('Ctrl Pts',(1.29145022885181,-1.,-1.50178230149776));
#36917=CARTESIAN_POINT('Ctrl Pts',(1.29145022885181,1.,-1.50178230149776));
#36918=CARTESIAN_POINT('Ctrl Pts',(1.29373841372842,-1.,-1.50741159078365));
#36919=CARTESIAN_POINT('Ctrl Pts',(1.29373841372842,1.,-1.50741159078365));
#36920=CARTESIAN_POINT('Ctrl Pts',(1.29596850710509,-1.,-1.51305994241402));
#36921=CARTESIAN_POINT('Ctrl Pts',(1.29596850710509,1.,-1.51305994241402));
#36922=CARTESIAN_POINT('Ctrl Pts',(1.29813791800747,-1.,-1.51872184912724));
#36923=CARTESIAN_POINT('Ctrl Pts',(1.29813791800747,1.,-1.51872184912724));
#36924=CARTESIAN_POINT('Ctrl Pts',(1.30024984366328,-1.,-1.52439957861062));
#36925=CARTESIAN_POINT('Ctrl Pts',(1.30024984366328,1.,-1.52439957861062));
#36926=CARTESIAN_POINT('Ctrl Pts',(1.30231064395568,-1.,-1.53009970283891));
#36927=CARTESIAN_POINT('Ctrl Pts',(1.30231064395568,1.,-1.53009970283891));
#36928=CARTESIAN_POINT('Ctrl Pts',(1.30432735639489,-1.,-1.53582981268977));
#36929=CARTESIAN_POINT('Ctrl Pts',(1.30432735639489,1.,-1.53582981268977));
#36930=CARTESIAN_POINT('Ctrl Pts',(1.30630475189556,-1.,-1.54159462645432));
#36931=CARTESIAN_POINT('Ctrl Pts',(1.30630475189556,1.,-1.54159462645432));
#36932=CARTESIAN_POINT('Ctrl Pts',(1.30824393907473,-1.,-1.54739413957185));
#36933=CARTESIAN_POINT('Ctrl Pts',(1.30824393907473,1.,-1.54739413957185));
#36934=CARTESIAN_POINT('Ctrl Pts',(1.31014393684222,-1.,-1.55322568759481));
#36935=CARTESIAN_POINT('Ctrl Pts',(1.31014393684222,1.,-1.55322568759481));
#36936=CARTESIAN_POINT('Ctrl Pts',(1.31200264341696,-1.,-1.55908521254821));
#36937=CARTESIAN_POINT('Ctrl Pts',(1.31200264341696,1.,-1.55908521254821));
#36938=CARTESIAN_POINT('Ctrl Pts',(1.31381795281002,-1.,-1.56496872402353));
#36939=CARTESIAN_POINT('Ctrl Pts',(1.31381795281002,1.,-1.56496872402353));
#36940=CARTESIAN_POINT('Ctrl Pts',(1.31558903860016,-1.,-1.57087397835723));
#36941=CARTESIAN_POINT('Ctrl Pts',(1.31558903860016,1.,-1.57087397835723));
#36942=CARTESIAN_POINT('Ctrl Pts',(1.31731642317187,-1.,-1.5768005650559));
#36943=CARTESIAN_POINT('Ctrl Pts',(1.31731642317187,1.,-1.5768005650559));
#36944=CARTESIAN_POINT('Ctrl Pts',(1.31900135021432,-1.,-1.58274907898834));
#36945=CARTESIAN_POINT('Ctrl Pts',(1.31900135021432,1.,-1.58274907898834));
#36946=CARTESIAN_POINT('Ctrl Pts',(1.32064537110892,-1.,-1.58872057258245));
#36947=CARTESIAN_POINT('Ctrl Pts',(1.32064537110892,1.,-1.58872057258245));
#36948=CARTESIAN_POINT('Ctrl Pts',(1.32224985747682,-1.,-1.59471591079403));
#36949=CARTESIAN_POINT('Ctrl Pts',(1.32224985747682,1.,-1.59471591079403));
#36950=CARTESIAN_POINT('Ctrl Pts',(1.32381550858256,-1.,-1.60073511858687));
#36951=CARTESIAN_POINT('Ctrl Pts',(1.32381550858256,1.,-1.60073511858687));
#36952=CARTESIAN_POINT('Ctrl Pts',(1.32534250785782,-1.,-1.60677758290954));
#36953=CARTESIAN_POINT('Ctrl Pts',(1.32534250785782,1.,-1.60677758290954));
#36954=CARTESIAN_POINT('Ctrl Pts',(1.32683074483356,-1.,-1.6128423401575));
#36955=CARTESIAN_POINT('Ctrl Pts',(1.32683074483356,1.,-1.6128423401575));
#36956=CARTESIAN_POINT('Ctrl Pts',(1.32828000610449,-1.,-1.61892832270724));
#36957=CARTESIAN_POINT('Ctrl Pts',(1.32828000610449,1.,-1.61892832270724));
#36958=CARTESIAN_POINT('Ctrl Pts',(1.3296901950568,-1.,-1.62503464209797));
#36959=CARTESIAN_POINT('Ctrl Pts',(1.3296901950568,1.,-1.62503464209797));
#36960=CARTESIAN_POINT('Ctrl Pts',(1.33106149345645,-1.,-1.63116079730923));
#36961=CARTESIAN_POINT('Ctrl Pts',(1.33106149345645,1.,-1.63116079730923));
#36962=CARTESIAN_POINT('Ctrl Pts',(1.33239425103724,-1.,-1.63730653475089));
#36963=CARTESIAN_POINT('Ctrl Pts',(1.33239425103724,1.,-1.63730653475089));
#36964=CARTESIAN_POINT('Ctrl Pts',(1.33368890676572,-1.,-1.6434717485603));
#36965=CARTESIAN_POINT('Ctrl Pts',(1.33368890676572,1.,-1.6434717485603));
#36966=CARTESIAN_POINT('Ctrl Pts',(1.33494590467993,-1.,-1.6496563728683));
#36967=CARTESIAN_POINT('Ctrl Pts',(1.33494590467993,1.,-1.6496563728683));
#36968=CARTESIAN_POINT('Ctrl Pts',(1.33616559745172,-1.,-1.65586025952593));
#36969=CARTESIAN_POINT('Ctrl Pts',(1.33616559745172,1.,-1.65586025952593));
#36970=CARTESIAN_POINT('Ctrl Pts',(1.33734820885262,-1.,-1.66208312541983));
#36971=CARTESIAN_POINT('Ctrl Pts',(1.33734820885262,1.,-1.66208312541983));
#36972=CARTESIAN_POINT('Ctrl Pts',(1.33849388654388,-1.,-1.66832460783989));
#36973=CARTESIAN_POINT('Ctrl Pts',(1.33849388654388,1.,-1.66832460783989));
#36974=CARTESIAN_POINT('Ctrl Pts',(1.3396027347034,-1.,-1.67458429426086));
#36975=CARTESIAN_POINT('Ctrl Pts',(1.3396027347034,1.,-1.67458429426086));
#36976=CARTESIAN_POINT('Ctrl Pts',(1.34067485185203,-1.,-1.68086176030362));
#36977=CARTESIAN_POINT('Ctrl Pts',(1.34067485185203,1.,-1.68086176030362));
#36978=CARTESIAN_POINT('Ctrl Pts',(1.341710374848,-1.,-1.68715660868764));
#36979=CARTESIAN_POINT('Ctrl Pts',(1.341710374848,1.,-1.68715660868764));
#36980=CARTESIAN_POINT('Ctrl Pts',(1.34270948206319,-1.,-1.6934684849687));
#36981=CARTESIAN_POINT('Ctrl Pts',(1.34270948206319,1.,-1.6934684849687));
#36982=CARTESIAN_POINT('Ctrl Pts',(1.34367237124483,-1.,-1.69979707754427));
#36983=CARTESIAN_POINT('Ctrl Pts',(1.34367237124483,1.,-1.69979707754427));
#36984=CARTESIAN_POINT('Ctrl Pts',(1.34459924533831,-1.,-1.70614212266738));
#36985=CARTESIAN_POINT('Ctrl Pts',(1.34459924533831,1.,-1.70614212266738));
#36986=CARTESIAN_POINT('Ctrl Pts',(1.34549029589416,-1.,-1.71250340686822));
#36987=CARTESIAN_POINT('Ctrl Pts',(1.34549029589416,1.,-1.71250340686822));
#36988=CARTESIAN_POINT('Ctrl Pts',(1.34634568653227,-1.,-1.7188807715049));
#36989=CARTESIAN_POINT('Ctrl Pts',(1.34634568653227,1.,-1.7188807715049));
#36990=CARTESIAN_POINT('Ctrl Pts',(1.34716554819527,-1.,-1.72527410680674));
#36991=CARTESIAN_POINT('Ctrl Pts',(1.34716554819527,1.,-1.72527410680674));
#36992=CARTESIAN_POINT('Ctrl Pts',(1.34779309152035,-1.,-1.7304014965394));
#36993=CARTESIAN_POINT('Ctrl Pts',(1.34779309152035,1.,-1.7304014965394));
#36994=CARTESIAN_POINT('Ctrl Pts',(1.34824783112887,-1.,-1.73425417885907));
#36995=CARTESIAN_POINT('Ctrl Pts',(1.34824783112887,1.,-1.73425417885907));
#36996=CARTESIAN_POINT('Ctrl Pts',(1.34854391898045,-1.,-1.73682580585691));
#36997=CARTESIAN_POINT('Ctrl Pts',(1.34854391898045,1.,-1.73682580585691));
#36998=CARTESIAN_POINT('Ctrl Pts',(1.34869019493419,-1.,-1.73811241238545));
#36999=CARTESIAN_POINT('Ctrl Pts',(1.34869019493419,1.,-1.73811241238545));
#37000=CARTESIAN_POINT('',(1.15624053661742,1.,-1.31362392696032));
#37001=CARTESIAN_POINT('Ctrl Pts',(1.15624053661742,1.,-1.31362392696032));
#37002=CARTESIAN_POINT('Ctrl Pts',(1.15950888730809,1.,-1.31722977216397));
#37003=CARTESIAN_POINT('Ctrl Pts',(1.16589330093588,1.,-1.32428080721772));
#37004=CARTESIAN_POINT('Ctrl Pts',(1.17501305789857,1.,-1.33437539347008));
#37005=CARTESIAN_POINT('Ctrl Pts',(1.18625865667441,1.,-1.34687054001093));
#37006=CARTESIAN_POINT('Ctrl Pts',(1.1987959077932,1.,-1.36088705043885));
#37007=CARTESIAN_POINT('Ctrl Pts',(1.20982812925645,1.,-1.37331915607905));
#37008=CARTESIAN_POINT('Ctrl Pts',(1.21938737280852,1.,-1.38420564527715));
#37009=CARTESIAN_POINT('Ctrl Pts',(1.22752961899387,1.,-1.39361389568796));
#37010=CARTESIAN_POINT('Ctrl Pts',(1.23434087290423,1.,-1.40164708206106));
#37011=CARTESIAN_POINT('Ctrl Pts',(1.23994455029534,1.,-1.40845295531283));
#37012=CARTESIAN_POINT('Ctrl Pts',(1.24450600513056,1.,-1.41422913175179));
#37013=CARTESIAN_POINT('Ctrl Pts',(1.24824430986571,1.,-1.41923722596025));
#37014=CARTESIAN_POINT('Ctrl Pts',(1.2514145557001,1.,-1.42378102115575));
#37015=CARTESIAN_POINT('Ctrl Pts',(1.25426945222639,1.,-1.42815938799387));
#37016=CARTESIAN_POINT('Ctrl Pts',(1.25702687965755,1.,-1.43262645609691));
#37017=CARTESIAN_POINT('Ctrl Pts',(1.25983531012005,1.,-1.43734919180848));
#37018=CARTESIAN_POINT('Ctrl Pts',(1.26273903323858,1.,-1.44236470511303));
#37019=CARTESIAN_POINT('Ctrl Pts',(1.26570925118868,1.,-1.44761985001662));
#37020=CARTESIAN_POINT('Ctrl Pts',(1.2686778680489,1.,-1.45301422764247));
#37021=CARTESIAN_POINT('Ctrl Pts',(1.27156805265289,1.,-1.45843906294697));
#37022=CARTESIAN_POINT('Ctrl Pts',(1.27433119897822,1.,-1.46382431332476));
#37023=CARTESIAN_POINT('Ctrl Pts',(1.27696414831089,1.,-1.46916035917133));
#37024=CARTESIAN_POINT('Ctrl Pts',(1.2794891824849,1.,-1.4744717526707));
#37025=CARTESIAN_POINT('Ctrl Pts',(1.28194158939517,1.,-1.47980070347096));
#37026=CARTESIAN_POINT('Ctrl Pts',(1.28435533880201,1.,-1.4851881711891));
#37027=CARTESIAN_POINT('Ctrl Pts',(1.2867467611644,1.,-1.4906522831278));
#37028=CARTESIAN_POINT('Ctrl Pts',(1.28911506584254,1.,-1.49618896881754));
#37029=CARTESIAN_POINT('Ctrl Pts',(1.29145022885181,1.,-1.50178230149776));
#37030=CARTESIAN_POINT('Ctrl Pts',(1.29373841372842,1.,-1.50741159078365));
#37031=CARTESIAN_POINT('Ctrl Pts',(1.29596850710509,1.,-1.51305994241402));
#37032=CARTESIAN_POINT('Ctrl Pts',(1.29813791800747,1.,-1.51872184912724));
#37033=CARTESIAN_POINT('Ctrl Pts',(1.30024984366328,1.,-1.52439957861062));
#37034=CARTESIAN_POINT('Ctrl Pts',(1.30231064395568,1.,-1.53009970283891));
#37035=CARTESIAN_POINT('Ctrl Pts',(1.30432735639489,1.,-1.53582981268977));
#37036=CARTESIAN_POINT('Ctrl Pts',(1.30630475189556,1.,-1.54159462645432));
#37037=CARTESIAN_POINT('Ctrl Pts',(1.30824393907473,1.,-1.54739413957185));
#37038=CARTESIAN_POINT('Ctrl Pts',(1.31014393684222,1.,-1.55322568759481));
#37039=CARTESIAN_POINT('Ctrl Pts',(1.31200264341696,1.,-1.55908521254821));
#37040=CARTESIAN_POINT('Ctrl Pts',(1.31381795281002,1.,-1.56496872402353));
#37041=CARTESIAN_POINT('Ctrl Pts',(1.31558903860016,1.,-1.57087397835723));
#37042=CARTESIAN_POINT('Ctrl Pts',(1.31731642317187,1.,-1.5768005650559));
#37043=CARTESIAN_POINT('Ctrl Pts',(1.31900135021432,1.,-1.58274907898834));
#37044=CARTESIAN_POINT('Ctrl Pts',(1.32064537110892,1.,-1.58872057258245));
#37045=CARTESIAN_POINT('Ctrl Pts',(1.32224985747682,1.,-1.59471591079403));
#37046=CARTESIAN_POINT('Ctrl Pts',(1.32381550858256,1.,-1.60073511858687));
#37047=CARTESIAN_POINT('Ctrl Pts',(1.32534250785782,1.,-1.60677758290954));
#37048=CARTESIAN_POINT('Ctrl Pts',(1.32683074483356,1.,-1.6128423401575));
#37049=CARTESIAN_POINT('Ctrl Pts',(1.32828000610449,1.,-1.61892832270724));
#37050=CARTESIAN_POINT('Ctrl Pts',(1.3296901950568,1.,-1.62503464209797));
#37051=CARTESIAN_POINT('Ctrl Pts',(1.33106149345645,1.,-1.63116079730923));
#37052=CARTESIAN_POINT('Ctrl Pts',(1.33239425103724,1.,-1.63730653475089));
#37053=CARTESIAN_POINT('Ctrl Pts',(1.33368890676572,1.,-1.6434717485603));
#37054=CARTESIAN_POINT('Ctrl Pts',(1.33494590467993,1.,-1.6496563728683));
#37055=CARTESIAN_POINT('Ctrl Pts',(1.33616559745172,1.,-1.65586025952593));
#37056=CARTESIAN_POINT('Ctrl Pts',(1.33734820885262,1.,-1.66208312541983));
#37057=CARTESIAN_POINT('Ctrl Pts',(1.33849388654388,1.,-1.66832460783989));
#37058=CARTESIAN_POINT('Ctrl Pts',(1.3396027347034,1.,-1.67458429426086));
#37059=CARTESIAN_POINT('Ctrl Pts',(1.34067485185203,1.,-1.68086176030362));
#37060=CARTESIAN_POINT('Ctrl Pts',(1.341710374848,1.,-1.68715660868764));
#37061=CARTESIAN_POINT('Ctrl Pts',(1.34270948206319,1.,-1.6934684849687));
#37062=CARTESIAN_POINT('Ctrl Pts',(1.34367237124483,1.,-1.69979707754427));
#37063=CARTESIAN_POINT('Ctrl Pts',(1.34459924533831,1.,-1.70614212266738));
#37064=CARTESIAN_POINT('Ctrl Pts',(1.34549029589416,1.,-1.71250340686822));
#37065=CARTESIAN_POINT('Ctrl Pts',(1.34634568653227,1.,-1.7188807715049));
#37066=CARTESIAN_POINT('Ctrl Pts',(1.34716554819527,1.,-1.72527410680674));
#37067=CARTESIAN_POINT('Ctrl Pts',(1.34779309152035,1.,-1.7304014965394));
#37068=CARTESIAN_POINT('Ctrl Pts',(1.34824783112887,1.,-1.73425417885907));
#37069=CARTESIAN_POINT('Ctrl Pts',(1.34854391898045,1.,-1.73682580585691));
#37070=CARTESIAN_POINT('Ctrl Pts',(1.34869019493419,1.,-1.73811241238545));
#37071=CARTESIAN_POINT('',(1.15624053661742,0.,-1.31362392696032));
#37072=CARTESIAN_POINT('Origin',(0.,0.,0.));
#37073=CARTESIAN_POINT('',(1.31362392696032,1.,-1.15624053661742));
#37074=CARTESIAN_POINT('Origin',(0.,1.,0.));
#37075=CARTESIAN_POINT('',(1.31362392696032,0.,-1.15624053661742));
#37076=CARTESIAN_POINT('Ctrl Pts',(1.73811241238545,-1.,-1.34869019493419));
#37077=CARTESIAN_POINT('Ctrl Pts',(1.73811241238545,1.,-1.34869019493419));
#37078=CARTESIAN_POINT('Ctrl Pts',(1.73682580585819,-1.,-1.34854391898145));
#37079=CARTESIAN_POINT('Ctrl Pts',(1.73682580585819,1.,-1.34854391898145));
#37080=CARTESIAN_POINT('Ctrl Pts',(1.73425417886254,-1.,-1.34824783113158));
#37081=CARTESIAN_POINT('Ctrl Pts',(1.73425417886254,1.,-1.34824783113158));
#37082=CARTESIAN_POINT('Ctrl Pts',(1.73040149654497,-1.,-1.3477930915247));
#37083=CARTESIAN_POINT('Ctrl Pts',(1.73040149654497,1.,-1.3477930915247));
#37084=CARTESIAN_POINT('Ctrl Pts',(1.72527410681298,-1.,-1.34716554820013));
#37085=CARTESIAN_POINT('Ctrl Pts',(1.72527410681298,1.,-1.34716554820013));
#37086=CARTESIAN_POINT('Ctrl Pts',(1.7188807715095,-1.,-1.34634568653586));
#37087=CARTESIAN_POINT('Ctrl Pts',(1.7188807715095,1.,-1.34634568653586));
#37088=CARTESIAN_POINT('Ctrl Pts',(1.71250340687011,-1.,-1.34549029589563));
#37089=CARTESIAN_POINT('Ctrl Pts',(1.71250340687011,1.,-1.34549029589563));
#37090=CARTESIAN_POINT('Ctrl Pts',(1.70614212266676,-1.,-1.34459924533783));
#37091=CARTESIAN_POINT('Ctrl Pts',(1.70614212266676,1.,-1.34459924533783));
#37092=CARTESIAN_POINT('Ctrl Pts',(1.69979707754221,-1.,-1.34367237124322));
#37093=CARTESIAN_POINT('Ctrl Pts',(1.69979707754221,1.,-1.34367237124322));
#37094=CARTESIAN_POINT('Ctrl Pts',(1.6934684849664,-1.,-1.34270948206139));
#37095=CARTESIAN_POINT('Ctrl Pts',(1.6934684849664,1.,-1.34270948206139));
#37096=CARTESIAN_POINT('Ctrl Pts',(1.68715660868602,-1.,-1.34171037484673));
#37097=CARTESIAN_POINT('Ctrl Pts',(1.68715660868602,1.,-1.34171037484673));
#37098=CARTESIAN_POINT('Ctrl Pts',(1.68086176030308,-1.,-1.3406748518516));
#37099=CARTESIAN_POINT('Ctrl Pts',(1.68086176030308,1.,-1.3406748518516));
#37100=CARTESIAN_POINT('Ctrl Pts',(1.67458429426126,-1.,-1.33960273470372));
#37101=CARTESIAN_POINT('Ctrl Pts',(1.67458429426126,1.,-1.33960273470372));
#37102=CARTESIAN_POINT('Ctrl Pts',(1.66832460784078,-1.,-1.33849388654458));
#37103=CARTESIAN_POINT('Ctrl Pts',(1.66832460784078,1.,-1.33849388654458));
#37104=CARTESIAN_POINT('Ctrl Pts',(1.66208312542073,-1.,-1.33734820885331));
#37105=CARTESIAN_POINT('Ctrl Pts',(1.66208312542073,1.,-1.33734820885331));
#37106=CARTESIAN_POINT('Ctrl Pts',(1.65586025952651,-1.,-1.33616559745217));
#37107=CARTESIAN_POINT('Ctrl Pts',(1.65586025952651,1.,-1.33616559745217));
#37108=CARTESIAN_POINT('Ctrl Pts',(1.64965637286843,-1.,-1.33494590468003));
#37109=CARTESIAN_POINT('Ctrl Pts',(1.64965637286843,1.,-1.33494590468003));
#37110=CARTESIAN_POINT('Ctrl Pts',(1.64347174856007,-1.,-1.33368890676554));
#37111=CARTESIAN_POINT('Ctrl Pts',(1.64347174856007,1.,-1.33368890676554));
#37112=CARTESIAN_POINT('Ctrl Pts',(1.63730653475049,-1.,-1.33239425103694));
#37113=CARTESIAN_POINT('Ctrl Pts',(1.63730653475049,1.,-1.33239425103694));
#37114=CARTESIAN_POINT('Ctrl Pts',(1.63116079730887,-1.,-1.33106149345618));
#37115=CARTESIAN_POINT('Ctrl Pts',(1.63116079730887,1.,-1.33106149345618));
#37116=CARTESIAN_POINT('Ctrl Pts',(1.62503464209777,-1.,-1.32969019505665));
#37117=CARTESIAN_POINT('Ctrl Pts',(1.62503464209777,1.,-1.32969019505665));
#37118=CARTESIAN_POINT('Ctrl Pts',(1.61892832270723,-1.,-1.32828000610448));
#37119=CARTESIAN_POINT('Ctrl Pts',(1.61892832270723,1.,-1.32828000610448));
#37120=CARTESIAN_POINT('Ctrl Pts',(1.61284234015762,-1.,-1.32683074483365));
#37121=CARTESIAN_POINT('Ctrl Pts',(1.61284234015762,1.,-1.32683074483365));
#37122=CARTESIAN_POINT('Ctrl Pts',(1.6067775829097,-1.,-1.32534250785794));
#37123=CARTESIAN_POINT('Ctrl Pts',(1.6067775829097,1.,-1.32534250785794));
#37124=CARTESIAN_POINT('Ctrl Pts',(1.600735118587,-1.,-1.32381550858266));
#37125=CARTESIAN_POINT('Ctrl Pts',(1.600735118587,1.,-1.32381550858266));
#37126=CARTESIAN_POINT('Ctrl Pts',(1.59471591079408,-1.,-1.32224985747686));
#37127=CARTESIAN_POINT('Ctrl Pts',(1.59471591079408,1.,-1.32224985747686));
#37128=CARTESIAN_POINT('Ctrl Pts',(1.58872057258244,-1.,-1.32064537110891));
#37129=CARTESIAN_POINT('Ctrl Pts',(1.58872057258244,1.,-1.32064537110891));
#37130=CARTESIAN_POINT('Ctrl Pts',(1.58274907898829,-1.,-1.31900135021428));
#37131=CARTESIAN_POINT('Ctrl Pts',(1.58274907898829,1.,-1.31900135021428));
#37132=CARTESIAN_POINT('Ctrl Pts',(1.57680056505585,-1.,-1.31731642317183));
#37133=CARTESIAN_POINT('Ctrl Pts',(1.57680056505585,1.,-1.31731642317183));
#37134=CARTESIAN_POINT('Ctrl Pts',(1.57087397835721,-1.,-1.31558903860015));
#37135=CARTESIAN_POINT('Ctrl Pts',(1.57087397835721,1.,-1.31558903860015));
#37136=CARTESIAN_POINT('Ctrl Pts',(1.56496872402352,-1.,-1.31381795281002));
#37137=CARTESIAN_POINT('Ctrl Pts',(1.56496872402352,1.,-1.31381795281002));
#37138=CARTESIAN_POINT('Ctrl Pts',(1.55908521254822,-1.,-1.31200264341696));
#37139=CARTESIAN_POINT('Ctrl Pts',(1.55908521254822,1.,-1.31200264341696));
#37140=CARTESIAN_POINT('Ctrl Pts',(1.55322568759481,-1.,-1.31014393684221));
#37141=CARTESIAN_POINT('Ctrl Pts',(1.55322568759481,1.,-1.31014393684221));
#37142=CARTESIAN_POINT('Ctrl Pts',(1.54739413957183,-1.,-1.30824393907471));
#37143=CARTESIAN_POINT('Ctrl Pts',(1.54739413957183,1.,-1.30824393907471));
#37144=CARTESIAN_POINT('Ctrl Pts',(1.54159462645428,-1.,-1.30630475189553));
#37145=CARTESIAN_POINT('Ctrl Pts',(1.54159462645428,1.,-1.30630475189553));
#37146=CARTESIAN_POINT('Ctrl Pts',(1.53582981268976,-1.,-1.30432735639487));
#37147=CARTESIAN_POINT('Ctrl Pts',(1.53582981268976,1.,-1.30432735639487));
#37148=CARTESIAN_POINT('Ctrl Pts',(1.53009970283893,-1.,-1.3023106439557));
#37149=CARTESIAN_POINT('Ctrl Pts',(1.53009970283893,1.,-1.3023106439557));
#37150=CARTESIAN_POINT('Ctrl Pts',(1.5243995786107,-1.,-1.30024984366334));
#37151=CARTESIAN_POINT('Ctrl Pts',(1.5243995786107,1.,-1.30024984366334));
#37152=CARTESIAN_POINT('Ctrl Pts',(1.51872184912735,-1.,-1.29813791800757));
#37153=CARTESIAN_POINT('Ctrl Pts',(1.51872184912735,1.,-1.29813791800757));
#37154=CARTESIAN_POINT('Ctrl Pts',(1.51305994241412,-1.,-1.29596850710518));
#37155=CARTESIAN_POINT('Ctrl Pts',(1.51305994241412,1.,-1.29596850710518));
#37156=CARTESIAN_POINT('Ctrl Pts',(1.50741159078367,-1.,-1.29373841372843));
#37157=CARTESIAN_POINT('Ctrl Pts',(1.50741159078367,1.,-1.29373841372843));
#37158=CARTESIAN_POINT('Ctrl Pts',(1.50178230149764,-1.,-1.29145022885171));
#37159=CARTESIAN_POINT('Ctrl Pts',(1.50178230149764,1.,-1.29145022885171));
#37160=CARTESIAN_POINT('Ctrl Pts',(1.49618896881729,-1.,-1.28911506584232));
#37161=CARTESIAN_POINT('Ctrl Pts',(1.49618896881729,1.,-1.28911506584232));
#37162=CARTESIAN_POINT('Ctrl Pts',(1.4906522831275,-1.,-1.28674676116415));
#37163=CARTESIAN_POINT('Ctrl Pts',(1.4906522831275,1.,-1.28674676116415));
#37164=CARTESIAN_POINT('Ctrl Pts',(1.48518817118891,-1.,-1.28435533880184));
#37165=CARTESIAN_POINT('Ctrl Pts',(1.48518817118891,1.,-1.28435533880184));
#37166=CARTESIAN_POINT('Ctrl Pts',(1.47980070347102,-1.,-1.28194158939522));
#37167=CARTESIAN_POINT('Ctrl Pts',(1.47980070347102,1.,-1.28194158939522));
#37168=CARTESIAN_POINT('Ctrl Pts',(1.4744717526711,-1.,-1.27948918248524));
#37169=CARTESIAN_POINT('Ctrl Pts',(1.4744717526711,1.,-1.27948918248524));
#37170=CARTESIAN_POINT('Ctrl Pts',(1.46916035917197,-1.,-1.27696414831144));
#37171=CARTESIAN_POINT('Ctrl Pts',(1.46916035917197,1.,-1.27696414831144));
#37172=CARTESIAN_POINT('Ctrl Pts',(1.4638243133254,-1.,-1.27433119897877));
#37173=CARTESIAN_POINT('Ctrl Pts',(1.4638243133254,1.,-1.27433119897877));
#37174=CARTESIAN_POINT('Ctrl Pts',(1.45843906294725,-1.,-1.27156805265312));
#37175=CARTESIAN_POINT('Ctrl Pts',(1.45843906294725,1.,-1.27156805265312));
#37176=CARTESIAN_POINT('Ctrl Pts',(1.45301422764205,-1.,-1.26867786804854));
#37177=CARTESIAN_POINT('Ctrl Pts',(1.45301422764205,1.,-1.26867786804854));
#37178=CARTESIAN_POINT('Ctrl Pts',(1.44761985001544,-1.,-1.26570925118767));
#37179=CARTESIAN_POINT('Ctrl Pts',(1.44761985001544,1.,-1.26570925118767));
#37180=CARTESIAN_POINT('Ctrl Pts',(1.44236470511145,-1.,-1.26273903323723));
#37181=CARTESIAN_POINT('Ctrl Pts',(1.44236470511145,1.,-1.26273903323723));
#37182=CARTESIAN_POINT('Ctrl Pts',(1.43734919180719,-1.,-1.25983531011894));
#37183=CARTESIAN_POINT('Ctrl Pts',(1.43734919180719,1.,-1.25983531011894));
#37184=CARTESIAN_POINT('Ctrl Pts',(1.43262645609679,-1.,-1.25702687965744));
#37185=CARTESIAN_POINT('Ctrl Pts',(1.43262645609679,1.,-1.25702687965744));
#37186=CARTESIAN_POINT('Ctrl Pts',(1.42815938799555,-1.,-1.25426945222783));
#37187=CARTESIAN_POINT('Ctrl Pts',(1.42815938799555,1.,-1.25426945222783));
#37188=CARTESIAN_POINT('Ctrl Pts',(1.42378102115911,-1.,-1.25141455570299));
#37189=CARTESIAN_POINT('Ctrl Pts',(1.42378102115911,1.,-1.25141455570299));
#37190=CARTESIAN_POINT('Ctrl Pts',(1.41923722596421,-1.,-1.24824430986911));
#37191=CARTESIAN_POINT('Ctrl Pts',(1.41923722596421,1.,-1.24824430986911));
#37192=CARTESIAN_POINT('Ctrl Pts',(1.41422913175437,-1.,-1.24450600513278));
#37193=CARTESIAN_POINT('Ctrl Pts',(1.41422913175437,1.,-1.24450600513278));
#37194=CARTESIAN_POINT('Ctrl Pts',(1.40845295531151,-1.,-1.23994455029421));
#37195=CARTESIAN_POINT('Ctrl Pts',(1.40845295531151,1.,-1.23994455029421));
#37196=CARTESIAN_POINT('Ctrl Pts',(1.40164708205345,-1.,-1.23434087289768));
#37197=CARTESIAN_POINT('Ctrl Pts',(1.40164708205345,1.,-1.23434087289768));
#37198=CARTESIAN_POINT('Ctrl Pts',(1.39361389567257,-1.,-1.22752961898063));
#37199=CARTESIAN_POINT('Ctrl Pts',(1.39361389567257,1.,-1.22752961898063));
#37200=CARTESIAN_POINT('Ctrl Pts',(1.38420564525391,-1.,-1.21938737278853));
#37201=CARTESIAN_POINT('Ctrl Pts',(1.38420564525391,1.,-1.21938737278853));
#37202=CARTESIAN_POINT('Ctrl Pts',(1.37331915604962,-1.,-1.20982812923113));
#37203=CARTESIAN_POINT('Ctrl Pts',(1.37331915604962,1.,-1.20982812923113));
#37204=CARTESIAN_POINT('Ctrl Pts',(1.36088705040677,-1.,-1.1987959077656));
#37205=CARTESIAN_POINT('Ctrl Pts',(1.36088705040677,1.,-1.1987959077656));
#37206=CARTESIAN_POINT('Ctrl Pts',(1.34687053998157,-1.,-1.18625865664915));
#37207=CARTESIAN_POINT('Ctrl Pts',(1.34687053998157,1.,-1.18625865664915));
#37208=CARTESIAN_POINT('Ctrl Pts',(1.33437539344842,-1.,-1.17501305787994));
#37209=CARTESIAN_POINT('Ctrl Pts',(1.33437539344842,1.,-1.17501305787994));
#37210=CARTESIAN_POINT('Ctrl Pts',(1.32428080720544,-1.,-1.16589330092532));
#37211=CARTESIAN_POINT('Ctrl Pts',(1.32428080720544,1.,-1.16589330092532));
#37212=CARTESIAN_POINT('Ctrl Pts',(1.3172297721596,-1.,-1.15950888730433));
#37213=CARTESIAN_POINT('Ctrl Pts',(1.3172297721596,1.,-1.15950888730433));
#37214=CARTESIAN_POINT('Ctrl Pts',(1.31362392696032,-1.,-1.15624053661742));
#37215=CARTESIAN_POINT('Ctrl Pts',(1.31362392696032,1.,-1.15624053661742));
#37216=CARTESIAN_POINT('',(1.73811241238545,1.,-1.34869019493419));
#37217=CARTESIAN_POINT('Ctrl Pts',(1.73811241238545,1.,-1.34869019493419));
#37218=CARTESIAN_POINT('Ctrl Pts',(1.73682580585819,1.,-1.34854391898145));
#37219=CARTESIAN_POINT('Ctrl Pts',(1.73425417886254,1.,-1.34824783113158));
#37220=CARTESIAN_POINT('Ctrl Pts',(1.73040149654497,1.,-1.3477930915247));
#37221=CARTESIAN_POINT('Ctrl Pts',(1.72527410681298,1.,-1.34716554820013));
#37222=CARTESIAN_POINT('Ctrl Pts',(1.7188807715095,1.,-1.34634568653586));
#37223=CARTESIAN_POINT('Ctrl Pts',(1.71250340687011,1.,-1.34549029589563));
#37224=CARTESIAN_POINT('Ctrl Pts',(1.70614212266676,1.,-1.34459924533783));
#37225=CARTESIAN_POINT('Ctrl Pts',(1.69979707754221,1.,-1.34367237124322));
#37226=CARTESIAN_POINT('Ctrl Pts',(1.6934684849664,1.,-1.34270948206139));
#37227=CARTESIAN_POINT('Ctrl Pts',(1.68715660868602,1.,-1.34171037484673));
#37228=CARTESIAN_POINT('Ctrl Pts',(1.68086176030308,1.,-1.3406748518516));
#37229=CARTESIAN_POINT('Ctrl Pts',(1.67458429426126,1.,-1.33960273470372));
#37230=CARTESIAN_POINT('Ctrl Pts',(1.66832460784078,1.,-1.33849388654458));
#37231=CARTESIAN_POINT('Ctrl Pts',(1.66208312542073,1.,-1.33734820885331));
#37232=CARTESIAN_POINT('Ctrl Pts',(1.65586025952651,1.,-1.33616559745217));
#37233=CARTESIAN_POINT('Ctrl Pts',(1.64965637286843,1.,-1.33494590468003));
#37234=CARTESIAN_POINT('Ctrl Pts',(1.64347174856007,1.,-1.33368890676554));
#37235=CARTESIAN_POINT('Ctrl Pts',(1.63730653475049,1.,-1.33239425103694));
#37236=CARTESIAN_POINT('Ctrl Pts',(1.63116079730887,1.,-1.33106149345618));
#37237=CARTESIAN_POINT('Ctrl Pts',(1.62503464209777,1.,-1.32969019505665));
#37238=CARTESIAN_POINT('Ctrl Pts',(1.61892832270723,1.,-1.32828000610448));
#37239=CARTESIAN_POINT('Ctrl Pts',(1.61284234015762,1.,-1.32683074483365));
#37240=CARTESIAN_POINT('Ctrl Pts',(1.6067775829097,1.,-1.32534250785794));
#37241=CARTESIAN_POINT('Ctrl Pts',(1.600735118587,1.,-1.32381550858266));
#37242=CARTESIAN_POINT('Ctrl Pts',(1.59471591079408,1.,-1.32224985747686));
#37243=CARTESIAN_POINT('Ctrl Pts',(1.58872057258244,1.,-1.32064537110891));
#37244=CARTESIAN_POINT('Ctrl Pts',(1.58274907898829,1.,-1.31900135021428));
#37245=CARTESIAN_POINT('Ctrl Pts',(1.57680056505585,1.,-1.31731642317183));
#37246=CARTESIAN_POINT('Ctrl Pts',(1.57087397835721,1.,-1.31558903860015));
#37247=CARTESIAN_POINT('Ctrl Pts',(1.56496872402352,1.,-1.31381795281002));
#37248=CARTESIAN_POINT('Ctrl Pts',(1.55908521254822,1.,-1.31200264341696));
#37249=CARTESIAN_POINT('Ctrl Pts',(1.55322568759481,1.,-1.31014393684221));
#37250=CARTESIAN_POINT('Ctrl Pts',(1.54739413957183,1.,-1.30824393907471));
#37251=CARTESIAN_POINT('Ctrl Pts',(1.54159462645428,1.,-1.30630475189553));
#37252=CARTESIAN_POINT('Ctrl Pts',(1.53582981268976,1.,-1.30432735639487));
#37253=CARTESIAN_POINT('Ctrl Pts',(1.53009970283893,1.,-1.3023106439557));
#37254=CARTESIAN_POINT('Ctrl Pts',(1.5243995786107,1.,-1.30024984366334));
#37255=CARTESIAN_POINT('Ctrl Pts',(1.51872184912735,1.,-1.29813791800757));
#37256=CARTESIAN_POINT('Ctrl Pts',(1.51305994241412,1.,-1.29596850710518));
#37257=CARTESIAN_POINT('Ctrl Pts',(1.50741159078367,1.,-1.29373841372843));
#37258=CARTESIAN_POINT('Ctrl Pts',(1.50178230149764,1.,-1.29145022885171));
#37259=CARTESIAN_POINT('Ctrl Pts',(1.49618896881729,1.,-1.28911506584232));
#37260=CARTESIAN_POINT('Ctrl Pts',(1.4906522831275,1.,-1.28674676116415));
#37261=CARTESIAN_POINT('Ctrl Pts',(1.48518817118891,1.,-1.28435533880184));
#37262=CARTESIAN_POINT('Ctrl Pts',(1.47980070347102,1.,-1.28194158939522));
#37263=CARTESIAN_POINT('Ctrl Pts',(1.4744717526711,1.,-1.27948918248524));
#37264=CARTESIAN_POINT('Ctrl Pts',(1.46916035917197,1.,-1.27696414831144));
#37265=CARTESIAN_POINT('Ctrl Pts',(1.4638243133254,1.,-1.27433119897877));
#37266=CARTESIAN_POINT('Ctrl Pts',(1.45843906294725,1.,-1.27156805265312));
#37267=CARTESIAN_POINT('Ctrl Pts',(1.45301422764205,1.,-1.26867786804854));
#37268=CARTESIAN_POINT('Ctrl Pts',(1.44761985001544,1.,-1.26570925118767));
#37269=CARTESIAN_POINT('Ctrl Pts',(1.44236470511145,1.,-1.26273903323723));
#37270=CARTESIAN_POINT('Ctrl Pts',(1.43734919180719,1.,-1.25983531011894));
#37271=CARTESIAN_POINT('Ctrl Pts',(1.43262645609679,1.,-1.25702687965744));
#37272=CARTESIAN_POINT('Ctrl Pts',(1.42815938799555,1.,-1.25426945222783));
#37273=CARTESIAN_POINT('Ctrl Pts',(1.42378102115911,1.,-1.25141455570299));
#37274=CARTESIAN_POINT('Ctrl Pts',(1.41923722596421,1.,-1.24824430986911));
#37275=CARTESIAN_POINT('Ctrl Pts',(1.41422913175437,1.,-1.24450600513278));
#37276=CARTESIAN_POINT('Ctrl Pts',(1.40845295531151,1.,-1.23994455029421));
#37277=CARTESIAN_POINT('Ctrl Pts',(1.40164708205345,1.,-1.23434087289768));
#37278=CARTESIAN_POINT('Ctrl Pts',(1.39361389567257,1.,-1.22752961898063));
#37279=CARTESIAN_POINT('Ctrl Pts',(1.38420564525391,1.,-1.21938737278853));
#37280=CARTESIAN_POINT('Ctrl Pts',(1.37331915604962,1.,-1.20982812923113));
#37281=CARTESIAN_POINT('Ctrl Pts',(1.36088705040677,1.,-1.1987959077656));
#37282=CARTESIAN_POINT('Ctrl Pts',(1.34687053998157,1.,-1.18625865664915));
#37283=CARTESIAN_POINT('Ctrl Pts',(1.33437539344842,1.,-1.17501305787994));
#37284=CARTESIAN_POINT('Ctrl Pts',(1.32428080720544,1.,-1.16589330092532));
#37285=CARTESIAN_POINT('Ctrl Pts',(1.3172297721596,1.,-1.15950888730433));
#37286=CARTESIAN_POINT('Ctrl Pts',(1.31362392696032,1.,-1.15624053661742));
#37287=CARTESIAN_POINT('',(1.73811241238545,0.,-1.34869019493419));
#37288=CARTESIAN_POINT('Origin',(1.81978687191668,0.,-1.23627494547115));
#37289=CARTESIAN_POINT('',(1.81978687191668,1.,-1.23627494547115));
#37290=CARTESIAN_POINT('',(1.73811241238545,1.,-1.34869019493419));
#37291=CARTESIAN_POINT('',(1.81978687191668,0.,-1.23627494547115));
#37292=CARTESIAN_POINT('Ctrl Pts',(1.5055822144029,-1.,-0.892032620296855));
#37293=CARTESIAN_POINT('Ctrl Pts',(1.5055822144029,1.,-0.892032620296855));
#37294=CARTESIAN_POINT('Ctrl Pts',(1.50980486807181,-1.,-0.894452006967538));
#37295=CARTESIAN_POINT('Ctrl Pts',(1.50980486807181,1.,-0.894452006967538));
#37296=CARTESIAN_POINT('Ctrl Pts',(1.51805569591479,-1.,-0.89918504749193));
#37297=CARTESIAN_POINT('Ctrl Pts',(1.51805569591479,1.,-0.89918504749193));
#37298=CARTESIAN_POINT('Ctrl Pts',(1.52984849890434,-1.,-0.905967409640499));
#37299=CARTESIAN_POINT('Ctrl Pts',(1.52984849890434,1.,-0.905967409640499));
#37300=CARTESIAN_POINT('Ctrl Pts',(1.54440491152807,-1.,-0.91437591904658));
#37301=CARTESIAN_POINT('Ctrl Pts',(1.54440491152807,1.,-0.91437591904658));
#37302=CARTESIAN_POINT('Ctrl Pts',(1.56065988582509,-1.,-0.923832188966322));
#37303=CARTESIAN_POINT('Ctrl Pts',(1.56065988582509,1.,-0.923832188966322));
#37304=CARTESIAN_POINT('Ctrl Pts',(1.57499388385561,-1.,-0.932246680128849));
#37305=CARTESIAN_POINT('Ctrl Pts',(1.57499388385561,1.,-0.932246680128849));
#37306=CARTESIAN_POINT('Ctrl Pts',(1.58744937489796,-1.,-0.939646377909319));
#37307=CARTESIAN_POINT('Ctrl Pts',(1.58744937489796,1.,-0.939646377909319));
#37308=CARTESIAN_POINT('Ctrl Pts',(1.59810042045408,-1.,-0.946078063325796));
#37309=CARTESIAN_POINT('Ctrl Pts',(1.59810042045408,1.,-0.946078063325796));
#37310=CARTESIAN_POINT('Ctrl Pts',(1.60706069897794,-1.,-0.951613284361248));
#37311=CARTESIAN_POINT('Ctrl Pts',(1.60706069897794,1.,-0.951613284361248));
#37312=CARTESIAN_POINT('Ctrl Pts',(1.61449324337233,-1.,-0.956354422921573));
#37313=CARTESIAN_POINT('Ctrl Pts',(1.61449324337233,1.,-0.956354422921573));
#37314=CARTESIAN_POINT('Ctrl Pts',(1.62061638139929,-1.,-0.960438326099958));
#37315=CARTESIAN_POINT('Ctrl Pts',(1.62061638139929,1.,-0.960438326099958));
#37316=CARTESIAN_POINT('Ctrl Pts',(1.6257193066974,-1.,-0.964046107037821));
#37317=CARTESIAN_POINT('Ctrl Pts',(1.6257193066974,1.,-0.964046107037821));
#37318=CARTESIAN_POINT('Ctrl Pts',(1.63013849959083,-1.,-0.967387853228041));
#37319=CARTESIAN_POINT('Ctrl Pts',(1.63013849959083,1.,-0.967387853228041));
#37320=CARTESIAN_POINT('Ctrl Pts',(1.63420665729609,-1.,-0.970669715996356));
#37321=CARTESIAN_POINT('Ctrl Pts',(1.63420665729609,1.,-0.970669715996356));
#37322=CARTESIAN_POINT('Ctrl Pts',(1.63820952658157,-1.,-0.974066058287501));
#37323=CARTESIAN_POINT('Ctrl Pts',(1.63820952658157,1.,-0.974066058287501));
#37324=CARTESIAN_POINT('Ctrl Pts',(1.64233990826831,-1.,-0.977689794120297));
#37325=CARTESIAN_POINT('Ctrl Pts',(1.64233990826831,1.,-0.977689794120297));
#37326=CARTESIAN_POINT('Ctrl Pts',(1.64665139190834,-1.,-0.981562530940574));
#37327=CARTESIAN_POINT('Ctrl Pts',(1.64665139190834,1.,-0.981562530940574));
#37328=CARTESIAN_POINT('Ctrl Pts',(1.6511001661277,-1.,-0.985642622921626));
#37329=CARTESIAN_POINT('Ctrl Pts',(1.6511001661277,1.,-0.985642622921626));
#37330=CARTESIAN_POINT('Ctrl Pts',(1.65559044289746,-1.,-0.98985562785445));
#37331=CARTESIAN_POINT('Ctrl Pts',(1.65559044289746,1.,-0.98985562785445));
#37332=CARTESIAN_POINT('Ctrl Pts',(1.66001553809916,-1.,-0.994121836661116));
#37333=CARTESIAN_POINT('Ctrl Pts',(1.66001553809916,1.,-0.994121836661116));
#37334=CARTESIAN_POINT('Ctrl Pts',(1.66430758030304,-1.,-0.998389654952317));
#37335=CARTESIAN_POINT('Ctrl Pts',(1.66430758030304,1.,-0.998389654952317));
#37336=CARTESIAN_POINT('Ctrl Pts',(1.66846059277231,-1.,-1.00265091003682));
#37337=CARTESIAN_POINT('Ctrl Pts',(1.66846059277231,1.,-1.00265091003682));
#37338=CARTESIAN_POINT('Ctrl Pts',(1.67250335383248,-1.,-1.00692206696387));
#37339=CARTESIAN_POINT('Ctrl Pts',(1.67250335383248,1.,-1.00692206696387));
#37340=CARTESIAN_POINT('Ctrl Pts',(1.67648246776457,-1.,-1.01123236493507));
#37341=CARTESIAN_POINT('Ctrl Pts',(1.67648246776457,1.,-1.01123236493507));
#37342=CARTESIAN_POINT('Ctrl Pts',(1.6804428989482,-1.,-1.01561026162787));
#37343=CARTESIAN_POINT('Ctrl Pts',(1.6804428989482,1.,-1.01561026162787));
#37344=CARTESIAN_POINT('Ctrl Pts',(1.68440578021739,-1.,-1.02006795074222));
#37345=CARTESIAN_POINT('Ctrl Pts',(1.68440578021739,1.,-1.02006795074222));
#37346=CARTESIAN_POINT('Ctrl Pts',(1.68836910178475,-1.,-1.02460180535272));
#37347=CARTESIAN_POINT('Ctrl Pts',(1.68836910178475,1.,-1.02460180535272));
#37348=CARTESIAN_POINT('Ctrl Pts',(1.69231840863471,-1.,-1.02919977579155));
#37349=CARTESIAN_POINT('Ctrl Pts',(1.69231840863471,1.,-1.02919977579155));
#37350=CARTESIAN_POINT('Ctrl Pts',(1.69623414782769,-1.,-1.03384646003587));
#37351=CARTESIAN_POINT('Ctrl Pts',(1.69623414782769,1.,-1.03384646003587));
#37352=CARTESIAN_POINT('Ctrl Pts',(1.70010052930951,-1.,-1.03852922490782));
#37353=CARTESIAN_POINT('Ctrl Pts',(1.70010052930951,1.,-1.03852922490782));
#37354=CARTESIAN_POINT('Ctrl Pts',(1.70391338707969,-1.,-1.04324363334546));
#37355=CARTESIAN_POINT('Ctrl Pts',(1.70391338707969,1.,-1.04324363334546));
#37356=CARTESIAN_POINT('Ctrl Pts',(1.70767646263641,-1.,-1.0479908540499));
#37357=CARTESIAN_POINT('Ctrl Pts',(1.70767646263641,1.,-1.0479908540499));
#37358=CARTESIAN_POINT('Ctrl Pts',(1.71139783543986,-1.,-1.05277517202854));
#37359=CARTESIAN_POINT('Ctrl Pts',(1.71139783543986,1.,-1.05277517202854));
#37360=CARTESIAN_POINT('Ctrl Pts',(1.71508654427022,-1.,-1.05760163192481));
#37361=CARTESIAN_POINT('Ctrl Pts',(1.71508654427022,1.,-1.05760163192481));
#37362=CARTESIAN_POINT('Ctrl Pts',(1.71874858456908,-1.,-1.0624732468065));
#37363=CARTESIAN_POINT('Ctrl Pts',(1.71874858456908,1.,-1.0624732468065));
#37364=CARTESIAN_POINT('Ctrl Pts',(1.72238500928456,-1.,-1.06738966975463));
#37365=CARTESIAN_POINT('Ctrl Pts',(1.72238500928456,1.,-1.06738966975463));
#37366=CARTESIAN_POINT('Ctrl Pts',(1.72599406198489,-1.,-1.07234866990252));
#37367=CARTESIAN_POINT('Ctrl Pts',(1.72599406198489,1.,-1.07234866990252));
#37368=CARTESIAN_POINT('Ctrl Pts',(1.72957248977424,-1.,-1.0773470373727));
#37369=CARTESIAN_POINT('Ctrl Pts',(1.72957248977424,1.,-1.0773470373727));
#37370=CARTESIAN_POINT('Ctrl Pts',(1.73311705663407,-1.,-1.08238162784749));
#37371=CARTESIAN_POINT('Ctrl Pts',(1.73311705663407,1.,-1.08238162784749));
#37372=CARTESIAN_POINT('Ctrl Pts',(1.73662628326093,-1.,-1.08745056285429));
#37373=CARTESIAN_POINT('Ctrl Pts',(1.73662628326093,1.,-1.08745056285429));
#37374=CARTESIAN_POINT('Ctrl Pts',(1.74010053962252,-1.,-1.09255329056496));
#37375=CARTESIAN_POINT('Ctrl Pts',(1.74010053962252,1.,-1.09255329056496));
#37376=CARTESIAN_POINT('Ctrl Pts',(1.74354119236212,-1.,-1.09768999241229));
#37377=CARTESIAN_POINT('Ctrl Pts',(1.74354119236212,1.,-1.09768999241229));
#37378=CARTESIAN_POINT('Ctrl Pts',(1.74695004214924,-1.,-1.10286118991144));
#37379=CARTESIAN_POINT('Ctrl Pts',(1.74695004214924,1.,-1.10286118991144));
#37380=CARTESIAN_POINT('Ctrl Pts',(1.75032866075914,-1.,-1.10806728183003));
#37381=CARTESIAN_POINT('Ctrl Pts',(1.75032866075914,1.,-1.10806728183003));
#37382=CARTESIAN_POINT('Ctrl Pts',(1.75367772094617,-1.,-1.11330807582542));
#37383=CARTESIAN_POINT('Ctrl Pts',(1.75367772094617,1.,-1.11330807582542));
#37384=CARTESIAN_POINT('Ctrl Pts',(1.75699720772089,-1.,-1.11858293216752));
#37385=CARTESIAN_POINT('Ctrl Pts',(1.75699720772089,1.,-1.11858293216752));
#37386=CARTESIAN_POINT('Ctrl Pts',(1.76028671825084,-1.,-1.12389096855078));
#37387=CARTESIAN_POINT('Ctrl Pts',(1.76028671825084,1.,-1.12389096855078));
#37388=CARTESIAN_POINT('Ctrl Pts',(1.76354571966171,-1.,-1.12923123555076));
#37389=CARTESIAN_POINT('Ctrl Pts',(1.76354571966171,1.,-1.12923123555076));
#37390=CARTESIAN_POINT('Ctrl Pts',(1.76677384551883,-1.,-1.13460291804635));
#37391=CARTESIAN_POINT('Ctrl Pts',(1.76677384551883,1.,-1.13460291804635));
#37392=CARTESIAN_POINT('Ctrl Pts',(1.76997111386806,-1.,-1.14000548337));
#37393=CARTESIAN_POINT('Ctrl Pts',(1.76997111386806,1.,-1.14000548337));
#37394=CARTESIAN_POINT('Ctrl Pts',(1.77313777896234,-1.,-1.14543858226948));
#37395=CARTESIAN_POINT('Ctrl Pts',(1.77313777896234,1.,-1.14543858226948));
#37396=CARTESIAN_POINT('Ctrl Pts',(1.77627422557034,-1.,-1.15090197841531));
#37397=CARTESIAN_POINT('Ctrl Pts',(1.77627422557034,1.,-1.15090197841531));
#37398=CARTESIAN_POINT('Ctrl Pts',(1.77938085564261,-1.,-1.15639547194689));
#37399=CARTESIAN_POINT('Ctrl Pts',(1.77938085564261,1.,-1.15639547194689));
#37400=CARTESIAN_POINT('Ctrl Pts',(1.78245795880949,-1.,-1.16191881298458));
#37401=CARTESIAN_POINT('Ctrl Pts',(1.78245795880949,1.,-1.16191881298458));
#37402=CARTESIAN_POINT('Ctrl Pts',(1.78550566040349,-1.,-1.16747166312239));
#37403=CARTESIAN_POINT('Ctrl Pts',(1.78550566040349,1.,-1.16747166312239));
#37404=CARTESIAN_POINT('Ctrl Pts',(1.78852398877523,-1.,-1.17305363177265));
#37405=CARTESIAN_POINT('Ctrl Pts',(1.78852398877523,1.,-1.17305363177265));
#37406=CARTESIAN_POINT('Ctrl Pts',(1.79151291552646,-1.,-1.17866429440781));
#37407=CARTESIAN_POINT('Ctrl Pts',(1.79151291552646,1.,-1.17866429440781));
#37408=CARTESIAN_POINT('Ctrl Pts',(1.79447240321572,-1.,-1.18430321697471));
#37409=CARTESIAN_POINT('Ctrl Pts',(1.79447240321572,1.,-1.18430321697471));
#37410=CARTESIAN_POINT('Ctrl Pts',(1.79740245923649,-1.,-1.1899699793456));
#37411=CARTESIAN_POINT('Ctrl Pts',(1.79740245923649,1.,-1.1899699793456));
#37412=CARTESIAN_POINT('Ctrl Pts',(1.80030314370121,-1.,-1.19566418930405));
#37413=CARTESIAN_POINT('Ctrl Pts',(1.80030314370121,1.,-1.19566418930405));
#37414=CARTESIAN_POINT('Ctrl Pts',(1.8031745483882,-1.,-1.2013854893912));
#37415=CARTESIAN_POINT('Ctrl Pts',(1.8031745483882,1.,-1.2013854893912));
#37416=CARTESIAN_POINT('Ctrl Pts',(1.80601678480772,-1.,-1.20713356605519));
#37417=CARTESIAN_POINT('Ctrl Pts',(1.80601678480772,1.,-1.20713356605519));
#37418=CARTESIAN_POINT('Ctrl Pts',(1.80882996916931,-1.,-1.2129081570818));
#37419=CARTESIAN_POINT('Ctrl Pts',(1.80882996916931,1.,-1.2129081570818));
#37420=CARTESIAN_POINT('Ctrl Pts',(1.81161420806172,-1.,-1.2187090610323));
#37421=CARTESIAN_POINT('Ctrl Pts',(1.81161420806172,1.,-1.2187090610323));
#37422=CARTESIAN_POINT('Ctrl Pts',(1.81436959209778,-1.,-1.22453613304507));
#37423=CARTESIAN_POINT('Ctrl Pts',(1.81436959209778,1.,-1.22453613304507));
#37424=CARTESIAN_POINT('Ctrl Pts',(1.81655087183054,-1.,-1.22921864890975));
#37425=CARTESIAN_POINT('Ctrl Pts',(1.81655087183054,1.,-1.22921864890975));
#37426=CARTESIAN_POINT('Ctrl Pts',(1.81817389920914,-1.,-1.23274224526804));
#37427=CARTESIAN_POINT('Ctrl Pts',(1.81817389920914,1.,-1.23274224526804));
#37428=CARTESIAN_POINT('Ctrl Pts',(1.81925017193531,-1.,-1.23509651170384));
#37429=CARTESIAN_POINT('Ctrl Pts',(1.81925017193531,1.,-1.23509651170384));
#37430=CARTESIAN_POINT('Ctrl Pts',(1.81978687191668,-1.,-1.23627494547115));
#37431=CARTESIAN_POINT('Ctrl Pts',(1.81978687191668,1.,-1.23627494547115));
#37432=CARTESIAN_POINT('',(1.5055822144029,1.,-0.892032620296855));
#37433=CARTESIAN_POINT('Ctrl Pts',(1.5055822144029,1.,-0.892032620296855));
#37434=CARTESIAN_POINT('Ctrl Pts',(1.50980486807181,1.,-0.894452006967538));
#37435=CARTESIAN_POINT('Ctrl Pts',(1.51805569591479,1.,-0.89918504749193));
#37436=CARTESIAN_POINT('Ctrl Pts',(1.52984849890434,1.,-0.905967409640499));
#37437=CARTESIAN_POINT('Ctrl Pts',(1.54440491152807,1.,-0.91437591904658));
#37438=CARTESIAN_POINT('Ctrl Pts',(1.56065988582509,1.,-0.923832188966322));
#37439=CARTESIAN_POINT('Ctrl Pts',(1.57499388385561,1.,-0.932246680128849));
#37440=CARTESIAN_POINT('Ctrl Pts',(1.58744937489796,1.,-0.939646377909319));
#37441=CARTESIAN_POINT('Ctrl Pts',(1.59810042045408,1.,-0.946078063325796));
#37442=CARTESIAN_POINT('Ctrl Pts',(1.60706069897794,1.,-0.951613284361248));
#37443=CARTESIAN_POINT('Ctrl Pts',(1.61449324337233,1.,-0.956354422921573));
#37444=CARTESIAN_POINT('Ctrl Pts',(1.62061638139929,1.,-0.960438326099958));
#37445=CARTESIAN_POINT('Ctrl Pts',(1.6257193066974,1.,-0.964046107037821));
#37446=CARTESIAN_POINT('Ctrl Pts',(1.63013849959083,1.,-0.967387853228041));
#37447=CARTESIAN_POINT('Ctrl Pts',(1.63420665729609,1.,-0.970669715996356));
#37448=CARTESIAN_POINT('Ctrl Pts',(1.63820952658157,1.,-0.974066058287501));
#37449=CARTESIAN_POINT('Ctrl Pts',(1.64233990826831,1.,-0.977689794120297));
#37450=CARTESIAN_POINT('Ctrl Pts',(1.64665139190834,1.,-0.981562530940574));
#37451=CARTESIAN_POINT('Ctrl Pts',(1.6511001661277,1.,-0.985642622921626));
#37452=CARTESIAN_POINT('Ctrl Pts',(1.65559044289746,1.,-0.98985562785445));
#37453=CARTESIAN_POINT('Ctrl Pts',(1.66001553809916,1.,-0.994121836661116));
#37454=CARTESIAN_POINT('Ctrl Pts',(1.66430758030304,1.,-0.998389654952317));
#37455=CARTESIAN_POINT('Ctrl Pts',(1.66846059277231,1.,-1.00265091003682));
#37456=CARTESIAN_POINT('Ctrl Pts',(1.67250335383248,1.,-1.00692206696387));
#37457=CARTESIAN_POINT('Ctrl Pts',(1.67648246776457,1.,-1.01123236493507));
#37458=CARTESIAN_POINT('Ctrl Pts',(1.6804428989482,1.,-1.01561026162787));
#37459=CARTESIAN_POINT('Ctrl Pts',(1.68440578021739,1.,-1.02006795074222));
#37460=CARTESIAN_POINT('Ctrl Pts',(1.68836910178475,1.,-1.02460180535272));
#37461=CARTESIAN_POINT('Ctrl Pts',(1.69231840863471,1.,-1.02919977579155));
#37462=CARTESIAN_POINT('Ctrl Pts',(1.69623414782769,1.,-1.03384646003587));
#37463=CARTESIAN_POINT('Ctrl Pts',(1.70010052930951,1.,-1.03852922490782));
#37464=CARTESIAN_POINT('Ctrl Pts',(1.70391338707969,1.,-1.04324363334546));
#37465=CARTESIAN_POINT('Ctrl Pts',(1.70767646263641,1.,-1.0479908540499));
#37466=CARTESIAN_POINT('Ctrl Pts',(1.71139783543986,1.,-1.05277517202854));
#37467=CARTESIAN_POINT('Ctrl Pts',(1.71508654427022,1.,-1.05760163192481));
#37468=CARTESIAN_POINT('Ctrl Pts',(1.71874858456908,1.,-1.0624732468065));
#37469=CARTESIAN_POINT('Ctrl Pts',(1.72238500928456,1.,-1.06738966975463));
#37470=CARTESIAN_POINT('Ctrl Pts',(1.72599406198489,1.,-1.07234866990252));
#37471=CARTESIAN_POINT('Ctrl Pts',(1.72957248977424,1.,-1.0773470373727));
#37472=CARTESIAN_POINT('Ctrl Pts',(1.73311705663407,1.,-1.08238162784749));
#37473=CARTESIAN_POINT('Ctrl Pts',(1.73662628326093,1.,-1.08745056285429));
#37474=CARTESIAN_POINT('Ctrl Pts',(1.74010053962252,1.,-1.09255329056496));
#37475=CARTESIAN_POINT('Ctrl Pts',(1.74354119236212,1.,-1.09768999241229));
#37476=CARTESIAN_POINT('Ctrl Pts',(1.74695004214924,1.,-1.10286118991144));
#37477=CARTESIAN_POINT('Ctrl Pts',(1.75032866075914,1.,-1.10806728183003));
#37478=CARTESIAN_POINT('Ctrl Pts',(1.75367772094617,1.,-1.11330807582542));
#37479=CARTESIAN_POINT('Ctrl Pts',(1.75699720772089,1.,-1.11858293216752));
#37480=CARTESIAN_POINT('Ctrl Pts',(1.76028671825084,1.,-1.12389096855078));
#37481=CARTESIAN_POINT('Ctrl Pts',(1.76354571966171,1.,-1.12923123555076));
#37482=CARTESIAN_POINT('Ctrl Pts',(1.76677384551883,1.,-1.13460291804635));
#37483=CARTESIAN_POINT('Ctrl Pts',(1.76997111386806,1.,-1.14000548337));
#37484=CARTESIAN_POINT('Ctrl Pts',(1.77313777896234,1.,-1.14543858226948));
#37485=CARTESIAN_POINT('Ctrl Pts',(1.77627422557034,1.,-1.15090197841531));
#37486=CARTESIAN_POINT('Ctrl Pts',(1.77938085564261,1.,-1.15639547194689));
#37487=CARTESIAN_POINT('Ctrl Pts',(1.78245795880949,1.,-1.16191881298458));
#37488=CARTESIAN_POINT('Ctrl Pts',(1.78550566040349,1.,-1.16747166312239));
#37489=CARTESIAN_POINT('Ctrl Pts',(1.78852398877523,1.,-1.17305363177265));
#37490=CARTESIAN_POINT('Ctrl Pts',(1.79151291552646,1.,-1.17866429440781));
#37491=CARTESIAN_POINT('Ctrl Pts',(1.79447240321572,1.,-1.18430321697471));
#37492=CARTESIAN_POINT('Ctrl Pts',(1.79740245923649,1.,-1.1899699793456));
#37493=CARTESIAN_POINT('Ctrl Pts',(1.80030314370121,1.,-1.19566418930405));
#37494=CARTESIAN_POINT('Ctrl Pts',(1.8031745483882,1.,-1.2013854893912));
#37495=CARTESIAN_POINT('Ctrl Pts',(1.80601678480772,1.,-1.20713356605519));
#37496=CARTESIAN_POINT('Ctrl Pts',(1.80882996916931,1.,-1.2129081570818));
#37497=CARTESIAN_POINT('Ctrl Pts',(1.81161420806172,1.,-1.2187090610323));
#37498=CARTESIAN_POINT('Ctrl Pts',(1.81436959209778,1.,-1.22453613304507));
#37499=CARTESIAN_POINT('Ctrl Pts',(1.81655087183054,1.,-1.22921864890975));
#37500=CARTESIAN_POINT('Ctrl Pts',(1.81817389920914,1.,-1.23274224526804));
#37501=CARTESIAN_POINT('Ctrl Pts',(1.81925017193531,1.,-1.23509651170384));
#37502=CARTESIAN_POINT('Ctrl Pts',(1.81978687191668,1.,-1.23627494547115));
#37503=CARTESIAN_POINT('',(1.5055822144029,0.,-0.892032620296855));
#37504=CARTESIAN_POINT('Origin',(0.,0.,0.));
#37505=CARTESIAN_POINT('',(1.60662857109684,1.,-0.693717979106306));
#37506=CARTESIAN_POINT('Origin',(0.,1.,0.));
#37507=CARTESIAN_POINT('',(1.60662857109684,0.,-0.693717979106308));
#37508=CARTESIAN_POINT('Ctrl Pts',(2.0698113262342,-1.,-0.745574324794401));
#37509=CARTESIAN_POINT('Ctrl Pts',(2.0698113262342,1.,-0.745574324794401));
#37510=CARTESIAN_POINT('Ctrl Pts',(2.06854248895728,-1.,-0.745832791378367));
#37511=CARTESIAN_POINT('Ctrl Pts',(2.06854248895728,1.,-0.745832791378367));
#37512=CARTESIAN_POINT('Ctrl Pts',(2.06600523016815,-1.,-0.746345871544201));
#37513=CARTESIAN_POINT('Ctrl Pts',(2.06600523016815,1.,-0.746345871544201));
#37514=CARTESIAN_POINT('Ctrl Pts',(2.06220058927826,-1.,-0.74710393278792));
#37515=CARTESIAN_POINT('Ctrl Pts',(2.06220058927826,1.,-0.74710393278792));
#37516=CARTESIAN_POINT('Ctrl Pts',(2.05713023031006,-1.,-0.748091554183803));
#37517=CARTESIAN_POINT('Ctrl Pts',(2.05713023031006,1.,-0.748091554183803));
#37518=CARTESIAN_POINT('Ctrl Pts',(2.05079645592154,-1.,-0.749287468665046));
#37519=CARTESIAN_POINT('Ctrl Pts',(2.05079645592154,1.,-0.749287468665046));
#37520=CARTESIAN_POINT('Ctrl Pts',(2.04446689147979,-1.,-0.750444657875576));
#37521=CARTESIAN_POINT('Ctrl Pts',(2.04446689147979,1.,-0.750444657875576));
#37522=CARTESIAN_POINT('Ctrl Pts',(2.03814160092099,-1.,-0.751562963361115));
#37523=CARTESIAN_POINT('Ctrl Pts',(2.03814160092099,1.,-0.751562963361115));
#37524=CARTESIAN_POINT('Ctrl Pts',(2.03182068456221,-1.,-0.752642180487211));
#37525=CARTESIAN_POINT('Ctrl Pts',(2.03182068456221,1.,-0.752642180487211));
#37526=CARTESIAN_POINT('Ctrl Pts',(2.02550428623313,-1.,-0.753682061112768));
#37527=CARTESIAN_POINT('Ctrl Pts',(2.02550428623313,1.,-0.753682061112768));
#37528=CARTESIAN_POINT('Ctrl Pts',(2.01919259405809,-1.,-0.754682330722816));
#37529=CARTESIAN_POINT('Ctrl Pts',(2.01919259405809,1.,-0.754682330722816));
#37530=CARTESIAN_POINT('Ctrl Pts',(2.01288584328084,-1.,-0.755642704957865));
#37531=CARTESIAN_POINT('Ctrl Pts',(2.01288584328084,1.,-0.755642704957865));
#37532=CARTESIAN_POINT('Ctrl Pts',(2.0065843158773,-1.,-0.756562904646671));
#37533=CARTESIAN_POINT('Ctrl Pts',(2.0065843158773,1.,-0.756562904646671));
#37534=CARTESIAN_POINT('Ctrl Pts',(2.00028834739178,-1.,-0.757442676862724));
#37535=CARTESIAN_POINT('Ctrl Pts',(2.00028834739178,1.,-0.757442676862724));
#37536=CARTESIAN_POINT('Ctrl Pts',(1.99399831098817,-1.,-0.758281796766761));
#37537=CARTESIAN_POINT('Ctrl Pts',(1.99399831098817,1.,-0.758281796766761));
#37538=CARTESIAN_POINT('Ctrl Pts',(1.98771456680874,-1.,-0.759080037802488));
#37539=CARTESIAN_POINT('Ctrl Pts',(1.98771456680874,1.,-0.759080037802488));
#37540=CARTESIAN_POINT('Ctrl Pts',(1.98143741418172,-1.,-0.75983714745219));
#37541=CARTESIAN_POINT('Ctrl Pts',(1.98143741418172,1.,-0.75983714745219));
#37542=CARTESIAN_POINT('Ctrl Pts',(1.97516705321494,-1.,-0.760552825409757));
#37543=CARTESIAN_POINT('Ctrl Pts',(1.97516705321494,1.,-0.760552825409757));
#37544=CARTESIAN_POINT('Ctrl Pts',(1.96890351582499,-1.,-0.761226690483821));
#37545=CARTESIAN_POINT('Ctrl Pts',(1.96890351582499,1.,-0.761226690483821));
#37546=CARTESIAN_POINT('Ctrl Pts',(1.96264672744186,-1.,-0.761858300014424));
#37547=CARTESIAN_POINT('Ctrl Pts',(1.96264672744186,1.,-0.761858300014424));
#37548=CARTESIAN_POINT('Ctrl Pts',(1.95639665309869,-1.,-0.762447203806179));
#37549=CARTESIAN_POINT('Ctrl Pts',(1.95639665309869,1.,-0.762447203806179));
#37550=CARTESIAN_POINT('Ctrl Pts',(1.95015342590024,-1.,-0.762992990878769));
#37551=CARTESIAN_POINT('Ctrl Pts',(1.95015342590024,1.,-0.762992990878769));
#37552=CARTESIAN_POINT('Ctrl Pts',(1.9439174661764,-1.,-0.763495333538629));
#37553=CARTESIAN_POINT('Ctrl Pts',(1.9439174661764,1.,-0.763495333538629));
#37554=CARTESIAN_POINT('Ctrl Pts',(1.93768964875886,-1.,-0.763954049121459));
#37555=CARTESIAN_POINT('Ctrl Pts',(1.93768964875886,1.,-0.763954049121459));
#37556=CARTESIAN_POINT('Ctrl Pts',(1.93147105496382,-1.,-0.764369010673941));
#37557=CARTESIAN_POINT('Ctrl Pts',(1.93147105496382,1.,-0.764369010673941));
#37558=CARTESIAN_POINT('Ctrl Pts',(1.92526263537048,-1.,-0.764740025488212));
#37559=CARTESIAN_POINT('Ctrl Pts',(1.92526263537048,1.,-0.764740025488212));
#37560=CARTESIAN_POINT('Ctrl Pts',(1.91906491634196,-1.,-0.765066729667089));
#37561=CARTESIAN_POINT('Ctrl Pts',(1.91906491634196,1.,-0.765066729667089));
#37562=CARTESIAN_POINT('Ctrl Pts',(1.91287765805169,-1.,-0.765348465884722));
#37563=CARTESIAN_POINT('Ctrl Pts',(1.91287765805169,1.,-0.765348465884722));
#37564=CARTESIAN_POINT('Ctrl Pts',(1.90669961402356,-1.,-0.765584196937919));
#37565=CARTESIAN_POINT('Ctrl Pts',(1.90669961402356,1.,-0.765584196937919));
#37566=CARTESIAN_POINT('Ctrl Pts',(1.90052930393596,-1.,-0.765772772593386));
#37567=CARTESIAN_POINT('Ctrl Pts',(1.90052930393596,1.,-0.765772772593386));
#37568=CARTESIAN_POINT('Ctrl Pts',(1.89436577771388,-1.,-0.765913193856978));
#37569=CARTESIAN_POINT('Ctrl Pts',(1.89436577771388,1.,-0.765913193856978));
#37570=CARTESIAN_POINT('Ctrl Pts',(1.88820926433409,-1.,-0.766004837062091));
#37571=CARTESIAN_POINT('Ctrl Pts',(1.88820926433409,1.,-0.766004837062091));
#37572=CARTESIAN_POINT('Ctrl Pts',(1.88206215302561,-1.,-0.766047794851865));
#37573=CARTESIAN_POINT('Ctrl Pts',(1.88206215302561,1.,-0.766047794851865));
#37574=CARTESIAN_POINT('Ctrl Pts',(1.87592888967883,-1.,-0.766042837036744));
#37575=CARTESIAN_POINT('Ctrl Pts',(1.87592888967883,1.,-0.766042837036744));
#37576=CARTESIAN_POINT('Ctrl Pts',(1.86981398314341,-1.,-0.765990708546091));
#37577=CARTESIAN_POINT('Ctrl Pts',(1.86981398314341,1.,-0.765990708546091));
#37578=CARTESIAN_POINT('Ctrl Pts',(1.86372027063312,-1.,-0.765891519092547));
#37579=CARTESIAN_POINT('Ctrl Pts',(1.86372027063312,1.,-0.765891519092547));
#37580=CARTESIAN_POINT('Ctrl Pts',(1.85764741390394,-1.,-0.765744212909319));
#37581=CARTESIAN_POINT('Ctrl Pts',(1.85764741390394,1.,-0.765744212909319));
#37582=CARTESIAN_POINT('Ctrl Pts',(1.85158945130063,-1.,-0.765545710619063));
#37583=CARTESIAN_POINT('Ctrl Pts',(1.85158945130063,1.,-0.765545710619063));
#37584=CARTESIAN_POINT('Ctrl Pts',(1.84553698875924,-1.,-0.765291664862029));
#37585=CARTESIAN_POINT('Ctrl Pts',(1.84553698875924,1.,-0.765291664862029));
#37586=CARTESIAN_POINT('Ctrl Pts',(1.83948181064835,-1.,-0.764978057881738));
#37587=CARTESIAN_POINT('Ctrl Pts',(1.83948181064835,1.,-0.764978057881738));
#37588=CARTESIAN_POINT('Ctrl Pts',(1.83342077227142,-1.,-0.764602549687853));
#37589=CARTESIAN_POINT('Ctrl Pts',(1.83342077227142,1.,-0.764602549687853));
#37590=CARTESIAN_POINT('Ctrl Pts',(1.82735991200065,-1.,-0.764165902605995));
#37591=CARTESIAN_POINT('Ctrl Pts',(1.82735991200065,1.,-0.764165902605995));
#37592=CARTESIAN_POINT('Ctrl Pts',(1.82131873145266,-1.,-0.763673465462727));
#37593=CARTESIAN_POINT('Ctrl Pts',(1.82131873145266,1.,-0.763673465462727));
#37594=CARTESIAN_POINT('Ctrl Pts',(1.8153211840553,-1.,-0.763132003836634));
#37595=CARTESIAN_POINT('Ctrl Pts',(1.8153211840553,1.,-0.763132003836634));
#37596=CARTESIAN_POINT('Ctrl Pts',(1.80938551463965,-1.,-0.762546129463938));
#37597=CARTESIAN_POINT('Ctrl Pts',(1.80938551463965,1.,-0.762546129463938));
#37598=CARTESIAN_POINT('Ctrl Pts',(1.80351583877342,-1.,-0.761915336443547));
#37599=CARTESIAN_POINT('Ctrl Pts',(1.80351583877342,1.,-0.761915336443547));
#37600=CARTESIAN_POINT('Ctrl Pts',(1.79768986997783,-1.,-0.761229695230558));
#37601=CARTESIAN_POINT('Ctrl Pts',(1.79768986997783,1.,-0.761229695230558));
#37602=CARTESIAN_POINT('Ctrl Pts',(1.7918581561088,-1.,-0.760469555880749));
#37603=CARTESIAN_POINT('Ctrl Pts',(1.7918581561088,1.,-0.760469555880749));
#37604=CARTESIAN_POINT('Ctrl Pts',(1.78596964884604,-1.,-0.75961440111019));
#37605=CARTESIAN_POINT('Ctrl Pts',(1.78596964884604,1.,-0.75961440111019));
#37606=CARTESIAN_POINT('Ctrl Pts',(1.77999411220945,-1.,-0.758650626677519));
#37607=CARTESIAN_POINT('Ctrl Pts',(1.77999411220945,1.,-0.758650626677519));
#37608=CARTESIAN_POINT('Ctrl Pts',(1.77394167108292,-1.,-0.757578264077029));
#37609=CARTESIAN_POINT('Ctrl Pts',(1.77394167108292,1.,-0.757578264077029));
#37610=CARTESIAN_POINT('Ctrl Pts',(1.76789396002998,-1.,-0.75642189602781));
#37611=CARTESIAN_POINT('Ctrl Pts',(1.76789396002998,1.,-0.75642189602781));
#37612=CARTESIAN_POINT('Ctrl Pts',(1.76197817240128,-1.,-0.755220979974462));
#37613=CARTESIAN_POINT('Ctrl Pts',(1.76197817240128,1.,-0.755220979974462));
#37614=CARTESIAN_POINT('Ctrl Pts',(1.75631083600019,-1.,-0.754009254027829));
#37615=CARTESIAN_POINT('Ctrl Pts',(1.75631083600019,1.,-0.754009254027829));
#37616=CARTESIAN_POINT('Ctrl Pts',(1.75095139468794,-1.,-0.752797683531314));
#37617=CARTESIAN_POINT('Ctrl Pts',(1.75095139468794,1.,-0.752797683531314));
#37618=CARTESIAN_POINT('Ctrl Pts',(1.74585086852502,-1.,-0.751555614164483));
#37619=CARTESIAN_POINT('Ctrl Pts',(1.74585086852502,1.,-0.751555614164483));
#37620=CARTESIAN_POINT('Ctrl Pts',(1.74080458267114,-1.,-0.75019343598125));
#37621=CARTESIAN_POINT('Ctrl Pts',(1.74080458267114,1.,-0.75019343598125));
#37622=CARTESIAN_POINT('Ctrl Pts',(1.7355035168033,-1.,-0.74858246295687));
#37623=CARTESIAN_POINT('Ctrl Pts',(1.7355035168033,1.,-0.74858246295687));
#37624=CARTESIAN_POINT('Ctrl Pts',(1.72958533647714,-1.,-0.746574710097752));
#37625=CARTESIAN_POINT('Ctrl Pts',(1.72958533647714,1.,-0.746574710097752));
#37626=CARTESIAN_POINT('Ctrl Pts',(1.72268229916769,-1.,-0.744021445433094));
#37627=CARTESIAN_POINT('Ctrl Pts',(1.72268229916769,1.,-0.744021445433094));
#37628=CARTESIAN_POINT('Ctrl Pts',(1.71447789751001,-1.,-0.74079516202821));
#37629=CARTESIAN_POINT('Ctrl Pts',(1.71447789751001,1.,-0.74079516202821));
#37630=CARTESIAN_POINT('Ctrl Pts',(1.70473309004249,-1.,-0.736799665716932));
#37631=CARTESIAN_POINT('Ctrl Pts',(1.70473309004249,1.,-0.736799665716932));
#37632=CARTESIAN_POINT('Ctrl Pts',(1.69326921972915,-1.,-0.731963238685357));
#37633=CARTESIAN_POINT('Ctrl Pts',(1.69326921972915,1.,-0.731963238685357));
#37634=CARTESIAN_POINT('Ctrl Pts',(1.67996158451922,-1.,-0.726235967982445));
#37635=CARTESIAN_POINT('Ctrl Pts',(1.67996158451922,1.,-0.726235967982445));
#37636=CARTESIAN_POINT('Ctrl Pts',(1.66472880551777,-1.,-0.71958543378795));
#37637=CARTESIAN_POINT('Ctrl Pts',(1.66472880551777,1.,-0.71958543378795));
#37638=CARTESIAN_POINT('Ctrl Pts',(1.64752408828442,-1.,-0.711993139340448));
#37639=CARTESIAN_POINT('Ctrl Pts',(1.64752408828442,1.,-0.711993139340448));
#37640=CARTESIAN_POINT('Ctrl Pts',(1.6321654166204,-1.,-0.705159151977294));
#37641=CARTESIAN_POINT('Ctrl Pts',(1.6321654166204,1.,-0.705159151977294));
#37642=CARTESIAN_POINT('Ctrl Pts',(1.61974673471117,-1.,-0.699605146398837));
#37643=CARTESIAN_POINT('Ctrl Pts',(1.61974673471117,1.,-0.699605146398837));
#37644=CARTESIAN_POINT('Ctrl Pts',(1.61106790957619,-1.,-0.69571209787897));
#37645=CARTESIAN_POINT('Ctrl Pts',(1.61106790957619,1.,-0.69571209787897));
#37646=CARTESIAN_POINT('Ctrl Pts',(1.60662857109684,-1.,-0.693717979106306));
#37647=CARTESIAN_POINT('Ctrl Pts',(1.60662857109684,1.,-0.693717979106306));
#37648=CARTESIAN_POINT('',(2.0698113262342,1.,-0.745574324794401));
#37649=CARTESIAN_POINT('Ctrl Pts',(2.0698113262342,1.,-0.745574324794401));
#37650=CARTESIAN_POINT('Ctrl Pts',(2.06854248895728,1.,-0.745832791378367));
#37651=CARTESIAN_POINT('Ctrl Pts',(2.06600523016815,1.,-0.746345871544201));
#37652=CARTESIAN_POINT('Ctrl Pts',(2.06220058927826,1.,-0.74710393278792));
#37653=CARTESIAN_POINT('Ctrl Pts',(2.05713023031006,1.,-0.748091554183803));
#37654=CARTESIAN_POINT('Ctrl Pts',(2.05079645592154,1.,-0.749287468665046));
#37655=CARTESIAN_POINT('Ctrl Pts',(2.04446689147979,1.,-0.750444657875576));
#37656=CARTESIAN_POINT('Ctrl Pts',(2.03814160092099,1.,-0.751562963361115));
#37657=CARTESIAN_POINT('Ctrl Pts',(2.03182068456221,1.,-0.752642180487211));
#37658=CARTESIAN_POINT('Ctrl Pts',(2.02550428623313,1.,-0.753682061112768));
#37659=CARTESIAN_POINT('Ctrl Pts',(2.01919259405809,1.,-0.754682330722816));
#37660=CARTESIAN_POINT('Ctrl Pts',(2.01288584328084,1.,-0.755642704957865));
#37661=CARTESIAN_POINT('Ctrl Pts',(2.0065843158773,1.,-0.756562904646671));
#37662=CARTESIAN_POINT('Ctrl Pts',(2.00028834739178,1.,-0.757442676862724));
#37663=CARTESIAN_POINT('Ctrl Pts',(1.99399831098817,1.,-0.758281796766761));
#37664=CARTESIAN_POINT('Ctrl Pts',(1.98771456680874,1.,-0.759080037802488));
#37665=CARTESIAN_POINT('Ctrl Pts',(1.98143741418172,1.,-0.75983714745219));
#37666=CARTESIAN_POINT('Ctrl Pts',(1.97516705321494,1.,-0.760552825409757));
#37667=CARTESIAN_POINT('Ctrl Pts',(1.96890351582499,1.,-0.761226690483821));
#37668=CARTESIAN_POINT('Ctrl Pts',(1.96264672744186,1.,-0.761858300014424));
#37669=CARTESIAN_POINT('Ctrl Pts',(1.95639665309869,1.,-0.762447203806179));
#37670=CARTESIAN_POINT('Ctrl Pts',(1.95015342590024,1.,-0.762992990878769));
#37671=CARTESIAN_POINT('Ctrl Pts',(1.9439174661764,1.,-0.763495333538629));
#37672=CARTESIAN_POINT('Ctrl Pts',(1.93768964875886,1.,-0.763954049121459));
#37673=CARTESIAN_POINT('Ctrl Pts',(1.93147105496382,1.,-0.764369010673941));
#37674=CARTESIAN_POINT('Ctrl Pts',(1.92526263537048,1.,-0.764740025488212));
#37675=CARTESIAN_POINT('Ctrl Pts',(1.91906491634196,1.,-0.765066729667089));
#37676=CARTESIAN_POINT('Ctrl Pts',(1.91287765805169,1.,-0.765348465884722));
#37677=CARTESIAN_POINT('Ctrl Pts',(1.90669961402356,1.,-0.765584196937919));
#37678=CARTESIAN_POINT('Ctrl Pts',(1.90052930393596,1.,-0.765772772593386));
#37679=CARTESIAN_POINT('Ctrl Pts',(1.89436577771388,1.,-0.765913193856978));
#37680=CARTESIAN_POINT('Ctrl Pts',(1.88820926433409,1.,-0.766004837062091));
#37681=CARTESIAN_POINT('Ctrl Pts',(1.88206215302561,1.,-0.766047794851865));
#37682=CARTESIAN_POINT('Ctrl Pts',(1.87592888967883,1.,-0.766042837036744));
#37683=CARTESIAN_POINT('Ctrl Pts',(1.86981398314341,1.,-0.765990708546091));
#37684=CARTESIAN_POINT('Ctrl Pts',(1.86372027063312,1.,-0.765891519092547));
#37685=CARTESIAN_POINT('Ctrl Pts',(1.85764741390394,1.,-0.765744212909319));
#37686=CARTESIAN_POINT('Ctrl Pts',(1.85158945130063,1.,-0.765545710619063));
#37687=CARTESIAN_POINT('Ctrl Pts',(1.84553698875924,1.,-0.765291664862029));
#37688=CARTESIAN_POINT('Ctrl Pts',(1.83948181064835,1.,-0.764978057881738));
#37689=CARTESIAN_POINT('Ctrl Pts',(1.83342077227142,1.,-0.764602549687853));
#37690=CARTESIAN_POINT('Ctrl Pts',(1.82735991200065,1.,-0.764165902605995));
#37691=CARTESIAN_POINT('Ctrl Pts',(1.82131873145266,1.,-0.763673465462727));
#37692=CARTESIAN_POINT('Ctrl Pts',(1.8153211840553,1.,-0.763132003836634));
#37693=CARTESIAN_POINT('Ctrl Pts',(1.80938551463965,1.,-0.762546129463938));
#37694=CARTESIAN_POINT('Ctrl Pts',(1.80351583877342,1.,-0.761915336443547));
#37695=CARTESIAN_POINT('Ctrl Pts',(1.79768986997783,1.,-0.761229695230558));
#37696=CARTESIAN_POINT('Ctrl Pts',(1.7918581561088,1.,-0.760469555880749));
#37697=CARTESIAN_POINT('Ctrl Pts',(1.78596964884604,1.,-0.75961440111019));
#37698=CARTESIAN_POINT('Ctrl Pts',(1.77999411220945,1.,-0.758650626677519));
#37699=CARTESIAN_POINT('Ctrl Pts',(1.77394167108292,1.,-0.757578264077029));
#37700=CARTESIAN_POINT('Ctrl Pts',(1.76789396002998,1.,-0.75642189602781));
#37701=CARTESIAN_POINT('Ctrl Pts',(1.76197817240128,1.,-0.755220979974462));
#37702=CARTESIAN_POINT('Ctrl Pts',(1.75631083600019,1.,-0.754009254027829));
#37703=CARTESIAN_POINT('Ctrl Pts',(1.75095139468794,1.,-0.752797683531314));
#37704=CARTESIAN_POINT('Ctrl Pts',(1.74585086852502,1.,-0.751555614164483));
#37705=CARTESIAN_POINT('Ctrl Pts',(1.74080458267114,1.,-0.75019343598125));
#37706=CARTESIAN_POINT('Ctrl Pts',(1.7355035168033,1.,-0.74858246295687));
#37707=CARTESIAN_POINT('Ctrl Pts',(1.72958533647714,1.,-0.746574710097752));
#37708=CARTESIAN_POINT('Ctrl Pts',(1.72268229916769,1.,-0.744021445433094));
#37709=CARTESIAN_POINT('Ctrl Pts',(1.71447789751001,1.,-0.74079516202821));
#37710=CARTESIAN_POINT('Ctrl Pts',(1.70473309004249,1.,-0.736799665716932));
#37711=CARTESIAN_POINT('Ctrl Pts',(1.69326921972915,1.,-0.731963238685357));
#37712=CARTESIAN_POINT('Ctrl Pts',(1.67996158451922,1.,-0.726235967982445));
#37713=CARTESIAN_POINT('Ctrl Pts',(1.66472880551777,1.,-0.71958543378795));
#37714=CARTESIAN_POINT('Ctrl Pts',(1.64752408828442,1.,-0.711993139340448));
#37715=CARTESIAN_POINT('Ctrl Pts',(1.6321654166204,1.,-0.705159151977294));
#37716=CARTESIAN_POINT('Ctrl Pts',(1.61974673471117,1.,-0.699605146398837));
#37717=CARTESIAN_POINT('Ctrl Pts',(1.61106790957619,1.,-0.69571209787897));
#37718=CARTESIAN_POINT('Ctrl Pts',(1.60662857109684,1.,-0.693717979106306));
#37719=CARTESIAN_POINT('',(2.0698113262342,0.,-0.745574324794401));
#37720=CARTESIAN_POINT('Origin',(2.11275013067528,0.,-0.61342227326009));
#37721=CARTESIAN_POINT('',(2.11275013067528,1.,-0.61342227326009));
#37722=CARTESIAN_POINT('',(2.0698113262342,1.,-0.745574324794401));
#37723=CARTESIAN_POINT('',(2.11275013067528,0.,-0.61342227326009));
#37724=CARTESIAN_POINT('Ctrl Pts',(1.7075470150345,-1.,-0.383122945602004));
#37725=CARTESIAN_POINT('Ctrl Pts',(1.7075470150345,1.,-0.383122945602004));
#37726=CARTESIAN_POINT('Ctrl Pts',(1.71231062891958,-1.,-0.384119047315542));
#37727=CARTESIAN_POINT('Ctrl Pts',(1.71231062891958,1.,-0.384119047315542));
#37728=CARTESIAN_POINT('Ctrl Pts',(1.72162022246158,-1.,-0.38607079032701));
#37729=CARTESIAN_POINT('Ctrl Pts',(1.72162022246158,1.,-0.38607079032701));
#37730=CARTESIAN_POINT('Ctrl Pts',(1.7349317097561,-1.,-0.388877023509192));
#37731=CARTESIAN_POINT('Ctrl Pts',(1.7349317097561,1.,-0.388877023509192));
#37732=CARTESIAN_POINT('Ctrl Pts',(1.75137405313962,-1.,-0.392375812294307));
#37733=CARTESIAN_POINT('Ctrl Pts',(1.75137405313962,1.,-0.392375812294307));
#37734=CARTESIAN_POINT('Ctrl Pts',(1.7697556004756,-1.,-0.39634619612042));
#37735=CARTESIAN_POINT('Ctrl Pts',(1.7697556004756,1.,-0.39634619612042));
#37736=CARTESIAN_POINT('Ctrl Pts',(1.78598826347533,-1.,-0.399919403783081));
#37737=CARTESIAN_POINT('Ctrl Pts',(1.78598826347533,1.,-0.399919403783081));
#37738=CARTESIAN_POINT('Ctrl Pts',(1.80012077176221,-1.,-0.403107976170441));
#37739=CARTESIAN_POINT('Ctrl Pts',(1.80012077176221,1.,-0.403107976170441));
#37740=CARTESIAN_POINT('Ctrl Pts',(1.81223801813988,-1.,-0.405933518411838));
#37741=CARTESIAN_POINT('Ctrl Pts',(1.81223801813988,1.,-0.405933518411838));
#37742=CARTESIAN_POINT('Ctrl Pts',(1.8224702267854,-1.,-0.408428948108534));
#37743=CARTESIAN_POINT('Ctrl Pts',(1.8224702267854,1.,-0.408428948108534));
#37744=CARTESIAN_POINT('Ctrl Pts',(1.83100408895216,-1.,-0.410641256301675));
#37745=CARTESIAN_POINT('Ctrl Pts',(1.83100408895216,1.,-0.410641256301675));
#37746=CARTESIAN_POINT('Ctrl Pts',(1.83808953475839,-1.,-0.412633125322162));
#37747=CARTESIAN_POINT('Ctrl Pts',(1.83808953475839,1.,-0.412633125322162));
#37748=CARTESIAN_POINT('Ctrl Pts',(1.8440575707371,-1.,-0.41448743825434));
#37749=CARTESIAN_POINT('Ctrl Pts',(1.8440575707371,1.,-0.41448743825434));
#37750=CARTESIAN_POINT('Ctrl Pts',(1.84929312929882,-1.,-0.416300022038864));
#37751=CARTESIAN_POINT('Ctrl Pts',(1.84929312929882,1.,-0.416300022038864));
#37752=CARTESIAN_POINT('Ctrl Pts',(1.85417632856234,-1.,-0.418164129143534));
#37753=CARTESIAN_POINT('Ctrl Pts',(1.85417632856234,1.,-0.418164129143534));
#37754=CARTESIAN_POINT('Ctrl Pts',(1.85903281096686,-1.,-0.42015728797562));
#37755=CARTESIAN_POINT('Ctrl Pts',(1.85903281096686,1.,-0.42015728797562));
#37756=CARTESIAN_POINT('Ctrl Pts',(1.86408083334028,-1.,-0.422327307418275));
#37757=CARTESIAN_POINT('Ctrl Pts',(1.86408083334028,1.,-0.422327307418275));
#37758=CARTESIAN_POINT('Ctrl Pts',(1.86937803944323,-1.,-0.424678177291359));
#37759=CARTESIAN_POINT('Ctrl Pts',(1.86937803944323,1.,-0.424678177291359));
#37760=CARTESIAN_POINT('Ctrl Pts',(1.87486989291484,-1.,-0.427183828519102));
#37761=CARTESIAN_POINT('Ctrl Pts',(1.87486989291484,1.,-0.427183828519102));
#37762=CARTESIAN_POINT('Ctrl Pts',(1.88044229001832,-1.,-0.429803062482345));
#37763=CARTESIAN_POINT('Ctrl Pts',(1.88044229001832,1.,-0.429803062482345));
#37764=CARTESIAN_POINT('Ctrl Pts',(1.88596913666793,-1.,-0.432493038548748));
#37765=CARTESIAN_POINT('Ctrl Pts',(1.88596913666793,1.,-0.432493038548748));
#37766=CARTESIAN_POINT('Ctrl Pts',(1.89136993975504,-1.,-0.435225660963383));
#37767=CARTESIAN_POINT('Ctrl Pts',(1.89136993975504,1.,-0.435225660963383));
#37768=CARTESIAN_POINT('Ctrl Pts',(1.89663648956466,-1.,-0.437995003948244));
#37769=CARTESIAN_POINT('Ctrl Pts',(1.89663648956466,1.,-0.437995003948244));
#37770=CARTESIAN_POINT('Ctrl Pts',(1.90180124389086,-1.,-0.440807833704038));
#37771=CARTESIAN_POINT('Ctrl Pts',(1.90180124389086,1.,-0.440807833704038));
#37772=CARTESIAN_POINT('Ctrl Pts',(1.90691756144898,-1.,-0.443677556849151));
#37773=CARTESIAN_POINT('Ctrl Pts',(1.90691756144898,1.,-0.443677556849151));
#37774=CARTESIAN_POINT('Ctrl Pts',(1.9120369998112,-1.,-0.446617343485711));
#37775=CARTESIAN_POINT('Ctrl Pts',(1.9120369998112,1.,-0.446617343485711));
#37776=CARTESIAN_POINT('Ctrl Pts',(1.91718342555755,-1.,-0.449632260106662));
#37777=CARTESIAN_POINT('Ctrl Pts',(1.91718342555755,1.,-0.449632260106662));
#37778=CARTESIAN_POINT('Ctrl Pts',(1.92235380648502,-1.,-0.452719478359433));
#37779=CARTESIAN_POINT('Ctrl Pts',(1.92235380648502,1.,-0.452719478359433));
#37780=CARTESIAN_POINT('Ctrl Pts',(1.92753067150476,-1.,-0.455872005174371));
#37781=CARTESIAN_POINT('Ctrl Pts',(1.92753067150476,1.,-0.455872005174371));
#37782=CARTESIAN_POINT('Ctrl Pts',(1.93269066517934,-1.,-0.459081234547926));
#37783=CARTESIAN_POINT('Ctrl Pts',(1.93269066517934,1.,-0.459081234547926));
#37784=CARTESIAN_POINT('Ctrl Pts',(1.93781486640821,-1.,-0.462340031009057));
#37785=CARTESIAN_POINT('Ctrl Pts',(1.93781486640821,1.,-0.462340031009057));
#37786=CARTESIAN_POINT('Ctrl Pts',(1.9428979419619,-1.,-0.46564546202603));
#37787=CARTESIAN_POINT('Ctrl Pts',(1.9428979419619,1.,-0.46564546202603));
#37788=CARTESIAN_POINT('Ctrl Pts',(1.94794381136514,-1.,-0.468997482913135));
#37789=CARTESIAN_POINT('Ctrl Pts',(1.94794381136514,1.,-0.468997482913135));
#37790=CARTESIAN_POINT('Ctrl Pts',(1.95296148278133,-1.,-0.472397672264072));
#37791=CARTESIAN_POINT('Ctrl Pts',(1.95296148278133,1.,-0.472397672264072));
#37792=CARTESIAN_POINT('Ctrl Pts',(1.95796111148177,-1.,-0.475848034683176));
#37793=CARTESIAN_POINT('Ctrl Pts',(1.95796111148177,1.,-0.475848034683176));
#37794=CARTESIAN_POINT('Ctrl Pts',(1.96294933055943,-1.,-0.479349583074855));
#37795=CARTESIAN_POINT('Ctrl Pts',(1.96294933055943,1.,-0.479349583074855));
#37796=CARTESIAN_POINT('Ctrl Pts',(1.96792703422362,-1.,-0.482901662120691));
#37797=CARTESIAN_POINT('Ctrl Pts',(1.96792703422362,1.,-0.482901662120691));
#37798=CARTESIAN_POINT('Ctrl Pts',(1.97289186263272,-1.,-0.486502692907659));
#37799=CARTESIAN_POINT('Ctrl Pts',(1.97289186263272,1.,-0.486502692907659));
#37800=CARTESIAN_POINT('Ctrl Pts',(1.97783973019229,-1.,-0.490150627860953));
#37801=CARTESIAN_POINT('Ctrl Pts',(1.97783973019229,1.,-0.490150627860953));
#37802=CARTESIAN_POINT('Ctrl Pts',(1.98276658761821,-1.,-0.493843476541495));
#37803=CARTESIAN_POINT('Ctrl Pts',(1.98276658761821,1.,-0.493843476541495));
#37804=CARTESIAN_POINT('Ctrl Pts',(1.98767044752932,-1.,-0.497579909545574));
#37805=CARTESIAN_POINT('Ctrl Pts',(1.98767044752932,1.,-0.497579909545574));
#37806=CARTESIAN_POINT('Ctrl Pts',(1.99255149126155,-1.,-0.501359287727146));
#37807=CARTESIAN_POINT('Ctrl Pts',(1.99255149126155,1.,-0.501359287727146));
#37808=CARTESIAN_POINT('Ctrl Pts',(1.99741107463572,-1.,-0.505181361323026));
#37809=CARTESIAN_POINT('Ctrl Pts',(1.99741107463572,1.,-0.505181361323026));
#37810=CARTESIAN_POINT('Ctrl Pts',(2.00225107134734,-1.,-0.509046069886157));
#37811=CARTESIAN_POINT('Ctrl Pts',(2.00225107134734,1.,-0.509046069886157));
#37812=CARTESIAN_POINT('Ctrl Pts',(2.00707309946949,-1.,-0.512953306961793));
#37813=CARTESIAN_POINT('Ctrl Pts',(2.00707309946949,1.,-0.512953306961793));
#37814=CARTESIAN_POINT('Ctrl Pts',(2.01187773939242,-1.,-0.516902681728687));
#37815=CARTESIAN_POINT('Ctrl Pts',(2.01187773939242,1.,-0.516902681728687));
#37816=CARTESIAN_POINT('Ctrl Pts',(2.01666477917286,-1.,-0.520893590399371));
#37817=CARTESIAN_POINT('Ctrl Pts',(2.01666477917286,1.,-0.520893590399371));
#37818=CARTESIAN_POINT('Ctrl Pts',(2.02143356304698,-1.,-0.524925318333476));
#37819=CARTESIAN_POINT('Ctrl Pts',(2.02143356304698,1.,-0.524925318333476));
#37820=CARTESIAN_POINT('Ctrl Pts',(2.0261832908329,-1.,-0.528997127241914));
#37821=CARTESIAN_POINT('Ctrl Pts',(2.0261832908329,1.,-0.528997127241914));
#37822=CARTESIAN_POINT('Ctrl Pts',(2.03091336214426,-1.,-0.533108355132977));
#37823=CARTESIAN_POINT('Ctrl Pts',(2.03091336214426,1.,-0.533108355132977));
#37824=CARTESIAN_POINT('Ctrl Pts',(2.03562362954037,-1.,-0.537258489833262));
#37825=CARTESIAN_POINT('Ctrl Pts',(2.03562362954037,1.,-0.537258489833262));
#37826=CARTESIAN_POINT('Ctrl Pts',(2.04031422690527,-1.,-0.541447120615659));
#37827=CARTESIAN_POINT('Ctrl Pts',(2.04031422690527,1.,-0.541447120615659));
#37828=CARTESIAN_POINT('Ctrl Pts',(2.04498544714588,-1.,-0.54567390381743));
#37829=CARTESIAN_POINT('Ctrl Pts',(2.04498544714588,1.,-0.54567390381743));
#37830=CARTESIAN_POINT('Ctrl Pts',(2.04963761077958,-1.,-0.549938525150295));
#37831=CARTESIAN_POINT('Ctrl Pts',(2.04963761077958,1.,-0.549938525150295));
#37832=CARTESIAN_POINT('Ctrl Pts',(2.05427091604413,-1.,-0.554240657463906));
#37833=CARTESIAN_POINT('Ctrl Pts',(2.05427091604413,1.,-0.554240657463906));
#37834=CARTESIAN_POINT('Ctrl Pts',(2.05888537756462,-1.,-0.558579940185152));
#37835=CARTESIAN_POINT('Ctrl Pts',(2.05888537756462,1.,-0.558579940185152));
#37836=CARTESIAN_POINT('Ctrl Pts',(2.06348090160589,-1.,-0.562955993082262));
#37837=CARTESIAN_POINT('Ctrl Pts',(2.06348090160589,1.,-0.562955993082262));
#37838=CARTESIAN_POINT('Ctrl Pts',(2.06805732997334,-1.,-0.567368421181087));
#37839=CARTESIAN_POINT('Ctrl Pts',(2.06805732997334,1.,-0.567368421181087));
#37840=CARTESIAN_POINT('Ctrl Pts',(2.07261449292824,-1.,-0.571816823242603));
#37841=CARTESIAN_POINT('Ctrl Pts',(2.07261449292824,1.,-0.571816823242603));
#37842=CARTESIAN_POINT('Ctrl Pts',(2.07715226767559,-1.,-0.576300797416845));
#37843=CARTESIAN_POINT('Ctrl Pts',(2.07715226767559,1.,-0.576300797416845));
#37844=CARTESIAN_POINT('Ctrl Pts',(2.08167059018418,-1.,-0.580819952108064));
#37845=CARTESIAN_POINT('Ctrl Pts',(2.08167059018418,1.,-0.580819952108064));
#37846=CARTESIAN_POINT('Ctrl Pts',(2.08616943727951,-1.,-0.585373918991617));
#37847=CARTESIAN_POINT('Ctrl Pts',(2.08616943727951,1.,-0.585373918991617));
#37848=CARTESIAN_POINT('Ctrl Pts',(2.09064881812129,-1.,-0.589962365403406));
#37849=CARTESIAN_POINT('Ctrl Pts',(2.09064881812129,1.,-0.589962365403406));
#37850=CARTESIAN_POINT('Ctrl Pts',(2.0951087622027,-1.,-0.594585006052162));
#37851=CARTESIAN_POINT('Ctrl Pts',(2.0951087622027,1.,-0.594585006052162));
#37852=CARTESIAN_POINT('Ctrl Pts',(2.0995493086477,-1.,-0.599241616420534));
#37853=CARTESIAN_POINT('Ctrl Pts',(2.0995493086477,1.,-0.599241616420534));
#37854=CARTESIAN_POINT('Ctrl Pts',(2.10397049886949,-1.,-0.60393203073603));
#37855=CARTESIAN_POINT('Ctrl Pts',(2.10397049886949,1.,-0.60393203073603));
#37856=CARTESIAN_POINT('Ctrl Pts',(2.1074919961518,-1.,-0.607711315454876));
#37857=CARTESIAN_POINT('Ctrl Pts',(2.1074919961518,1.,-0.607711315454876));
#37858=CARTESIAN_POINT('Ctrl Pts',(2.11012443807238,-1.,-0.610560911689899));
#37859=CARTESIAN_POINT('Ctrl Pts',(2.11012443807238,1.,-0.610560911689899));
#37860=CARTESIAN_POINT('Ctrl Pts',(2.11187554259986,-1.,-0.6124673655618));
#37861=CARTESIAN_POINT('Ctrl Pts',(2.11187554259986,1.,-0.6124673655618));
#37862=CARTESIAN_POINT('Ctrl Pts',(2.11275013067528,-1.,-0.61342227326009));
#37863=CARTESIAN_POINT('Ctrl Pts',(2.11275013067528,1.,-0.61342227326009));
#37864=CARTESIAN_POINT('',(1.7075470150345,1.,-0.383122945602004));
#37865=CARTESIAN_POINT('Ctrl Pts',(1.7075470150345,1.,-0.383122945602004));
#37866=CARTESIAN_POINT('Ctrl Pts',(1.71231062891958,1.,-0.384119047315542));
#37867=CARTESIAN_POINT('Ctrl Pts',(1.72162022246158,1.,-0.38607079032701));
#37868=CARTESIAN_POINT('Ctrl Pts',(1.7349317097561,1.,-0.388877023509192));
#37869=CARTESIAN_POINT('Ctrl Pts',(1.75137405313962,1.,-0.392375812294307));
#37870=CARTESIAN_POINT('Ctrl Pts',(1.7697556004756,1.,-0.39634619612042));
#37871=CARTESIAN_POINT('Ctrl Pts',(1.78598826347533,1.,-0.399919403783081));
#37872=CARTESIAN_POINT('Ctrl Pts',(1.80012077176221,1.,-0.403107976170441));
#37873=CARTESIAN_POINT('Ctrl Pts',(1.81223801813988,1.,-0.405933518411838));
#37874=CARTESIAN_POINT('Ctrl Pts',(1.8224702267854,1.,-0.408428948108534));
#37875=CARTESIAN_POINT('Ctrl Pts',(1.83100408895216,1.,-0.410641256301675));
#37876=CARTESIAN_POINT('Ctrl Pts',(1.83808953475839,1.,-0.412633125322162));
#37877=CARTESIAN_POINT('Ctrl Pts',(1.8440575707371,1.,-0.41448743825434));
#37878=CARTESIAN_POINT('Ctrl Pts',(1.84929312929882,1.,-0.416300022038864));
#37879=CARTESIAN_POINT('Ctrl Pts',(1.85417632856234,1.,-0.418164129143534));
#37880=CARTESIAN_POINT('Ctrl Pts',(1.85903281096686,1.,-0.42015728797562));
#37881=CARTESIAN_POINT('Ctrl Pts',(1.86408083334028,1.,-0.422327307418275));
#37882=CARTESIAN_POINT('Ctrl Pts',(1.86937803944323,1.,-0.424678177291359));
#37883=CARTESIAN_POINT('Ctrl Pts',(1.87486989291484,1.,-0.427183828519102));
#37884=CARTESIAN_POINT('Ctrl Pts',(1.88044229001832,1.,-0.429803062482345));
#37885=CARTESIAN_POINT('Ctrl Pts',(1.88596913666793,1.,-0.432493038548748));
#37886=CARTESIAN_POINT('Ctrl Pts',(1.89136993975504,1.,-0.435225660963383));
#37887=CARTESIAN_POINT('Ctrl Pts',(1.89663648956466,1.,-0.437995003948244));
#37888=CARTESIAN_POINT('Ctrl Pts',(1.90180124389086,1.,-0.440807833704038));
#37889=CARTESIAN_POINT('Ctrl Pts',(1.90691756144898,1.,-0.443677556849151));
#37890=CARTESIAN_POINT('Ctrl Pts',(1.9120369998112,1.,-0.446617343485711));
#37891=CARTESIAN_POINT('Ctrl Pts',(1.91718342555755,1.,-0.449632260106662));
#37892=CARTESIAN_POINT('Ctrl Pts',(1.92235380648502,1.,-0.452719478359433));
#37893=CARTESIAN_POINT('Ctrl Pts',(1.92753067150476,1.,-0.455872005174371));
#37894=CARTESIAN_POINT('Ctrl Pts',(1.93269066517934,1.,-0.459081234547926));
#37895=CARTESIAN_POINT('Ctrl Pts',(1.93781486640821,1.,-0.462340031009057));
#37896=CARTESIAN_POINT('Ctrl Pts',(1.9428979419619,1.,-0.46564546202603));
#37897=CARTESIAN_POINT('Ctrl Pts',(1.94794381136514,1.,-0.468997482913135));
#37898=CARTESIAN_POINT('Ctrl Pts',(1.95296148278133,1.,-0.472397672264072));
#37899=CARTESIAN_POINT('Ctrl Pts',(1.95796111148177,1.,-0.475848034683176));
#37900=CARTESIAN_POINT('Ctrl Pts',(1.96294933055943,1.,-0.479349583074855));
#37901=CARTESIAN_POINT('Ctrl Pts',(1.96792703422362,1.,-0.482901662120691));
#37902=CARTESIAN_POINT('Ctrl Pts',(1.97289186263272,1.,-0.486502692907659));
#37903=CARTESIAN_POINT('Ctrl Pts',(1.97783973019229,1.,-0.490150627860953));
#37904=CARTESIAN_POINT('Ctrl Pts',(1.98276658761821,1.,-0.493843476541495));
#37905=CARTESIAN_POINT('Ctrl Pts',(1.98767044752932,1.,-0.497579909545574));
#37906=CARTESIAN_POINT('Ctrl Pts',(1.99255149126155,1.,-0.501359287727146));
#37907=CARTESIAN_POINT('Ctrl Pts',(1.99741107463572,1.,-0.505181361323026));
#37908=CARTESIAN_POINT('Ctrl Pts',(2.00225107134734,1.,-0.509046069886157));
#37909=CARTESIAN_POINT('Ctrl Pts',(2.00707309946949,1.,-0.512953306961793));
#37910=CARTESIAN_POINT('Ctrl Pts',(2.01187773939242,1.,-0.516902681728687));
#37911=CARTESIAN_POINT('Ctrl Pts',(2.01666477917286,1.,-0.520893590399371));
#37912=CARTESIAN_POINT('Ctrl Pts',(2.02143356304698,1.,-0.524925318333476));
#37913=CARTESIAN_POINT('Ctrl Pts',(2.0261832908329,1.,-0.528997127241914));
#37914=CARTESIAN_POINT('Ctrl Pts',(2.03091336214426,1.,-0.533108355132977));
#37915=CARTESIAN_POINT('Ctrl Pts',(2.03562362954037,1.,-0.537258489833262));
#37916=CARTESIAN_POINT('Ctrl Pts',(2.04031422690527,1.,-0.541447120615659));
#37917=CARTESIAN_POINT('Ctrl Pts',(2.04498544714588,1.,-0.54567390381743));
#37918=CARTESIAN_POINT('Ctrl Pts',(2.04963761077958,1.,-0.549938525150295));
#37919=CARTESIAN_POINT('Ctrl Pts',(2.05427091604413,1.,-0.554240657463906));
#37920=CARTESIAN_POINT('Ctrl Pts',(2.05888537756462,1.,-0.558579940185152));
#37921=CARTESIAN_POINT('Ctrl Pts',(2.06348090160589,1.,-0.562955993082262));
#37922=CARTESIAN_POINT('Ctrl Pts',(2.06805732997334,1.,-0.567368421181087));
#37923=CARTESIAN_POINT('Ctrl Pts',(2.07261449292824,1.,-0.571816823242603));
#37924=CARTESIAN_POINT('Ctrl Pts',(2.07715226767559,1.,-0.576300797416845));
#37925=CARTESIAN_POINT('Ctrl Pts',(2.08167059018418,1.,-0.580819952108064));
#37926=CARTESIAN_POINT('Ctrl Pts',(2.08616943727951,1.,-0.585373918991617));
#37927=CARTESIAN_POINT('Ctrl Pts',(2.09064881812129,1.,-0.589962365403406));
#37928=CARTESIAN_POINT('Ctrl Pts',(2.0951087622027,1.,-0.594585006052162));
#37929=CARTESIAN_POINT('Ctrl Pts',(2.0995493086477,1.,-0.599241616420534));
#37930=CARTESIAN_POINT('Ctrl Pts',(2.10397049886949,1.,-0.60393203073603));
#37931=CARTESIAN_POINT('Ctrl Pts',(2.1074919961518,1.,-0.607711315454876));
#37932=CARTESIAN_POINT('Ctrl Pts',(2.11012443807238,1.,-0.610560911689899));
#37933=CARTESIAN_POINT('Ctrl Pts',(2.11187554259986,1.,-0.6124673655618));
#37934=CARTESIAN_POINT('Ctrl Pts',(2.11275013067528,1.,-0.61342227326009));
#37935=CARTESIAN_POINT('',(1.7075470150345,0.,-0.383122945602001));
#37936=CARTESIAN_POINT('Origin',(0.,0.,0.));
#37937=CARTESIAN_POINT('',(1.74236521665491,1.,-0.163289472382896));
#37938=CARTESIAN_POINT('Origin',(0.,1.,0.));
#37939=CARTESIAN_POINT('',(1.74236521665491,0.,-0.163289472382896));
#37940=CARTESIAN_POINT('Ctrl Pts',(2.19890268624765,-1.,-0.0694764450219582));
#37941=CARTESIAN_POINT('Ctrl Pts',(2.19890268624765,1.,-0.0694764450219582));
#37942=CARTESIAN_POINT('Ctrl Pts',(2.19777582085423,-1.,-0.0701143536325491));
#37943=CARTESIAN_POINT('Ctrl Pts',(2.19777582085423,1.,-0.0701143536325491));
#37944=CARTESIAN_POINT('Ctrl Pts',(2.19552129484002,-1.,-0.0713863779526155));
#37945=CARTESIAN_POINT('Ctrl Pts',(2.19552129484002,1.,-0.0713863779526155));
#37946=CARTESIAN_POINT('Ctrl Pts',(2.19213712013662,-1.,-0.0732830357306726));
#37947=CARTESIAN_POINT('Ctrl Pts',(2.19213712013662,1.,-0.0732830357306726));
#37948=CARTESIAN_POINT('Ctrl Pts',(2.1876201139953,-1.,-0.0757891465836149));
#37949=CARTESIAN_POINT('Ctrl Pts',(2.1876201139953,1.,-0.0757891465836149));
#37950=CARTESIAN_POINT('Ctrl Pts',(2.18196589448887,-1.,-0.0788837727685244));
#37951=CARTESIAN_POINT('Ctrl Pts',(2.18196589448887,1.,-0.0788837727685244));
#37952=CARTESIAN_POINT('Ctrl Pts',(2.176303712113,-1.,-0.0819402680872767));
#37953=CARTESIAN_POINT('Ctrl Pts',(2.176303712113,1.,-0.0819402680872767));
#37954=CARTESIAN_POINT('Ctrl Pts',(2.17063357870952,-1.,-0.0849584620835374));
#37955=CARTESIAN_POINT('Ctrl Pts',(2.17063357870952,1.,-0.0849584620835374));
#37956=CARTESIAN_POINT('Ctrl Pts',(2.16495552645014,-1.,-0.0879381291386924));
#37957=CARTESIAN_POINT('Ctrl Pts',(2.16495552645014,1.,-0.0879381291386924));
#37958=CARTESIAN_POINT('Ctrl Pts',(2.15926961544516,-1.,-0.0908789888107267));
#37959=CARTESIAN_POINT('Ctrl Pts',(2.15926961544516,1.,-0.0908789888107267));
#37960=CARTESIAN_POINT('Ctrl Pts',(2.1535759397817,-1.,-0.0937807218867645));
#37961=CARTESIAN_POINT('Ctrl Pts',(2.1535759397817,1.,-0.0937807218867645));
#37962=CARTESIAN_POINT('Ctrl Pts',(2.14787463531795,-1.,-0.096642985230546));
#37963=CARTESIAN_POINT('Ctrl Pts',(2.14787463531795,1.,-0.096642985230546));
#37964=CARTESIAN_POINT('Ctrl Pts',(2.14216588396025,-1.,-0.0994654261990917));
#37965=CARTESIAN_POINT('Ctrl Pts',(2.14216588396025,1.,-0.0994654261990917));
#37966=CARTESIAN_POINT('Ctrl Pts',(2.13644992667165,-1.,-0.102247700556101));
#37967=CARTESIAN_POINT('Ctrl Pts',(2.13644992667165,1.,-0.102247700556101));
#37968=CARTESIAN_POINT('Ctrl Pts',(2.13072704887293,-1.,-0.10498947915274));
#37969=CARTESIAN_POINT('Ctrl Pts',(2.13072704887293,1.,-0.10498947915274));
#37970=CARTESIAN_POINT('Ctrl Pts',(2.12499752307,-1.,-0.10769043523109));
#37971=CARTESIAN_POINT('Ctrl Pts',(2.12499752307,1.,-0.10769043523109));
#37972=CARTESIAN_POINT('Ctrl Pts',(2.11926155590865,-1.,-0.110350236135025));
#37973=CARTESIAN_POINT('Ctrl Pts',(2.11926155590865,1.,-0.110350236135025));
#37974=CARTESIAN_POINT('Ctrl Pts',(2.11351924490306,-1.,-0.112968534419737));
#37975=CARTESIAN_POINT('Ctrl Pts',(2.11351924490306,1.,-0.112968534419737));
#37976=CARTESIAN_POINT('Ctrl Pts',(2.10777050261309,-1.,-0.115544957687927));
#37977=CARTESIAN_POINT('Ctrl Pts',(2.10777050261309,1.,-0.115544957687927));
#37978=CARTESIAN_POINT('Ctrl Pts',(2.102015121329,-1.,-0.118079107988356));
#37979=CARTESIAN_POINT('Ctrl Pts',(2.102015121329,1.,-0.118079107988356));
#37980=CARTESIAN_POINT('Ctrl Pts',(2.0962529286773,-1.,-0.120570567965122));
#37981=CARTESIAN_POINT('Ctrl Pts',(2.0962529286773,1.,-0.120570567965122));
#37982=CARTESIAN_POINT('Ctrl Pts',(2.09048392424825,-1.,-0.123018905621083));
#37983=CARTESIAN_POINT('Ctrl Pts',(2.09048392424825,1.,-0.123018905621083));
#37984=CARTESIAN_POINT('Ctrl Pts',(2.08470840653643,-1.,-0.125423679412062));
#37985=CARTESIAN_POINT('Ctrl Pts',(2.08470840653643,1.,-0.125423679412062));
#37986=CARTESIAN_POINT('Ctrl Pts',(2.07892715110987,-1.,-0.12778444527612));
#37987=CARTESIAN_POINT('Ctrl Pts',(2.07892715110987,1.,-0.12778444527612));
#37988=CARTESIAN_POINT('Ctrl Pts',(2.07314114713063,-1.,-0.130100748328404));
#37989=CARTESIAN_POINT('Ctrl Pts',(2.07314114713063,1.,-0.130100748328404));
#37990=CARTESIAN_POINT('Ctrl Pts',(2.06735123910326,-1.,-0.132372111547711));
#37991=CARTESIAN_POINT('Ctrl Pts',(2.06735123910326,1.,-0.132372111547711));
#37992=CARTESIAN_POINT('Ctrl Pts',(2.06155781517842,-1.,-0.134598026192106));
#37993=CARTESIAN_POINT('Ctrl Pts',(2.06155781517842,1.,-0.134598026192106));
#37994=CARTESIAN_POINT('Ctrl Pts',(2.05576044414264,-1.,-0.136777941218044));
#37995=CARTESIAN_POINT('Ctrl Pts',(2.05576044414264,1.,-0.136777941218044));
#37996=CARTESIAN_POINT('Ctrl Pts',(2.04995762001328,-1.,-0.138911255368966));
#37997=CARTESIAN_POINT('Ctrl Pts',(2.04995762001328,1.,-0.138911255368966));
#37998=CARTESIAN_POINT('Ctrl Pts',(2.04414757947916,-1.,-0.140997332152546));
#37999=CARTESIAN_POINT('Ctrl Pts',(2.04414757947916,1.,-0.140997332152546));
#38000=CARTESIAN_POINT('Ctrl Pts',(2.03832911025912,-1.,-0.143035515058209));
#38001=CARTESIAN_POINT('Ctrl Pts',(2.03832911025912,1.,-0.143035515058209));
#38002=CARTESIAN_POINT('Ctrl Pts',(2.03250223739942,-1.,-0.145025140186058));
#38003=CARTESIAN_POINT('Ctrl Pts',(2.03250223739942,1.,-0.145025140186058));
#38004=CARTESIAN_POINT('Ctrl Pts',(2.02666926182017,-1.,-0.146965557332583));
#38005=CARTESIAN_POINT('Ctrl Pts',(2.02666926182017,1.,-0.146965557332583));
#38006=CARTESIAN_POINT('Ctrl Pts',(2.02083464969894,-1.,-0.148856124775337));
#38007=CARTESIAN_POINT('Ctrl Pts',(2.02083464969894,1.,-0.148856124775337));
#38008=CARTESIAN_POINT('Ctrl Pts',(2.01500291940238,-1.,-0.150696157673078));
#38009=CARTESIAN_POINT('Ctrl Pts',(2.01500291940238,1.,-0.150696157673078));
#38010=CARTESIAN_POINT('Ctrl Pts',(2.00917680318424,-1.,-0.15248488362145));
#38011=CARTESIAN_POINT('Ctrl Pts',(2.00917680318424,1.,-0.15248488362145));
#38012=CARTESIAN_POINT('Ctrl Pts',(2.00335565310543,-1.,-0.154221403049722));
#38013=CARTESIAN_POINT('Ctrl Pts',(2.00335565310543,1.,-0.154221403049722));
#38014=CARTESIAN_POINT('Ctrl Pts',(1.99753284771497,-1.,-0.155904629548784));
#38015=CARTESIAN_POINT('Ctrl Pts',(1.99753284771497,1.,-0.155904629548784));
#38016=CARTESIAN_POINT('Ctrl Pts',(1.99169810931908,-1.,-0.157533331459227));
#38017=CARTESIAN_POINT('Ctrl Pts',(1.99169810931908,1.,-0.157533331459227));
#38018=CARTESIAN_POINT('Ctrl Pts',(1.98584238283292,-1.,-0.159106226437299));
#38019=CARTESIAN_POINT('Ctrl Pts',(1.98584238283292,1.,-0.159106226437299));
#38020=CARTESIAN_POINT('Ctrl Pts',(1.97996195437559,-1.,-0.160622060784611));
#38021=CARTESIAN_POINT('Ctrl Pts',(1.97996195437559,1.,-0.160622060784611));
#38022=CARTESIAN_POINT('Ctrl Pts',(1.97406280235188,-1.,-0.162079693556289));
#38023=CARTESIAN_POINT('Ctrl Pts',(1.97406280235188,1.,-0.162079693556289));
#38024=CARTESIAN_POINT('Ctrl Pts',(1.96816512677967,-1.,-0.163478185457734));
#38025=CARTESIAN_POINT('Ctrl Pts',(1.96816512677967,1.,-0.163478185457734));
#38026=CARTESIAN_POINT('Ctrl Pts',(1.96229379940136,-1.,-0.164816568920269));
#38027=CARTESIAN_POINT('Ctrl Pts',(1.96229379940136,1.,-0.164816568920269));
#38028=CARTESIAN_POINT('Ctrl Pts',(1.9564675971873,-1.,-0.166093592002813));
#38029=CARTESIAN_POINT('Ctrl Pts',(1.9564675971873,1.,-0.166093592002813));
#38030=CARTESIAN_POINT('Ctrl Pts',(1.95069027794294,-1.,-0.167307501784476));
#38031=CARTESIAN_POINT('Ctrl Pts',(1.95069027794294,1.,-0.167307501784476));
#38032=CARTESIAN_POINT('Ctrl Pts',(1.94493757756931,-1.,-0.168455741607556));
#38033=CARTESIAN_POINT('Ctrl Pts',(1.94493757756931,1.,-0.168455741607556));
#38034=CARTESIAN_POINT('Ctrl Pts',(1.93915639211581,-1.,-0.169534904817491));
#38035=CARTESIAN_POINT('Ctrl Pts',(1.93915639211581,1.,-0.169534904817491));
#38036=CARTESIAN_POINT('Ctrl Pts',(1.93329183155539,-1.,-0.170541253116202));
#38037=CARTESIAN_POINT('Ctrl Pts',(1.93329183155539,1.,-0.170541253116202));
#38038=CARTESIAN_POINT('Ctrl Pts',(1.92731093582036,-1.,-0.171471191532988));
#38039=CARTESIAN_POINT('Ctrl Pts',(1.92731093582036,1.,-0.171471191532988));
#38040=CARTESIAN_POINT('Ctrl Pts',(1.9212233439798,-1.,-0.172321621259514));
#38041=CARTESIAN_POINT('Ctrl Pts',(1.9212233439798,1.,-0.172321621259514));
#38042=CARTESIAN_POINT('Ctrl Pts',(1.91511429159527,-1.,-0.173090695383496));
#38043=CARTESIAN_POINT('Ctrl Pts',(1.91511429159527,1.,-0.173090695383496));
#38044=CARTESIAN_POINT('Ctrl Pts',(1.90911693975267,-1.,-0.173776635257817));
#38045=CARTESIAN_POINT('Ctrl Pts',(1.90911693975267,1.,-0.173776635257817));
#38046=CARTESIAN_POINT('Ctrl Pts',(1.90335253862834,-1.,-0.174375518661085));
#38047=CARTESIAN_POINT('Ctrl Pts',(1.90335253862834,1.,-0.174375518661085));
#38048=CARTESIAN_POINT('Ctrl Pts',(1.89788101117132,-1.,-0.174879405091263));
#38049=CARTESIAN_POINT('Ctrl Pts',(1.89788101117132,1.,-0.174879405091263));
#38050=CARTESIAN_POINT('Ctrl Pts',(1.892646301985,-1.,-0.175274276190844));
#38051=CARTESIAN_POINT('Ctrl Pts',(1.892646301985,1.,-0.175274276190844));
#38052=CARTESIAN_POINT('Ctrl Pts',(1.88742606273259,-1.,-0.175538155840648));
#38053=CARTESIAN_POINT('Ctrl Pts',(1.88742606273259,1.,-0.175538155840648));
#38054=CARTESIAN_POINT('Ctrl Pts',(1.88188663145367,-1.,-0.175644148889699));
#38055=CARTESIAN_POINT('Ctrl Pts',(1.88188663145367,1.,-0.175644148889699));
#38056=CARTESIAN_POINT('Ctrl Pts',(1.87563767773588,-1.,-0.175563480746485));
#38057=CARTESIAN_POINT('Ctrl Pts',(1.87563767773588,1.,-0.175563480746485));
#38058=CARTESIAN_POINT('Ctrl Pts',(1.86828349694799,-1.,-0.175268337590758));
#38059=CARTESIAN_POINT('Ctrl Pts',(1.86828349694799,1.,-0.175268337590758));
#38060=CARTESIAN_POINT('Ctrl Pts',(1.85948367088837,-1.,-0.17473525927603));
#38061=CARTESIAN_POINT('Ctrl Pts',(1.85948367088837,1.,-0.17473525927603));
#38062=CARTESIAN_POINT('Ctrl Pts',(1.8489811319852,-1.,-0.173946627587732));
#38063=CARTESIAN_POINT('Ctrl Pts',(1.8489811319852,1.,-0.173946627587732));
#38064=CARTESIAN_POINT('Ctrl Pts',(1.83658380527692,-1.,-0.1728894428919));
#38065=CARTESIAN_POINT('Ctrl Pts',(1.83658380527692,1.,-0.1728894428919));
#38066=CARTESIAN_POINT('Ctrl Pts',(1.82215766811545,-1.,-0.171554770204119));
#38067=CARTESIAN_POINT('Ctrl Pts',(1.82215766811545,1.,-0.171554770204119));
#38068=CARTESIAN_POINT('Ctrl Pts',(1.80561530629706,-1.,-0.169936923904608));
#38069=CARTESIAN_POINT('Ctrl Pts',(1.80561530629706,1.,-0.169936923904608));
#38070=CARTESIAN_POINT('Ctrl Pts',(1.7869064998507,-1.,-0.168032772805197));
#38071=CARTESIAN_POINT('Ctrl Pts',(1.7869064998507,1.,-0.168032772805197));
#38072=CARTESIAN_POINT('Ctrl Pts',(1.77018771684844,-1.,-0.1662793551464));
#38073=CARTESIAN_POINT('Ctrl Pts',(1.77018771684844,1.,-0.1662793551464));
#38074=CARTESIAN_POINT('Ctrl Pts',(1.75666056638427,-1.,-0.164834765707159));
#38075=CARTESIAN_POINT('Ctrl Pts',(1.75666056638427,1.,-0.164834765707159));
#38076=CARTESIAN_POINT('Ctrl Pts',(1.7472034950333,-1.,-0.163814161002002));
#38077=CARTESIAN_POINT('Ctrl Pts',(1.7472034950333,1.,-0.163814161002002));
#38078=CARTESIAN_POINT('Ctrl Pts',(1.74236521665491,-1.,-0.163289472382896));
#38079=CARTESIAN_POINT('Ctrl Pts',(1.74236521665491,1.,-0.163289472382896));
#38080=CARTESIAN_POINT('',(2.19890268624765,1.,-0.0694764450219582));
#38081=CARTESIAN_POINT('Ctrl Pts',(2.19890268624765,1.,-0.0694764450219582));
#38082=CARTESIAN_POINT('Ctrl Pts',(2.19777582085423,1.,-0.0701143536325491));
#38083=CARTESIAN_POINT('Ctrl Pts',(2.19552129484002,1.,-0.0713863779526155));
#38084=CARTESIAN_POINT('Ctrl Pts',(2.19213712013662,1.,-0.0732830357306726));
#38085=CARTESIAN_POINT('Ctrl Pts',(2.1876201139953,1.,-0.0757891465836149));
#38086=CARTESIAN_POINT('Ctrl Pts',(2.18196589448887,1.,-0.0788837727685244));
#38087=CARTESIAN_POINT('Ctrl Pts',(2.176303712113,1.,-0.0819402680872767));
#38088=CARTESIAN_POINT('Ctrl Pts',(2.17063357870952,1.,-0.0849584620835374));
#38089=CARTESIAN_POINT('Ctrl Pts',(2.16495552645014,1.,-0.0879381291386924));
#38090=CARTESIAN_POINT('Ctrl Pts',(2.15926961544516,1.,-0.0908789888107267));
#38091=CARTESIAN_POINT('Ctrl Pts',(2.1535759397817,1.,-0.0937807218867645));
#38092=CARTESIAN_POINT('Ctrl Pts',(2.14787463531795,1.,-0.096642985230546));
#38093=CARTESIAN_POINT('Ctrl Pts',(2.14216588396025,1.,-0.0994654261990917));
#38094=CARTESIAN_POINT('Ctrl Pts',(2.13644992667165,1.,-0.102247700556101));
#38095=CARTESIAN_POINT('Ctrl Pts',(2.13072704887293,1.,-0.10498947915274));
#38096=CARTESIAN_POINT('Ctrl Pts',(2.12499752307,1.,-0.10769043523109));
#38097=CARTESIAN_POINT('Ctrl Pts',(2.11926155590865,1.,-0.110350236135025));
#38098=CARTESIAN_POINT('Ctrl Pts',(2.11351924490306,1.,-0.112968534419737));
#38099=CARTESIAN_POINT('Ctrl Pts',(2.10777050261309,1.,-0.115544957687927));
#38100=CARTESIAN_POINT('Ctrl Pts',(2.102015121329,1.,-0.118079107988356));
#38101=CARTESIAN_POINT('Ctrl Pts',(2.0962529286773,1.,-0.120570567965122));
#38102=CARTESIAN_POINT('Ctrl Pts',(2.09048392424825,1.,-0.123018905621083));
#38103=CARTESIAN_POINT('Ctrl Pts',(2.08470840653643,1.,-0.125423679412062));
#38104=CARTESIAN_POINT('Ctrl Pts',(2.07892715110987,1.,-0.12778444527612));
#38105=CARTESIAN_POINT('Ctrl Pts',(2.07314114713063,1.,-0.130100748328404));
#38106=CARTESIAN_POINT('Ctrl Pts',(2.06735123910326,1.,-0.132372111547711));
#38107=CARTESIAN_POINT('Ctrl Pts',(2.06155781517842,1.,-0.134598026192106));
#38108=CARTESIAN_POINT('Ctrl Pts',(2.05576044414264,1.,-0.136777941218044));
#38109=CARTESIAN_POINT('Ctrl Pts',(2.04995762001328,1.,-0.138911255368966));
#38110=CARTESIAN_POINT('Ctrl Pts',(2.04414757947916,1.,-0.140997332152546));
#38111=CARTESIAN_POINT('Ctrl Pts',(2.03832911025912,1.,-0.143035515058209));
#38112=CARTESIAN_POINT('Ctrl Pts',(2.03250223739942,1.,-0.145025140186058));
#38113=CARTESIAN_POINT('Ctrl Pts',(2.02666926182017,1.,-0.146965557332583));
#38114=CARTESIAN_POINT('Ctrl Pts',(2.02083464969894,1.,-0.148856124775337));
#38115=CARTESIAN_POINT('Ctrl Pts',(2.01500291940238,1.,-0.150696157673078));
#38116=CARTESIAN_POINT('Ctrl Pts',(2.00917680318424,1.,-0.15248488362145));
#38117=CARTESIAN_POINT('Ctrl Pts',(2.00335565310543,1.,-0.154221403049722));
#38118=CARTESIAN_POINT('Ctrl Pts',(1.99753284771497,1.,-0.155904629548784));
#38119=CARTESIAN_POINT('Ctrl Pts',(1.99169810931908,1.,-0.157533331459227));
#38120=CARTESIAN_POINT('Ctrl Pts',(1.98584238283292,1.,-0.159106226437299));
#38121=CARTESIAN_POINT('Ctrl Pts',(1.97996195437559,1.,-0.160622060784611));
#38122=CARTESIAN_POINT('Ctrl Pts',(1.97406280235188,1.,-0.162079693556289));
#38123=CARTESIAN_POINT('Ctrl Pts',(1.96816512677967,1.,-0.163478185457734));
#38124=CARTESIAN_POINT('Ctrl Pts',(1.96229379940136,1.,-0.164816568920269));
#38125=CARTESIAN_POINT('Ctrl Pts',(1.9564675971873,1.,-0.166093592002813));
#38126=CARTESIAN_POINT('Ctrl Pts',(1.95069027794294,1.,-0.167307501784476));
#38127=CARTESIAN_POINT('Ctrl Pts',(1.94493757756931,1.,-0.168455741607556));
#38128=CARTESIAN_POINT('Ctrl Pts',(1.93915639211581,1.,-0.169534904817491));
#38129=CARTESIAN_POINT('Ctrl Pts',(1.93329183155539,1.,-0.170541253116202));
#38130=CARTESIAN_POINT('Ctrl Pts',(1.92731093582036,1.,-0.171471191532988));
#38131=CARTESIAN_POINT('Ctrl Pts',(1.9212233439798,1.,-0.172321621259514));
#38132=CARTESIAN_POINT('Ctrl Pts',(1.91511429159527,1.,-0.173090695383496));
#38133=CARTESIAN_POINT('Ctrl Pts',(1.90911693975267,1.,-0.173776635257817));
#38134=CARTESIAN_POINT('Ctrl Pts',(1.90335253862834,1.,-0.174375518661085));
#38135=CARTESIAN_POINT('Ctrl Pts',(1.89788101117132,1.,-0.174879405091263));
#38136=CARTESIAN_POINT('Ctrl Pts',(1.892646301985,1.,-0.175274276190844));
#38137=CARTESIAN_POINT('Ctrl Pts',(1.88742606273259,1.,-0.175538155840648));
#38138=CARTESIAN_POINT('Ctrl Pts',(1.88188663145367,1.,-0.175644148889699));
#38139=CARTESIAN_POINT('Ctrl Pts',(1.87563767773588,1.,-0.175563480746485));
#38140=CARTESIAN_POINT('Ctrl Pts',(1.86828349694799,1.,-0.175268337590758));
#38141=CARTESIAN_POINT('Ctrl Pts',(1.85948367088837,1.,-0.17473525927603));
#38142=CARTESIAN_POINT('Ctrl Pts',(1.8489811319852,1.,-0.173946627587732));
#38143=CARTESIAN_POINT('Ctrl Pts',(1.83658380527692,1.,-0.1728894428919));
#38144=CARTESIAN_POINT('Ctrl Pts',(1.82215766811545,1.,-0.171554770204119));
#38145=CARTESIAN_POINT('Ctrl Pts',(1.80561530629706,1.,-0.169936923904608));
#38146=CARTESIAN_POINT('Ctrl Pts',(1.7869064998507,1.,-0.168032772805197));
#38147=CARTESIAN_POINT('Ctrl Pts',(1.77018771684844,1.,-0.1662793551464));
#38148=CARTESIAN_POINT('Ctrl Pts',(1.75666056638427,1.,-0.164834765707159));
#38149=CARTESIAN_POINT('Ctrl Pts',(1.7472034950333,1.,-0.163814161002002));
#38150=CARTESIAN_POINT('Ctrl Pts',(1.74236521665491,1.,-0.163289472382896));
#38151=CARTESIAN_POINT('',(2.19890268624765,0.,-0.0694764450219582));
#38152=CARTESIAN_POINT('Origin',(2.19890268624765,0.,0.0694764450219582));
#38153=CARTESIAN_POINT('',(2.19890268624765,1.,0.0694764450219582));
#38154=CARTESIAN_POINT('',(2.19890268624765,1.,-0.0694764450219582));
#38155=CARTESIAN_POINT('',(2.19890268624765,0.,0.0694764450219582));
#38156=CARTESIAN_POINT('Ctrl Pts',(1.74236521665491,-1.,0.163289472382896));
#38157=CARTESIAN_POINT('Ctrl Pts',(1.74236521665491,1.,0.163289472382896));
#38158=CARTESIAN_POINT('Ctrl Pts',(1.74720349503904,-1.,0.163814161002474));
#38159=CARTESIAN_POINT('Ctrl Pts',(1.74720349503904,1.,0.163814161002474));
#38160=CARTESIAN_POINT('Ctrl Pts',(1.75666056640041,-1.,0.164834765708484));
#38161=CARTESIAN_POINT('Ctrl Pts',(1.75666056640041,1.,0.164834765708484));
#38162=CARTESIAN_POINT('Ctrl Pts',(1.77018771687692,-1.,0.166279355148738));
#38163=CARTESIAN_POINT('Ctrl Pts',(1.77018771687692,1.,0.166279355148738));
#38164=CARTESIAN_POINT('Ctrl Pts',(1.78690649988931,-1.,0.16803277280837));
#38165=CARTESIAN_POINT('Ctrl Pts',(1.78690649988931,1.,0.16803277280837));
#38166=CARTESIAN_POINT('Ctrl Pts',(1.80561530633924,-1.,0.169936923908078));
#38167=CARTESIAN_POINT('Ctrl Pts',(1.80561530633924,1.,0.169936923908078));
#38168=CARTESIAN_POINT('Ctrl Pts',(1.82215766815414,-1.,0.171554770207306));
#38169=CARTESIAN_POINT('Ctrl Pts',(1.82215766815414,1.,0.171554770207306));
#38170=CARTESIAN_POINT('Ctrl Pts',(1.83658380530747,-1.,0.17288944289442));
#38171=CARTESIAN_POINT('Ctrl Pts',(1.83658380530747,1.,0.17288944289442));
#38172=CARTESIAN_POINT('Ctrl Pts',(1.84898113200543,-1.,0.173946627589401));
#38173=CARTESIAN_POINT('Ctrl Pts',(1.84898113200543,1.,0.173946627589401));
#38174=CARTESIAN_POINT('Ctrl Pts',(1.85948367089838,-1.,0.174735259276856));
#38175=CARTESIAN_POINT('Ctrl Pts',(1.85948367089838,1.,0.174735259276856));
#38176=CARTESIAN_POINT('Ctrl Pts',(1.86828349694972,-1.,0.1752683375909));
#38177=CARTESIAN_POINT('Ctrl Pts',(1.86828349694972,1.,0.1752683375909));
#38178=CARTESIAN_POINT('Ctrl Pts',(1.87563767773249,-1.,0.175563480746205));
#38179=CARTESIAN_POINT('Ctrl Pts',(1.87563767773249,1.,0.175563480746205));
#38180=CARTESIAN_POINT('Ctrl Pts',(1.88188663144846,-1.,0.175644148889271));
#38181=CARTESIAN_POINT('Ctrl Pts',(1.88188663144846,1.,0.175644148889271));
#38182=CARTESIAN_POINT('Ctrl Pts',(1.88742606272818,-1.,0.175538155840286));
#38183=CARTESIAN_POINT('Ctrl Pts',(1.88742606272818,1.,0.175538155840286));
#38184=CARTESIAN_POINT('Ctrl Pts',(1.89264630198279,-1.,0.175274276190664));
#38185=CARTESIAN_POINT('Ctrl Pts',(1.89264630198279,1.,0.175274276190664));
#38186=CARTESIAN_POINT('Ctrl Pts',(1.89788101117148,-1.,0.174879405091277));
#38187=CARTESIAN_POINT('Ctrl Pts',(1.89788101117148,1.,0.174879405091277));
#38188=CARTESIAN_POINT('Ctrl Pts',(1.90335253863003,-1.,0.174375518661222));
#38189=CARTESIAN_POINT('Ctrl Pts',(1.90335253863003,1.,0.174375518661222));
#38190=CARTESIAN_POINT('Ctrl Pts',(1.90911693975475,-1.,0.173776635257983));
#38191=CARTESIAN_POINT('Ctrl Pts',(1.90911693975475,1.,0.173776635257983));
#38192=CARTESIAN_POINT('Ctrl Pts',(1.91511429159681,-1.,0.173090695383619));
#38193=CARTESIAN_POINT('Ctrl Pts',(1.91511429159681,1.,0.173090695383619));
#38194=CARTESIAN_POINT('Ctrl Pts',(1.92122334398034,-1.,0.172321621259556));
#38195=CARTESIAN_POINT('Ctrl Pts',(1.92122334398034,1.,0.172321621259556));
#38196=CARTESIAN_POINT('Ctrl Pts',(1.92731093582,-1.,0.17147119153296));
#38197=CARTESIAN_POINT('Ctrl Pts',(1.92731093582,1.,0.17147119153296));
#38198=CARTESIAN_POINT('Ctrl Pts',(1.93329183155455,-1.,0.170541253116136));
#38199=CARTESIAN_POINT('Ctrl Pts',(1.93329183155455,1.,0.170541253116136));
#38200=CARTESIAN_POINT('Ctrl Pts',(1.93915639211497,-1.,0.169534904817425));
#38201=CARTESIAN_POINT('Ctrl Pts',(1.93915639211497,1.,0.169534904817425));
#38202=CARTESIAN_POINT('Ctrl Pts',(1.94493757756879,-1.,0.168455741607515));
#38203=CARTESIAN_POINT('Ctrl Pts',(1.94493757756879,1.,0.168455741607515));
#38204=CARTESIAN_POINT('Ctrl Pts',(1.95069027794286,-1.,0.167307501784469));
#38205=CARTESIAN_POINT('Ctrl Pts',(1.95069027794286,1.,0.167307501784469));
#38206=CARTESIAN_POINT('Ctrl Pts',(1.95646759718755,-1.,0.166093592002832));
#38207=CARTESIAN_POINT('Ctrl Pts',(1.95646759718755,1.,0.166093592002832));
#38208=CARTESIAN_POINT('Ctrl Pts',(1.96229379940174,-1.,0.1648165689203));
#38209=CARTESIAN_POINT('Ctrl Pts',(1.96229379940174,1.,0.1648165689203));
#38210=CARTESIAN_POINT('Ctrl Pts',(1.96816512678,-1.,0.16347818545776));
#38211=CARTESIAN_POINT('Ctrl Pts',(1.96816512678,1.,0.16347818545776));
#38212=CARTESIAN_POINT('Ctrl Pts',(1.97406280235204,-1.,0.162079693556302));
#38213=CARTESIAN_POINT('Ctrl Pts',(1.97406280235204,1.,0.162079693556302));
#38214=CARTESIAN_POINT('Ctrl Pts',(1.97996195437557,-1.,0.16062206078461));
#38215=CARTESIAN_POINT('Ctrl Pts',(1.97996195437557,1.,0.16062206078461));
#38216=CARTESIAN_POINT('Ctrl Pts',(1.98584238283279,-1.,0.159106226437288));
#38217=CARTESIAN_POINT('Ctrl Pts',(1.98584238283279,1.,0.159106226437288));
#38218=CARTESIAN_POINT('Ctrl Pts',(1.99169810931893,-1.,0.157533331459215));
#38219=CARTESIAN_POINT('Ctrl Pts',(1.99169810931893,1.,0.157533331459215));
#38220=CARTESIAN_POINT('Ctrl Pts',(1.99753284771487,-1.,0.155904629548774));
#38221=CARTESIAN_POINT('Ctrl Pts',(1.99753284771487,1.,0.155904629548774));
#38222=CARTESIAN_POINT('Ctrl Pts',(2.00335565310539,-1.,0.154221403049719));
#38223=CARTESIAN_POINT('Ctrl Pts',(2.00335565310539,1.,0.154221403049719));
#38224=CARTESIAN_POINT('Ctrl Pts',(2.00917680318426,-1.,0.152484883621452));
#38225=CARTESIAN_POINT('Ctrl Pts',(2.00917680318426,1.,0.152484883621452));
#38226=CARTESIAN_POINT('Ctrl Pts',(2.01500291940243,-1.,0.150696157673084));
#38227=CARTESIAN_POINT('Ctrl Pts',(2.01500291940243,1.,0.150696157673084));
#38228=CARTESIAN_POINT('Ctrl Pts',(2.02083464969897,-1.,0.148856124775342));
#38229=CARTESIAN_POINT('Ctrl Pts',(2.02083464969897,1.,0.148856124775342));
#38230=CARTESIAN_POINT('Ctrl Pts',(2.02666926182017,-1.,0.146965557332586));
#38231=CARTESIAN_POINT('Ctrl Pts',(2.02666926182017,1.,0.146965557332586));
#38232=CARTESIAN_POINT('Ctrl Pts',(2.03250223739941,-1.,0.145025140186058));
#38233=CARTESIAN_POINT('Ctrl Pts',(2.03250223739941,1.,0.145025140186058));
#38234=CARTESIAN_POINT('Ctrl Pts',(2.03832911025913,-1.,0.143035515058208));
#38235=CARTESIAN_POINT('Ctrl Pts',(2.03832911025913,1.,0.143035515058208));
#38236=CARTESIAN_POINT('Ctrl Pts',(2.04414757947919,-1.,0.140997332152545));
#38237=CARTESIAN_POINT('Ctrl Pts',(2.04414757947919,1.,0.140997332152545));
#38238=CARTESIAN_POINT('Ctrl Pts',(2.04995762001333,-1.,0.138911255368966));
#38239=CARTESIAN_POINT('Ctrl Pts',(2.04995762001333,1.,0.138911255368966));
#38240=CARTESIAN_POINT('Ctrl Pts',(2.0557604441427,-1.,0.136777941218044));
#38241=CARTESIAN_POINT('Ctrl Pts',(2.0557604441427,1.,0.136777941218044));
#38242=CARTESIAN_POINT('Ctrl Pts',(2.06155781517844,-1.,0.134598026192107));
#38243=CARTESIAN_POINT('Ctrl Pts',(2.06155781517844,1.,0.134598026192107));
#38244=CARTESIAN_POINT('Ctrl Pts',(2.06735123910319,-1.,0.132372111547709));
#38245=CARTESIAN_POINT('Ctrl Pts',(2.06735123910319,1.,0.132372111547709));
#38246=CARTESIAN_POINT('Ctrl Pts',(2.07314114713047,-1.,0.1301007483284));
#38247=CARTESIAN_POINT('Ctrl Pts',(2.07314114713047,1.,0.1301007483284));
#38248=CARTESIAN_POINT('Ctrl Pts',(2.07892715110967,-1.,0.127784445276116));
#38249=CARTESIAN_POINT('Ctrl Pts',(2.07892715110967,1.,0.127784445276116));
#38250=CARTESIAN_POINT('Ctrl Pts',(2.08470840653628,-1.,0.125423679412058));
#38251=CARTESIAN_POINT('Ctrl Pts',(2.08470840653628,1.,0.125423679412058));
#38252=CARTESIAN_POINT('Ctrl Pts',(2.09048392424826,-1.,0.123018905621083));
#38253=CARTESIAN_POINT('Ctrl Pts',(2.09048392424826,1.,0.123018905621083));
#38254=CARTESIAN_POINT('Ctrl Pts',(2.09625292867756,-1.,0.120570567965129));
#38255=CARTESIAN_POINT('Ctrl Pts',(2.09625292867756,1.,0.120570567965129));
#38256=CARTESIAN_POINT('Ctrl Pts',(2.10201512132945,-1.,0.118079107988368));
#38257=CARTESIAN_POINT('Ctrl Pts',(2.10201512132945,1.,0.118079107988368));
#38258=CARTESIAN_POINT('Ctrl Pts',(2.10777050261359,-1.,0.11554495768794));
#38259=CARTESIAN_POINT('Ctrl Pts',(2.10777050261359,1.,0.11554495768794));
#38260=CARTESIAN_POINT('Ctrl Pts',(2.11351924490335,-1.,0.112968534419746));
#38261=CARTESIAN_POINT('Ctrl Pts',(2.11351924490335,1.,0.112968534419746));
#38262=CARTESIAN_POINT('Ctrl Pts',(2.11926155590849,-1.,0.11035023613502));
#38263=CARTESIAN_POINT('Ctrl Pts',(2.11926155590849,1.,0.11035023613502));
#38264=CARTESIAN_POINT('Ctrl Pts',(2.12499752306927,-1.,0.107690435231068));
#38265=CARTESIAN_POINT('Ctrl Pts',(2.12499752306927,1.,0.107690435231068));
#38266=CARTESIAN_POINT('Ctrl Pts',(2.1307270488718,-1.,0.104989479152703));
#38267=CARTESIAN_POINT('Ctrl Pts',(2.1307270488718,1.,0.104989479152703));
#38268=CARTESIAN_POINT('Ctrl Pts',(2.13644992667052,-1.,0.102247700556063));
#38269=CARTESIAN_POINT('Ctrl Pts',(2.13644992667052,1.,0.102247700556063));
#38270=CARTESIAN_POINT('Ctrl Pts',(2.14216588395974,-1.,0.0994654261990741));
#38271=CARTESIAN_POINT('Ctrl Pts',(2.14216588395974,1.,0.0994654261990741));
#38272=CARTESIAN_POINT('Ctrl Pts',(2.14787463531864,-1.,0.0966429852305688));
#38273=CARTESIAN_POINT('Ctrl Pts',(2.14787463531864,1.,0.0966429852305688));
#38274=CARTESIAN_POINT('Ctrl Pts',(2.15357593978377,-1.,0.0937807218868344));
#38275=CARTESIAN_POINT('Ctrl Pts',(2.15357593978377,1.,0.0937807218868344));
#38276=CARTESIAN_POINT('Ctrl Pts',(2.15926961544808,-1.,0.0908789888108265));
#38277=CARTESIAN_POINT('Ctrl Pts',(2.15926961544808,1.,0.0908789888108265));
#38278=CARTESIAN_POINT('Ctrl Pts',(2.16495552645275,-1.,0.0879381291387821));
#38279=CARTESIAN_POINT('Ctrl Pts',(2.16495552645275,1.,0.0879381291387821));
#38280=CARTESIAN_POINT('Ctrl Pts',(2.17063357871031,-1.,0.0849584620835642));
#38281=CARTESIAN_POINT('Ctrl Pts',(2.17063357871031,1.,0.0849584620835642));
#38282=CARTESIAN_POINT('Ctrl Pts',(2.1763037121106,-1.,0.0819402680871938));
#38283=CARTESIAN_POINT('Ctrl Pts',(2.1763037121106,1.,0.0819402680871938));
#38284=CARTESIAN_POINT('Ctrl Pts',(2.18196589448304,-1.,0.0788837727683226));
#38285=CARTESIAN_POINT('Ctrl Pts',(2.18196589448304,1.,0.0788837727683226));
#38286=CARTESIAN_POINT('Ctrl Pts',(2.1876201139874,-1.,0.075789146583341));
#38287=CARTESIAN_POINT('Ctrl Pts',(2.1876201139874,1.,0.075789146583341));
#38288=CARTESIAN_POINT('Ctrl Pts',(2.19213712012956,-1.,0.0732830357304275));
#38289=CARTESIAN_POINT('Ctrl Pts',(2.19213712012956,1.,0.0732830357304275));
#38290=CARTESIAN_POINT('Ctrl Pts',(2.19552129483562,-1.,0.0713863779524626));
#38291=CARTESIAN_POINT('Ctrl Pts',(2.19552129483562,1.,0.0713863779524626));
#38292=CARTESIAN_POINT('Ctrl Pts',(2.19777582085261,-1.,0.0701143536324925));
#38293=CARTESIAN_POINT('Ctrl Pts',(2.19777582085261,1.,0.0701143536324925));
#38294=CARTESIAN_POINT('Ctrl Pts',(2.19890268624765,-1.,0.0694764450219582));
#38295=CARTESIAN_POINT('Ctrl Pts',(2.19890268624765,1.,0.0694764450219582));
#38296=CARTESIAN_POINT('',(1.74236521665491,1.,0.163289472382896));
#38297=CARTESIAN_POINT('Ctrl Pts',(1.74236521665491,1.,0.163289472382896));
#38298=CARTESIAN_POINT('Ctrl Pts',(1.74720349503904,1.,0.163814161002474));
#38299=CARTESIAN_POINT('Ctrl Pts',(1.75666056640041,1.,0.164834765708484));
#38300=CARTESIAN_POINT('Ctrl Pts',(1.77018771687692,1.,0.166279355148738));
#38301=CARTESIAN_POINT('Ctrl Pts',(1.78690649988931,1.,0.16803277280837));
#38302=CARTESIAN_POINT('Ctrl Pts',(1.80561530633924,1.,0.169936923908078));
#38303=CARTESIAN_POINT('Ctrl Pts',(1.82215766815414,1.,0.171554770207306));
#38304=CARTESIAN_POINT('Ctrl Pts',(1.83658380530747,1.,0.17288944289442));
#38305=CARTESIAN_POINT('Ctrl Pts',(1.84898113200543,1.,0.173946627589401));
#38306=CARTESIAN_POINT('Ctrl Pts',(1.85948367089838,1.,0.174735259276856));
#38307=CARTESIAN_POINT('Ctrl Pts',(1.86828349694972,1.,0.1752683375909));
#38308=CARTESIAN_POINT('Ctrl Pts',(1.87563767773249,1.,0.175563480746205));
#38309=CARTESIAN_POINT('Ctrl Pts',(1.88188663144846,1.,0.175644148889271));
#38310=CARTESIAN_POINT('Ctrl Pts',(1.88742606272818,1.,0.175538155840286));
#38311=CARTESIAN_POINT('Ctrl Pts',(1.89264630198279,1.,0.175274276190664));
#38312=CARTESIAN_POINT('Ctrl Pts',(1.89788101117148,1.,0.174879405091277));
#38313=CARTESIAN_POINT('Ctrl Pts',(1.90335253863003,1.,0.174375518661222));
#38314=CARTESIAN_POINT('Ctrl Pts',(1.90911693975475,1.,0.173776635257983));
#38315=CARTESIAN_POINT('Ctrl Pts',(1.91511429159681,1.,0.173090695383619));
#38316=CARTESIAN_POINT('Ctrl Pts',(1.92122334398034,1.,0.172321621259556));
#38317=CARTESIAN_POINT('Ctrl Pts',(1.92731093582,1.,0.17147119153296));
#38318=CARTESIAN_POINT('Ctrl Pts',(1.93329183155455,1.,0.170541253116136));
#38319=CARTESIAN_POINT('Ctrl Pts',(1.93915639211497,1.,0.169534904817425));
#38320=CARTESIAN_POINT('Ctrl Pts',(1.94493757756879,1.,0.168455741607515));
#38321=CARTESIAN_POINT('Ctrl Pts',(1.95069027794286,1.,0.167307501784469));
#38322=CARTESIAN_POINT('Ctrl Pts',(1.95646759718755,1.,0.166093592002832));
#38323=CARTESIAN_POINT('Ctrl Pts',(1.96229379940174,1.,0.1648165689203));
#38324=CARTESIAN_POINT('Ctrl Pts',(1.96816512678,1.,0.16347818545776));
#38325=CARTESIAN_POINT('Ctrl Pts',(1.97406280235204,1.,0.162079693556302));
#38326=CARTESIAN_POINT('Ctrl Pts',(1.97996195437557,1.,0.16062206078461));
#38327=CARTESIAN_POINT('Ctrl Pts',(1.98584238283279,1.,0.159106226437288));
#38328=CARTESIAN_POINT('Ctrl Pts',(1.99169810931893,1.,0.157533331459215));
#38329=CARTESIAN_POINT('Ctrl Pts',(1.99753284771487,1.,0.155904629548774));
#38330=CARTESIAN_POINT('Ctrl Pts',(2.00335565310539,1.,0.154221403049719));
#38331=CARTESIAN_POINT('Ctrl Pts',(2.00917680318426,1.,0.152484883621452));
#38332=CARTESIAN_POINT('Ctrl Pts',(2.01500291940243,1.,0.150696157673084));
#38333=CARTESIAN_POINT('Ctrl Pts',(2.02083464969897,1.,0.148856124775342));
#38334=CARTESIAN_POINT('Ctrl Pts',(2.02666926182017,1.,0.146965557332586));
#38335=CARTESIAN_POINT('Ctrl Pts',(2.03250223739941,1.,0.145025140186058));
#38336=CARTESIAN_POINT('Ctrl Pts',(2.03832911025913,1.,0.143035515058208));
#38337=CARTESIAN_POINT('Ctrl Pts',(2.04414757947919,1.,0.140997332152545));
#38338=CARTESIAN_POINT('Ctrl Pts',(2.04995762001333,1.,0.138911255368966));
#38339=CARTESIAN_POINT('Ctrl Pts',(2.0557604441427,1.,0.136777941218044));
#38340=CARTESIAN_POINT('Ctrl Pts',(2.06155781517844,1.,0.134598026192107));
#38341=CARTESIAN_POINT('Ctrl Pts',(2.06735123910319,1.,0.132372111547709));
#38342=CARTESIAN_POINT('Ctrl Pts',(2.07314114713047,1.,0.1301007483284));
#38343=CARTESIAN_POINT('Ctrl Pts',(2.07892715110967,1.,0.127784445276116));
#38344=CARTESIAN_POINT('Ctrl Pts',(2.08470840653628,1.,0.125423679412058));
#38345=CARTESIAN_POINT('Ctrl Pts',(2.09048392424826,1.,0.123018905621083));
#38346=CARTESIAN_POINT('Ctrl Pts',(2.09625292867756,1.,0.120570567965129));
#38347=CARTESIAN_POINT('Ctrl Pts',(2.10201512132945,1.,0.118079107988368));
#38348=CARTESIAN_POINT('Ctrl Pts',(2.10777050261359,1.,0.11554495768794));
#38349=CARTESIAN_POINT('Ctrl Pts',(2.11351924490335,1.,0.112968534419746));
#38350=CARTESIAN_POINT('Ctrl Pts',(2.11926155590849,1.,0.11035023613502));
#38351=CARTESIAN_POINT('Ctrl Pts',(2.12499752306927,1.,0.107690435231068));
#38352=CARTESIAN_POINT('Ctrl Pts',(2.1307270488718,1.,0.104989479152703));
#38353=CARTESIAN_POINT('Ctrl Pts',(2.13644992667052,1.,0.102247700556063));
#38354=CARTESIAN_POINT('Ctrl Pts',(2.14216588395974,1.,0.0994654261990741));
#38355=CARTESIAN_POINT('Ctrl Pts',(2.14787463531864,1.,0.0966429852305688));
#38356=CARTESIAN_POINT('Ctrl Pts',(2.15357593978377,1.,0.0937807218868344));
#38357=CARTESIAN_POINT('Ctrl Pts',(2.15926961544808,1.,0.0908789888108265));
#38358=CARTESIAN_POINT('Ctrl Pts',(2.16495552645275,1.,0.0879381291387821));
#38359=CARTESIAN_POINT('Ctrl Pts',(2.17063357871031,1.,0.0849584620835642));
#38360=CARTESIAN_POINT('Ctrl Pts',(2.1763037121106,1.,0.0819402680871938));
#38361=CARTESIAN_POINT('Ctrl Pts',(2.18196589448304,1.,0.0788837727683226));
#38362=CARTESIAN_POINT('Ctrl Pts',(2.1876201139874,1.,0.075789146583341));
#38363=CARTESIAN_POINT('Ctrl Pts',(2.19213712012956,1.,0.0732830357304275));
#38364=CARTESIAN_POINT('Ctrl Pts',(2.19552129483562,1.,0.0713863779524626));
#38365=CARTESIAN_POINT('Ctrl Pts',(2.19777582085261,1.,0.0701143536324925));
#38366=CARTESIAN_POINT('Ctrl Pts',(2.19890268624765,1.,0.0694764450219582));
#38367=CARTESIAN_POINT('',(1.74236521665491,0.,0.163289472382896));
#38368=CARTESIAN_POINT('Origin',(0.,1.,0.));
#38369=CARTESIAN_POINT('Origin',(0.,1.,0.));
#38370=CARTESIAN_POINT('Origin',(0.,0.,0.));
#62667=UNCERTAINTY_MEASURE_WITH_UNIT(LENGTH_MEASURE(0.001),#62759,
'DISTANCE_ACCURACY_VALUE',
'Maximum model space distance between geometric entities at asserted c
onnectivities');
#62684=UNCERTAINTY_MEASURE_WITH_UNIT(LENGTH_MEASURE(0.001),#62759,
'DISTANCE_ACCURACY_VALUE',
'Maximum model space distance between geometric entities at asserted c
onnectivities');
#62741=(
GEOMETRIC_REPRESENTATION_CONTEXT(3)
GLOBAL_UNCERTAINTY_ASSIGNED_CONTEXT((#62667))
GLOBAL_UNIT_ASSIGNED_CONTEXT((#62759,#62761,#62762))
REPRESENTATION_CONTEXT('','3D')
);
#62758=(
GEOMETRIC_REPRESENTATION_CONTEXT(3)
GLOBAL_UNCERTAINTY_ASSIGNED_CONTEXT((#62684))
GLOBAL_UNIT_ASSIGNED_CONTEXT((#62759,#62761,#62762))
REPRESENTATION_CONTEXT('','3D')
);
#62759=(
LENGTH_UNIT()
NAMED_UNIT(*)
SI_UNIT(.CENTI.,.METRE.)
);
#62761=(
NAMED_UNIT(*)
PLANE_ANGLE_UNIT()
SI_UNIT($,.RADIAN.)
);
#62762=(
NAMED_UNIT(*)
SI_UNIT($,.STERADIAN.)
SOLID_ANGLE_UNIT()
);
#62819=SHAPE_DEFINITION_REPRESENTATION(#62902,#63087);
#62902=PRODUCT_DEFINITION_SHAPE('',$,#63161);
#63087=SHAPE_REPRESENTATION('',(#18271),#62741);
#63104=PRODUCT_DEFINITION_CONTEXT('part definition',#63325,'design');
#63161=PRODUCT_DEFINITION('Spur Gear - Module 2, 20 Teeth, 12 mm Bore',
'Spur Gear - Module 2, 20 Teeth, 12 mm Bore',#63234,#63104);
#63234=PRODUCT_DEFINITION_FORMATION('',$,#63383);
#63325=APPLICATION_CONTEXT(
'Core Data for Automotive Mechanical Design Process');
#63326=PRODUCT_CONTEXT('part definition',#63325,'mechanical');
#63383=PRODUCT('Spur Gear - Module 2, 20 Teeth, 12 mm Bore',
'Spur Gear - Module 2, 20 Teeth, 12 mm Bore',
'Spur Gear - Module 2, 20 Teeth, 12 mm Bore',(#63326));
#63470=COLOUR_RGB('Off White',0.89,0.88,0.83);
#63471=FILL_AREA_STYLE_COLOUR('',#63470);
#63472=FILL_AREA_STYLE('',(#63471));
#63473=SURFACE_STYLE_FILL_AREA(#63472);
#63474=SURFACE_SIDE_STYLE('',(#63473));
#63475=SURFACE_STYLE_USAGE(.BOTH.,#63474);
#63476=PRESENTATION_STYLE_ASSIGNMENT((#63475));
ENDSEC;
END-ISO-10303-21;
